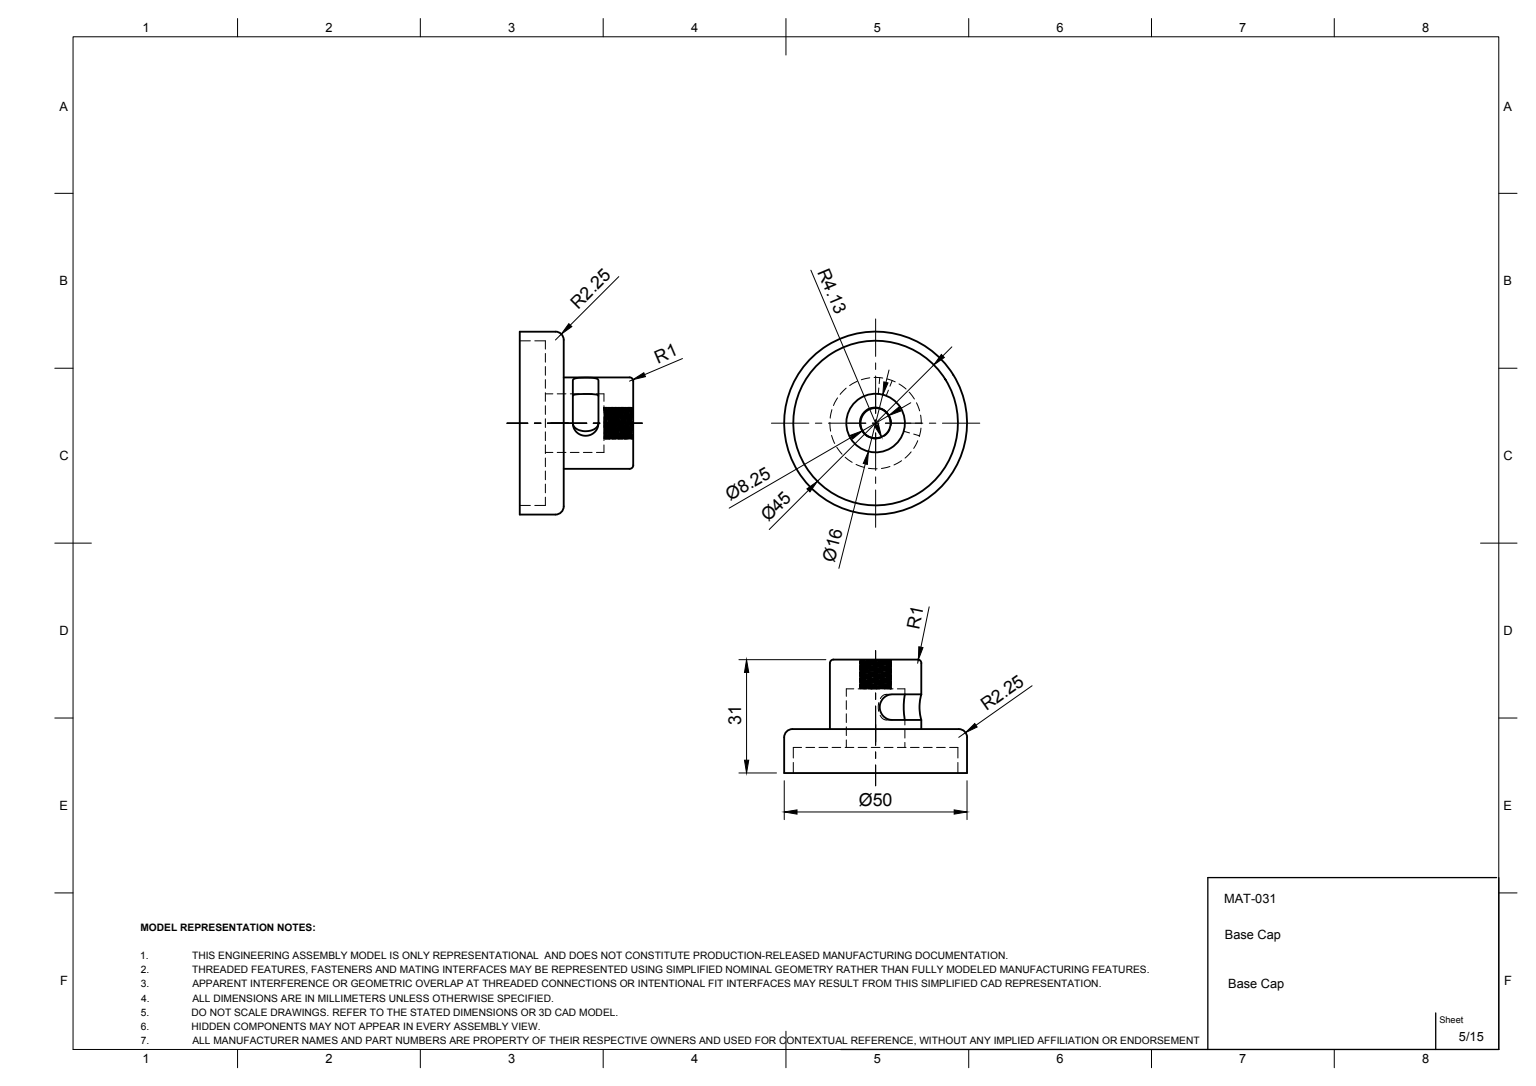
ISO-10303-21;
HEADER;
/* Generated by software containing ST-Developer
 * from STEP Tools, Inc. (www.steptools.com) 
 */

FILE_DESCRIPTION(
/* description */ ('STEP AP214'),
/* implementation_level */ '2;1');

FILE_NAME(
/* name */ 'Base Cap.step',
/* time_stamp */ '2026-11-14T06:58:01-08:00',
/* author */ (''),
/* organization */ (''),
/* preprocessor_version */ 'ST-DEVELOPER v20.2',
/* originating_system */ 'Autodesk Translation Framework v15.17.0.0',
/* authorisation */ '');

FILE_SCHEMA (('AUTOMOTIVE_DESIGN { 1 0 10303 214 3 1 1 }'));
ENDSEC;

DATA;
#10=MECHANICAL_DESIGN_GEOMETRIC_PRESENTATION_REPRESENTATION('',(#1148),#38635);
#124=(
BOUNDED_SURFACE()
B_SPLINE_SURFACE(1,2,((#28370,#28371,#28372,#28373,#28374,#28375,#28376,
#28377,#28378,#28379,#28380,#28381,#28382,#28383,#28384,#28385,#28386,#28387,
#28388,#28389,#28390,#28391,#28392,#28393,#28394,#28395,#28396,#28397,#28398,
#28399,#28400,#28401,#28402,#28403,#28404,#28405,#28406,#28407,#28408,#28409,
#28410,#28411,#28412,#28413,#28414,#28415,#28416,#28417,#28418,#28419,#28420,
#28421,#28422,#28423,#28424,#28425,#28426,#28427,#28428,#28429,#28430,#28431,
#28432,#28433,#28434,#28435,#28436,#28437,#28438,#28439,#28440,#28441,#28442,
#28443,#28444,#28445,#28446,#28447,#28448,#28449,#28450,#28451,#28452,#28453,
#28454,#28455,#28456,#28457,#28458,#28459,#28460,#28461,#28462,#28463,#28464,
#28465,#28466,#28467,#28468,#28469,#28470,#28471,#28472,#28473,#28474,#28475,
#28476,#28477,#28478,#28479,#28480,#28481,#28482,#28483,#28484,#28485,#28486,
#28487,#28488,#28489,#28490,#28491,#28492,#28493,#28494,#28495,#28496,#28497,
#28498,#28499,#28500,#28501,#28502,#28503,#28504,#28505,#28506,#28507,#28508,
#28509,#28510,#28511,#28512,#28513,#28514,#28515,#28516,#28517,#28518,#28519,
#28520,#28521,#28522,#28523,#28524,#28525,#28526,#28527,#28528,#28529,#28530,
#28531,#28532,#28533,#28534,#28535,#28536,#28537,#28538,#28539,#28540,#28541,
#28542,#28543,#28544,#28545,#28546,#28547,#28548,#28549,#28550,#28551,#28552,
#28553,#28554,#28555,#28556,#28557,#28558,#28559,#28560,#28561,#28562,#28563,
#28564,#28565,#28566,#28567,#28568,#28569,#28570,#28571,#28572,#28573,#28574,
#28575,#28576,#28577,#28578,#28579,#28580,#28581,#28582,#28583,#28584,#28585,
#28586,#28587,#28588,#28589,#28590,#28591,#28592,#28593,#28594,#28595,#28596,
#28597,#28598,#28599,#28600,#28601,#28602,#28603,#28604,#28605,#28606,#28607,
#28608,#28609,#28610,#28611,#28612,#28613,#28614,#28615,#28616,#28617,#28618,
#28619,#28620,#28621,#28622,#28623,#28624,#28625,#28626,#28627,#28628,#28629,
#28630,#28631,#28632,#28633,#28634,#28635,#28636,#28637,#28638,#28639,#28640,
#28641,#28642,#28643,#28644,#28645,#28646,#28647,#28648,#28649,#28650,#28651,
#28652,#28653,#28654,#28655,#28656,#28657,#28658,#28659,#28660,#28661,#28662,
#28663,#28664,#28665,#28666,#28667,#28668,#28669,#28670,#28671,#28672,#28673,
#28674,#28675,#28676,#28677,#28678,#28679,#28680,#28681,#28682,#28683,#28684,
#28685,#28686,#28687,#28688,#28689,#28690,#28691,#28692,#28693,#28694,#28695,
#28696,#28697,#28698,#28699,#28700,#28701,#28702,#28703,#28704,#28705,#28706,
#28707,#28708,#28709,#28710,#28711,#28712,#28713,#28714,#28715,#28716,#28717,
#28718,#28719,#28720,#28721,#28722,#28723,#28724,#28725,#28726,#28727,#28728,
#28729,#28730,#28731,#28732,#28733,#28734,#28735,#28736,#28737,#28738,#28739,
#28740,#28741,#28742,#28743,#28744,#28745,#28746,#28747,#28748),(#28749,
#28750,#28751,#28752,#28753,#28754,#28755,#28756,#28757,#28758,#28759,#28760,
#28761,#28762,#28763,#28764,#28765,#28766,#28767,#28768,#28769,#28770,#28771,
#28772,#28773,#28774,#28775,#28776,#28777,#28778,#28779,#28780,#28781,#28782,
#28783,#28784,#28785,#28786,#28787,#28788,#28789,#28790,#28791,#28792,#28793,
#28794,#28795,#28796,#28797,#28798,#28799,#28800,#28801,#28802,#28803,#28804,
#28805,#28806,#28807,#28808,#28809,#28810,#28811,#28812,#28813,#28814,#28815,
#28816,#28817,#28818,#28819,#28820,#28821,#28822,#28823,#28824,#28825,#28826,
#28827,#28828,#28829,#28830,#28831,#28832,#28833,#28834,#28835,#28836,#28837,
#28838,#28839,#28840,#28841,#28842,#28843,#28844,#28845,#28846,#28847,#28848,
#28849,#28850,#28851,#28852,#28853,#28854,#28855,#28856,#28857,#28858,#28859,
#28860,#28861,#28862,#28863,#28864,#28865,#28866,#28867,#28868,#28869,#28870,
#28871,#28872,#28873,#28874,#28875,#28876,#28877,#28878,#28879,#28880,#28881,
#28882,#28883,#28884,#28885,#28886,#28887,#28888,#28889,#28890,#28891,#28892,
#28893,#28894,#28895,#28896,#28897,#28898,#28899,#28900,#28901,#28902,#28903,
#28904,#28905,#28906,#28907,#28908,#28909,#28910,#28911,#28912,#28913,#28914,
#28915,#28916,#28917,#28918,#28919,#28920,#28921,#28922,#28923,#28924,#28925,
#28926,#28927,#28928,#28929,#28930,#28931,#28932,#28933,#28934,#28935,#28936,
#28937,#28938,#28939,#28940,#28941,#28942,#28943,#28944,#28945,#28946,#28947,
#28948,#28949,#28950,#28951,#28952,#28953,#28954,#28955,#28956,#28957,#28958,
#28959,#28960,#28961,#28962,#28963,#28964,#28965,#28966,#28967,#28968,#28969,
#28970,#28971,#28972,#28973,#28974,#28975,#28976,#28977,#28978,#28979,#28980,
#28981,#28982,#28983,#28984,#28985,#28986,#28987,#28988,#28989,#28990,#28991,
#28992,#28993,#28994,#28995,#28996,#28997,#28998,#28999,#29000,#29001,#29002,
#29003,#29004,#29005,#29006,#29007,#29008,#29009,#29010,#29011,#29012,#29013,
#29014,#29015,#29016,#29017,#29018,#29019,#29020,#29021,#29022,#29023,#29024,
#29025,#29026,#29027,#29028,#29029,#29030,#29031,#29032,#29033,#29034,#29035,
#29036,#29037,#29038,#29039,#29040,#29041,#29042,#29043,#29044,#29045,#29046,
#29047,#29048,#29049,#29050,#29051,#29052,#29053,#29054,#29055,#29056,#29057,
#29058,#29059,#29060,#29061,#29062,#29063,#29064,#29065,#29066,#29067,#29068,
#29069,#29070,#29071,#29072,#29073,#29074,#29075,#29076,#29077,#29078,#29079,
#29080,#29081,#29082,#29083,#29084,#29085,#29086,#29087,#29088,#29089,#29090,
#29091,#29092,#29093,#29094,#29095,#29096,#29097,#29098,#29099,#29100,#29101,
#29102,#29103,#29104,#29105,#29106,#29107,#29108,#29109,#29110,#29111,#29112,
#29113,#29114,#29115,#29116,#29117,#29118,#29119,#29120,#29121,#29122,#29123,
#29124,#29125,#29126,#29127)),.UNSPECIFIED.,.F.,.F.,.F.)
B_SPLINE_SURFACE_WITH_KNOTS((2,2),(3,2,2,2,2,2,2,2,2,2,2,2,2,2,2,2,2,2,
2,2,2,2,2,2,2,2,2,2,2,2,2,2,2,2,2,2,2,2,2,2,2,2,2,2,2,2,2,2,2,2,2,2,2,2,
2,2,2,2,2,2,2,2,2,2,2,2,2,2,2,2,2,2,2,2,2,2,2,2,2,2,2,2,2,2,2,2,2,2,2,2,
2,2,2,2,2,2,2,2,2,2,2,2,2,2,2,2,2,2,2,2,2,2,2,2,2,2,2,2,2,2,2,2,2,2,2,2,
2,2,2,2,2,2,2,2,2,2,2,2,2,2,2,2,2,2,2,2,2,2,2,2,2,2,2,2,2,2,2,2,2,2,2,2,
2,2,2,2,2,2,2,2,2,2,2,2,2,2,2,2,2,2,2,2,2,2,2,2,2,2,2,3),(0.,1.),(0.,0.00520833333333333,
0.0104166666666667,0.015625,0.0208333333333333,0.0260416666666667,0.03125,
0.0364583333333333,0.0416666666666667,0.046875,0.0520833333333333,0.0572916666666667,
0.0625,0.0677083333333333,0.0729166666666667,0.078125,0.0833333333333333,
0.0885416666666667,0.09375,0.0989583333333333,0.104166666666667,0.109375,
0.114583333333333,0.119791666666667,0.125,0.130208333333333,0.135416666666667,
0.140625,0.145833333333333,0.151041666666667,0.15625,0.161458333333333,
0.166666666666667,0.171875,0.177083333333333,0.182291666666667,0.1875,0.192708333333333,
0.197916666666667,0.203125,0.208333333333333,0.213541666666667,0.21875,
0.223958333333333,0.229166666666667,0.234375,0.239583333333333,0.244791666666667,
0.25,0.255208333333333,0.260416666666667,0.265625,0.270833333333333,0.276041666666667,
0.28125,0.286458333333333,0.291666666666667,0.296875,0.302083333333333,
0.307291666666667,0.3125,0.317708333333333,0.322916666666667,0.328125,0.333333333333333,
0.338541666666667,0.34375,0.348958333333333,0.354166666666667,0.359375,
0.364583333333333,0.369791666666667,0.375,0.380208333333333,0.385416666666667,
0.390625,0.395833333333333,0.401041666666667,0.40625,0.411458333333333,
0.416666666666667,0.421875,0.427083333333333,0.432291666666667,0.4375,0.442708333333333,
0.447916666666667,0.453125,0.458333333333333,0.463541666666667,0.46875,
0.473958333333333,0.479166666666667,0.484375,0.489583333333333,0.494791666666667,
0.5,0.505208333333333,0.510416666666667,0.515625,0.520833333333333,0.526041666666667,
0.53125,0.536458333333333,0.541666666666667,0.546875,0.552083333333333,
0.557291666666667,0.5625,0.567708333333333,0.572916666666667,0.578125,0.583333333333333,
0.588541666666667,0.59375,0.598958333333333,0.604166666666667,0.609375,
0.614583333333333,0.619791666666667,0.625,0.630208333333333,0.635416666666667,
0.640625,0.645833333333333,0.651041666666667,0.65625,0.661458333333333,
0.666666666666667,0.671875,0.677083333333333,0.682291666666667,0.6875,0.692708333333333,
0.697916666666667,0.703125,0.708333333333333,0.713541666666667,0.71875,
0.723958333333333,0.729166666666667,0.734375,0.739583333333333,0.744791666666667,
0.75,0.755208333333333,0.760416666666667,0.765625,0.770833333333333,0.776041666666667,
0.78125,0.786458333333333,0.791666666666667,0.796875,0.802083333333333,
0.807291666666667,0.8125,0.817708333333333,0.822916666666667,0.828125,0.833333333333333,
0.838541666666667,0.84375,0.848958333333333,0.854166666666667,0.859375,
0.864583333333333,0.869791666666667,0.875,0.880208333333333,0.885416666666667,
0.890625,0.895833333333333,0.901041666666667,0.90625,0.911458333333333,
0.916666666666667,0.921875,0.927083333333333,0.932291666666667,0.9375,0.942708333333333,
0.947916666666667,0.953125,0.958333333333333,0.963541666666667,0.96875,
0.973958333333333,0.979166666666667,0.984246579235552),.UNSPECIFIED.)
GEOMETRIC_REPRESENTATION_ITEM()
RATIONAL_B_SPLINE_SURFACE(((1.,0.866025403784439,1.,0.866025403784439,1.,
0.866025403784439,1.,0.866025403784439,1.,0.866025403784439,1.,0.866025403784439,
1.,0.866025403784439,1.,0.866025403784439,1.,0.866025403784439,1.,0.866025403784439,
1.,0.866025403784439,1.,0.866025403784439,1.,0.866025403784439,1.,0.866025403784439,
1.,0.866025403784439,1.,0.866025403784439,1.,0.866025403784439,1.,0.866025403784439,
1.,0.866025403784439,1.,0.866025403784439,1.,0.866025403784439,1.,0.866025403784439,
1.,0.866025403784439,1.,0.866025403784439,1.,0.866025403784439,1.,0.866025403784439,
1.,0.866025403784439,1.,0.866025403784439,1.,0.866025403784439,1.,0.866025403784439,
1.,0.866025403784439,1.,0.866025403784439,1.,0.866025403784439,1.,0.866025403784439,
1.,0.866025403784439,1.,0.866025403784439,1.,0.866025403784439,1.,0.866025403784439,
1.,0.866025403784439,1.,0.866025403784439,1.,0.866025403784439,1.,0.866025403784439,
1.,0.866025403784439,1.,0.866025403784439,1.,0.866025403784439,1.,0.866025403784439,
1.,0.866025403784439,1.,0.866025403784439,1.,0.866025403784439,1.,0.866025403784439,
1.,0.866025403784439,1.,0.866025403784439,1.,0.866025403784439,1.,0.866025403784439,
1.,0.866025403784439,1.,0.866025403784439,1.,0.866025403784439,1.,0.866025403784439,
1.,0.866025403784439,1.,0.866025403784439,1.,0.866025403784439,1.,0.866025403784439,
1.,0.866025403784439,1.,0.866025403784439,1.,0.866025403784439,1.,0.866025403784439,
1.,0.866025403784439,1.,0.866025403784439,1.,0.866025403784439,1.,0.866025403784439,
1.,0.866025403784439,1.,0.866025403784439,1.,0.866025403784439,1.,0.866025403784439,
1.,0.866025403784439,1.,0.866025403784439,1.,0.866025403784439,1.,0.866025403784439,
1.,0.866025403784439,1.,0.866025403784439,1.,0.866025403784439,1.,0.866025403784439,
1.,0.866025403784439,1.,0.866025403784439,1.,0.866025403784439,1.,0.866025403784439,
1.,0.866025403784439,1.,0.866025403784439,1.,0.866025403784439,1.,0.866025403784439,
1.,0.866025403784439,1.,0.866025403784439,1.,0.866025403784439,1.,0.866025403784439,
1.,0.866025403784439,1.,0.866025403784439,1.,0.866025403784439,1.,0.866025403784439,
1.,0.866025403784439,1.,0.866025403784439,1.,0.866025403784439,1.,0.866025403784439,
1.,0.866025403784439,1.,0.866025403784439,1.,0.866025403784439,1.,0.866025403784439,
1.,0.866025403784439,1.,0.866025403784439,1.,0.866025403784439,1.,0.866025403784439,
1.,0.866025403784439,1.,0.866025403784439,1.,0.866025403784439,1.,0.866025403784439,
1.,0.866025403784439,1.,0.866025403784439,1.,0.866025403784439,1.,0.866025403784439,
1.,0.866025403784439,1.,0.866025403784439,1.,0.866025403784439,1.,0.866025403784439,
1.,0.866025403784439,1.,0.866025403784439,1.,0.866025403784439,1.,0.866025403784439,
1.,0.866025403784439,1.,0.866025403784439,1.,0.866025403784439,1.,0.866025403784439,
1.,0.866025403784439,1.,0.866025403784439,1.,0.866025403784439,1.,0.866025403784439,
1.,0.866025403784439,1.,0.866025403784439,1.,0.866025403784439,1.,0.866025403784439,
1.,0.866025403784439,1.,0.866025403784439,1.,0.866025403784439,1.,0.866025403784439,
1.,0.866025403784439,1.,0.866025403784439,1.,0.866025403784439,1.,0.866025403784439,
1.,0.866025403784439,1.,0.866025403784439,1.,0.866025403784439,1.,0.866025403784439,
1.,0.866025403784439,1.,0.866025403784439,1.,0.866025403784439,1.,0.866025403784439,
1.,0.866025403784439,1.,0.866025403784439,1.,0.866025403784439,1.,0.866025403784439,
1.,0.866025403784439,1.,0.866025403784439,1.,0.866025403784439,1.,0.866025403784439,
1.,0.866025403784439,1.,0.866025403784439,1.,0.866025403784439,1.,0.866025403784439,
1.,0.866025403784439,1.,0.866025403784439,1.,0.866025403784439,1.,0.866025403784439,
1.,0.866025403784439,1.,0.866025403784439,1.,0.866025403784439,1.,0.866025403784439,
1.,0.866025403784439,1.,0.866025403784439,1.,0.866025403784439,1.,0.866025403784439,
1.,0.866025403784439,1.,0.866025403784439,1.,0.866025403784439,1.,0.866025403784439,
1.,0.866025403784439,1.,0.866025403784439,1.,0.866025403784439,1.,0.866025403784439,
1.,0.866025403784439,1.,0.866025403784439,1.,0.869328786836457,0.993556135519056),
(1.,0.866025403784439,1.,0.866025403784439,1.,0.866025403784439,1.,0.866025403784439,
1.,0.866025403784439,1.,0.866025403784439,1.,0.866025403784439,1.,0.866025403784439,
1.,0.866025403784439,1.,0.866025403784439,1.,0.866025403784439,1.,0.866025403784439,
1.,0.866025403784439,1.,0.866025403784439,1.,0.866025403784439,1.,0.866025403784439,
1.,0.866025403784439,1.,0.866025403784439,1.,0.866025403784439,1.,0.866025403784439,
1.,0.866025403784439,1.,0.866025403784439,1.,0.866025403784439,1.,0.866025403784439,
1.,0.866025403784439,1.,0.866025403784439,1.,0.866025403784439,1.,0.866025403784439,
1.,0.866025403784439,1.,0.866025403784439,1.,0.866025403784439,1.,0.866025403784439,
1.,0.866025403784439,1.,0.866025403784439,1.,0.866025403784439,1.,0.866025403784439,
1.,0.866025403784439,1.,0.866025403784439,1.,0.866025403784439,1.,0.866025403784439,
1.,0.866025403784439,1.,0.866025403784439,1.,0.866025403784439,1.,0.866025403784439,
1.,0.866025403784439,1.,0.866025403784439,1.,0.866025403784439,1.,0.866025403784439,
1.,0.866025403784439,1.,0.866025403784439,1.,0.866025403784439,1.,0.866025403784439,
1.,0.866025403784439,1.,0.866025403784439,1.,0.866025403784439,1.,0.866025403784439,
1.,0.866025403784439,1.,0.866025403784439,1.,0.866025403784439,1.,0.866025403784439,
1.,0.866025403784439,1.,0.866025403784439,1.,0.866025403784439,1.,0.866025403784439,
1.,0.866025403784439,1.,0.866025403784439,1.,0.866025403784439,1.,0.866025403784439,
1.,0.866025403784439,1.,0.866025403784439,1.,0.866025403784439,1.,0.866025403784439,
1.,0.866025403784439,1.,0.866025403784439,1.,0.866025403784439,1.,0.866025403784439,
1.,0.866025403784439,1.,0.866025403784439,1.,0.866025403784439,1.,0.866025403784439,
1.,0.866025403784439,1.,0.866025403784439,1.,0.866025403784439,1.,0.866025403784439,
1.,0.866025403784439,1.,0.866025403784439,1.,0.866025403784439,1.,0.866025403784439,
1.,0.866025403784439,1.,0.866025403784439,1.,0.866025403784439,1.,0.866025403784439,
1.,0.866025403784439,1.,0.866025403784439,1.,0.866025403784439,1.,0.866025403784439,
1.,0.866025403784439,1.,0.866025403784439,1.,0.866025403784439,1.,0.866025403784439,
1.,0.866025403784439,1.,0.866025403784439,1.,0.866025403784439,1.,0.866025403784439,
1.,0.866025403784439,1.,0.866025403784439,1.,0.866025403784439,1.,0.866025403784439,
1.,0.866025403784439,1.,0.866025403784439,1.,0.866025403784439,1.,0.866025403784439,
1.,0.866025403784439,1.,0.866025403784439,1.,0.866025403784439,1.,0.866025403784439,
1.,0.866025403784439,1.,0.866025403784439,1.,0.866025403784439,1.,0.866025403784439,
1.,0.866025403784439,1.,0.866025403784439,1.,0.866025403784439,1.,0.866025403784439,
1.,0.866025403784439,1.,0.866025403784439,1.,0.866025403784439,1.,0.866025403784439,
1.,0.866025403784439,1.,0.866025403784439,1.,0.866025403784439,1.,0.866025403784439,
1.,0.866025403784439,1.,0.866025403784439,1.,0.866025403784439,1.,0.866025403784439,
1.,0.866025403784439,1.,0.866025403784439,1.,0.866025403784439,1.,0.866025403784439,
1.,0.866025403784439,1.,0.866025403784439,1.,0.866025403784439,1.,0.866025403784439,
1.,0.866025403784439,1.,0.866025403784439,1.,0.866025403784439,1.,0.866025403784439,
1.,0.866025403784439,1.,0.866025403784439,1.,0.866025403784439,1.,0.866025403784439,
1.,0.866025403784439,1.,0.866025403784439,1.,0.866025403784439,1.,0.866025403784439,
1.,0.866025403784439,1.,0.866025403784439,1.,0.866025403784439,1.,0.866025403784439,
1.,0.866025403784439,1.,0.866025403784439,1.,0.866025403784439,1.,0.866025403784439,
1.,0.866025403784439,1.,0.866025403784439,1.,0.866025403784439,1.,0.866025403784439,
1.,0.866025403784439,1.,0.866025403784439,1.,0.866025403784439,1.,0.866025403784439,
1.,0.866025403784439,1.,0.866025403784439,1.,0.866025403784439,1.,0.866025403784439,
1.,0.866025403784439,1.,0.866025403784439,1.,0.866025403784439,1.,0.866025403784439,
1.,0.866025403784439,1.,0.866025403784439,1.,0.866025403784439,1.,0.866025403784439,
1.,0.866025403784439,1.,0.866025403784439,1.,0.866025403784439,1.,0.866025403784439,
1.,0.869328786836457,0.993556135519056)))
REPRESENTATION_ITEM('')
SURFACE()
);
#125=(
BOUNDED_SURFACE()
B_SPLINE_SURFACE(1,2,((#29128,#29129,#29130,#29131,#29132,#29133,#29134,
#29135,#29136,#29137,#29138,#29139,#29140,#29141,#29142,#29143,#29144,#29145,
#29146,#29147,#29148,#29149,#29150,#29151,#29152,#29153,#29154,#29155,#29156,
#29157,#29158,#29159,#29160,#29161,#29162,#29163,#29164,#29165,#29166,#29167,
#29168,#29169,#29170,#29171,#29172,#29173,#29174,#29175,#29176,#29177,#29178,
#29179,#29180,#29181,#29182,#29183,#29184,#29185,#29186,#29187,#29188,#29189,
#29190,#29191,#29192,#29193,#29194,#29195,#29196,#29197,#29198,#29199,#29200,
#29201,#29202,#29203,#29204,#29205,#29206,#29207,#29208,#29209,#29210,#29211,
#29212,#29213,#29214,#29215,#29216,#29217,#29218,#29219,#29220,#29221,#29222,
#29223,#29224,#29225,#29226,#29227,#29228,#29229,#29230,#29231,#29232,#29233,
#29234,#29235,#29236,#29237,#29238,#29239,#29240,#29241,#29242,#29243,#29244,
#29245,#29246,#29247,#29248,#29249,#29250,#29251,#29252,#29253,#29254,#29255,
#29256,#29257,#29258,#29259,#29260,#29261,#29262,#29263,#29264,#29265,#29266,
#29267,#29268,#29269,#29270,#29271,#29272,#29273,#29274,#29275,#29276,#29277,
#29278,#29279,#29280,#29281,#29282,#29283,#29284,#29285,#29286,#29287,#29288,
#29289,#29290,#29291,#29292,#29293,#29294,#29295,#29296,#29297,#29298,#29299,
#29300,#29301,#29302,#29303,#29304,#29305,#29306,#29307,#29308,#29309,#29310,
#29311,#29312,#29313,#29314,#29315,#29316,#29317,#29318,#29319,#29320,#29321,
#29322,#29323,#29324,#29325,#29326,#29327,#29328,#29329,#29330,#29331,#29332,
#29333,#29334,#29335,#29336,#29337,#29338,#29339,#29340,#29341,#29342,#29343,
#29344,#29345,#29346,#29347,#29348,#29349,#29350,#29351,#29352,#29353,#29354,
#29355,#29356,#29357,#29358,#29359,#29360,#29361,#29362,#29363,#29364,#29365,
#29366,#29367,#29368,#29369,#29370,#29371,#29372,#29373,#29374,#29375,#29376,
#29377,#29378,#29379,#29380,#29381,#29382,#29383,#29384,#29385,#29386,#29387,
#29388,#29389,#29390,#29391,#29392,#29393,#29394,#29395,#29396,#29397,#29398,
#29399,#29400,#29401,#29402,#29403,#29404,#29405,#29406,#29407,#29408,#29409,
#29410,#29411,#29412,#29413,#29414,#29415,#29416,#29417,#29418,#29419,#29420,
#29421,#29422,#29423,#29424,#29425,#29426,#29427,#29428,#29429,#29430,#29431,
#29432,#29433,#29434,#29435,#29436,#29437,#29438,#29439,#29440,#29441,#29442,
#29443,#29444,#29445,#29446,#29447,#29448,#29449,#29450,#29451,#29452,#29453,
#29454,#29455,#29456,#29457,#29458,#29459,#29460,#29461,#29462,#29463,#29464,
#29465,#29466,#29467,#29468,#29469,#29470,#29471,#29472,#29473,#29474,#29475,
#29476,#29477,#29478,#29479,#29480,#29481,#29482,#29483,#29484,#29485,#29486,
#29487,#29488,#29489,#29490,#29491,#29492,#29493,#29494,#29495,#29496,#29497,
#29498,#29499,#29500,#29501,#29502,#29503,#29504,#29505,#29506),(#29507,
#29508,#29509,#29510,#29511,#29512,#29513,#29514,#29515,#29516,#29517,#29518,
#29519,#29520,#29521,#29522,#29523,#29524,#29525,#29526,#29527,#29528,#29529,
#29530,#29531,#29532,#29533,#29534,#29535,#29536,#29537,#29538,#29539,#29540,
#29541,#29542,#29543,#29544,#29545,#29546,#29547,#29548,#29549,#29550,#29551,
#29552,#29553,#29554,#29555,#29556,#29557,#29558,#29559,#29560,#29561,#29562,
#29563,#29564,#29565,#29566,#29567,#29568,#29569,#29570,#29571,#29572,#29573,
#29574,#29575,#29576,#29577,#29578,#29579,#29580,#29581,#29582,#29583,#29584,
#29585,#29586,#29587,#29588,#29589,#29590,#29591,#29592,#29593,#29594,#29595,
#29596,#29597,#29598,#29599,#29600,#29601,#29602,#29603,#29604,#29605,#29606,
#29607,#29608,#29609,#29610,#29611,#29612,#29613,#29614,#29615,#29616,#29617,
#29618,#29619,#29620,#29621,#29622,#29623,#29624,#29625,#29626,#29627,#29628,
#29629,#29630,#29631,#29632,#29633,#29634,#29635,#29636,#29637,#29638,#29639,
#29640,#29641,#29642,#29643,#29644,#29645,#29646,#29647,#29648,#29649,#29650,
#29651,#29652,#29653,#29654,#29655,#29656,#29657,#29658,#29659,#29660,#29661,
#29662,#29663,#29664,#29665,#29666,#29667,#29668,#29669,#29670,#29671,#29672,
#29673,#29674,#29675,#29676,#29677,#29678,#29679,#29680,#29681,#29682,#29683,
#29684,#29685,#29686,#29687,#29688,#29689,#29690,#29691,#29692,#29693,#29694,
#29695,#29696,#29697,#29698,#29699,#29700,#29701,#29702,#29703,#29704,#29705,
#29706,#29707,#29708,#29709,#29710,#29711,#29712,#29713,#29714,#29715,#29716,
#29717,#29718,#29719,#29720,#29721,#29722,#29723,#29724,#29725,#29726,#29727,
#29728,#29729,#29730,#29731,#29732,#29733,#29734,#29735,#29736,#29737,#29738,
#29739,#29740,#29741,#29742,#29743,#29744,#29745,#29746,#29747,#29748,#29749,
#29750,#29751,#29752,#29753,#29754,#29755,#29756,#29757,#29758,#29759,#29760,
#29761,#29762,#29763,#29764,#29765,#29766,#29767,#29768,#29769,#29770,#29771,
#29772,#29773,#29774,#29775,#29776,#29777,#29778,#29779,#29780,#29781,#29782,
#29783,#29784,#29785,#29786,#29787,#29788,#29789,#29790,#29791,#29792,#29793,
#29794,#29795,#29796,#29797,#29798,#29799,#29800,#29801,#29802,#29803,#29804,
#29805,#29806,#29807,#29808,#29809,#29810,#29811,#29812,#29813,#29814,#29815,
#29816,#29817,#29818,#29819,#29820,#29821,#29822,#29823,#29824,#29825,#29826,
#29827,#29828,#29829,#29830,#29831,#29832,#29833,#29834,#29835,#29836,#29837,
#29838,#29839,#29840,#29841,#29842,#29843,#29844,#29845,#29846,#29847,#29848,
#29849,#29850,#29851,#29852,#29853,#29854,#29855,#29856,#29857,#29858,#29859,
#29860,#29861,#29862,#29863,#29864,#29865,#29866,#29867,#29868,#29869,#29870,
#29871,#29872,#29873,#29874,#29875,#29876,#29877,#29878,#29879,#29880,#29881,
#29882,#29883,#29884,#29885)),.UNSPECIFIED.,.F.,.F.,.F.)
B_SPLINE_SURFACE_WITH_KNOTS((2,2),(3,2,2,2,2,2,2,2,2,2,2,2,2,2,2,2,2,2,
2,2,2,2,2,2,2,2,2,2,2,2,2,2,2,2,2,2,2,2,2,2,2,2,2,2,2,2,2,2,2,2,2,2,2,2,
2,2,2,2,2,2,2,2,2,2,2,2,2,2,2,2,2,2,2,2,2,2,2,2,2,2,2,2,2,2,2,2,2,2,2,2,
2,2,2,2,2,2,2,2,2,2,2,2,2,2,2,2,2,2,2,2,2,2,2,2,2,2,2,2,2,2,2,2,2,2,2,2,
2,2,2,2,2,2,2,2,2,2,2,2,2,2,2,2,2,2,2,2,2,2,2,2,2,2,2,2,2,2,2,2,2,2,2,2,
2,2,2,2,2,2,2,2,2,2,2,2,2,2,2,2,2,2,2,2,2,2,2,2,2,2,2,3),(0.,1.),(0.,0.00520833333333333,
0.0104166666666667,0.015625,0.0208333333333333,0.0260416666666667,0.03125,
0.0364583333333333,0.0416666666666667,0.046875,0.0520833333333333,0.0572916666666667,
0.0625,0.0677083333333333,0.0729166666666667,0.078125,0.0833333333333333,
0.0885416666666667,0.09375,0.0989583333333333,0.104166666666667,0.109375,
0.114583333333333,0.119791666666667,0.125,0.130208333333333,0.135416666666667,
0.140625,0.145833333333333,0.151041666666667,0.15625,0.161458333333333,
0.166666666666667,0.171875,0.177083333333333,0.182291666666667,0.1875,0.192708333333333,
0.197916666666667,0.203125,0.208333333333333,0.213541666666667,0.21875,
0.223958333333333,0.229166666666667,0.234375,0.239583333333333,0.244791666666667,
0.25,0.255208333333333,0.260416666666667,0.265625,0.270833333333333,0.276041666666667,
0.28125,0.286458333333333,0.291666666666667,0.296875,0.302083333333333,
0.307291666666667,0.3125,0.317708333333333,0.322916666666667,0.328125,0.333333333333333,
0.338541666666667,0.34375,0.348958333333333,0.354166666666667,0.359375,
0.364583333333333,0.369791666666667,0.375,0.380208333333333,0.385416666666667,
0.390625,0.395833333333333,0.401041666666667,0.40625,0.411458333333333,
0.416666666666667,0.421875,0.427083333333333,0.432291666666667,0.4375,0.442708333333333,
0.447916666666667,0.453125,0.458333333333333,0.463541666666667,0.46875,
0.473958333333333,0.479166666666667,0.484375,0.489583333333333,0.494791666666667,
0.5,0.505208333333333,0.510416666666667,0.515625,0.520833333333333,0.526041666666667,
0.53125,0.536458333333333,0.541666666666667,0.546875,0.552083333333333,
0.557291666666667,0.5625,0.567708333333333,0.572916666666667,0.578125,0.583333333333333,
0.588541666666667,0.59375,0.598958333333333,0.604166666666667,0.609375,
0.614583333333333,0.619791666666667,0.625,0.630208333333333,0.635416666666667,
0.640625,0.645833333333333,0.651041666666667,0.65625,0.661458333333333,
0.666666666666667,0.671875,0.677083333333333,0.682291666666667,0.6875,0.692708333333333,
0.697916666666667,0.703125,0.708333333333333,0.713541666666667,0.71875,
0.723958333333333,0.729166666666667,0.734375,0.739583333333333,0.744791666666667,
0.75,0.755208333333333,0.760416666666667,0.765625,0.770833333333333,0.776041666666667,
0.78125,0.786458333333333,0.791666666666667,0.796875,0.802083333333333,
0.807291666666667,0.8125,0.817708333333333,0.822916666666667,0.828125,0.833333333333333,
0.838541666666667,0.84375,0.848958333333333,0.854166666666667,0.859375,
0.864583333333333,0.869791666666667,0.875,0.880208333333333,0.885416666666667,
0.890625,0.895833333333333,0.901041666666667,0.90625,0.911458333333333,
0.916666666666667,0.921875,0.927083333333333,0.932291666666667,0.9375,0.942708333333333,
0.947916666666667,0.953125,0.958333333333333,0.963541666666667,0.96875,
0.973958333333333,0.979166666666667,0.984246579355594),.UNSPECIFIED.)
GEOMETRIC_REPRESENTATION_ITEM()
RATIONAL_B_SPLINE_SURFACE(((1.,0.866025403784439,1.,0.866025403784439,1.,
0.866025403784439,1.,0.866025403784439,1.,0.866025403784439,1.,0.866025403784439,
1.,0.866025403784439,1.,0.866025403784439,1.,0.866025403784439,1.,0.866025403784439,
1.,0.866025403784439,1.,0.866025403784439,1.,0.866025403784439,1.,0.866025403784439,
1.,0.866025403784439,1.,0.866025403784439,1.,0.866025403784439,1.,0.866025403784439,
1.,0.866025403784439,1.,0.866025403784439,1.,0.866025403784439,1.,0.866025403784439,
1.,0.866025403784439,1.,0.866025403784439,1.,0.866025403784439,1.,0.866025403784439,
1.,0.866025403784439,1.,0.866025403784439,1.,0.866025403784439,1.,0.866025403784439,
1.,0.866025403784439,1.,0.866025403784439,1.,0.866025403784439,1.,0.866025403784439,
1.,0.866025403784439,1.,0.866025403784439,1.,0.866025403784439,1.,0.866025403784439,
1.,0.866025403784439,1.,0.866025403784439,1.,0.866025403784439,1.,0.866025403784439,
1.,0.866025403784439,1.,0.866025403784439,1.,0.866025403784439,1.,0.866025403784439,
1.,0.866025403784439,1.,0.866025403784439,1.,0.866025403784439,1.,0.866025403784439,
1.,0.866025403784439,1.,0.866025403784439,1.,0.866025403784439,1.,0.866025403784439,
1.,0.866025403784439,1.,0.866025403784439,1.,0.866025403784439,1.,0.866025403784439,
1.,0.866025403784439,1.,0.866025403784439,1.,0.866025403784439,1.,0.866025403784439,
1.,0.866025403784439,1.,0.866025403784439,1.,0.866025403784439,1.,0.866025403784439,
1.,0.866025403784439,1.,0.866025403784439,1.,0.866025403784439,1.,0.866025403784439,
1.,0.866025403784439,1.,0.866025403784439,1.,0.866025403784439,1.,0.866025403784439,
1.,0.866025403784439,1.,0.866025403784439,1.,0.866025403784439,1.,0.866025403784439,
1.,0.866025403784439,1.,0.866025403784439,1.,0.866025403784439,1.,0.866025403784439,
1.,0.866025403784439,1.,0.866025403784439,1.,0.866025403784439,1.,0.866025403784439,
1.,0.866025403784439,1.,0.866025403784439,1.,0.866025403784439,1.,0.866025403784439,
1.,0.866025403784439,1.,0.866025403784439,1.,0.866025403784439,1.,0.866025403784439,
1.,0.866025403784439,1.,0.866025403784439,1.,0.866025403784439,1.,0.866025403784439,
1.,0.866025403784439,1.,0.866025403784439,1.,0.866025403784439,1.,0.866025403784439,
1.,0.866025403784439,1.,0.866025403784439,1.,0.866025403784439,1.,0.866025403784439,
1.,0.866025403784439,1.,0.866025403784439,1.,0.866025403784439,1.,0.866025403784439,
1.,0.866025403784439,1.,0.866025403784439,1.,0.866025403784439,1.,0.866025403784439,
1.,0.866025403784439,1.,0.866025403784439,1.,0.866025403784439,1.,0.866025403784439,
1.,0.866025403784439,1.,0.866025403784439,1.,0.866025403784439,1.,0.866025403784439,
1.,0.866025403784439,1.,0.866025403784439,1.,0.866025403784439,1.,0.866025403784439,
1.,0.866025403784439,1.,0.866025403784439,1.,0.866025403784439,1.,0.866025403784439,
1.,0.866025403784439,1.,0.866025403784439,1.,0.866025403784439,1.,0.866025403784439,
1.,0.866025403784439,1.,0.866025403784439,1.,0.866025403784439,1.,0.866025403784439,
1.,0.866025403784439,1.,0.866025403784439,1.,0.866025403784439,1.,0.866025403784439,
1.,0.866025403784439,1.,0.866025403784439,1.,0.866025403784439,1.,0.866025403784439,
1.,0.866025403784439,1.,0.866025403784439,1.,0.866025403784439,1.,0.866025403784439,
1.,0.866025403784439,1.,0.866025403784439,1.,0.866025403784439,1.,0.866025403784439,
1.,0.866025403784439,1.,0.866025403784439,1.,0.866025403784439,1.,0.866025403784439,
1.,0.866025403784439,1.,0.866025403784439,1.,0.866025403784439,1.,0.866025403784439,
1.,0.866025403784439,1.,0.866025403784439,1.,0.866025403784439,1.,0.866025403784439,
1.,0.866025403784439,1.,0.866025403784439,1.,0.866025403784439,1.,0.866025403784439,
1.,0.866025403784439,1.,0.866025403784439,1.,0.866025403784439,1.,0.866025403784439,
1.,0.866025403784439,1.,0.866025403784439,1.,0.866025403784439,1.,0.866025403784439,
1.,0.866025403784439,1.,0.866025403784439,1.,0.866025403784439,1.,0.866025403784439,
1.,0.866025403784439,1.,0.866025403784439,1.,0.866025403784439,1.,0.866025403784439,
1.,0.866025403784439,1.,0.866025403784439,1.,0.869328783748594,0.993556141390235),
(1.,0.866025403784439,1.,0.866025403784439,1.,0.866025403784439,1.,0.866025403784439,
1.,0.866025403784439,1.,0.866025403784439,1.,0.866025403784439,1.,0.866025403784439,
1.,0.866025403784439,1.,0.866025403784439,1.,0.866025403784439,1.,0.866025403784439,
1.,0.866025403784439,1.,0.866025403784439,1.,0.866025403784439,1.,0.866025403784439,
1.,0.866025403784439,1.,0.866025403784439,1.,0.866025403784439,1.,0.866025403784439,
1.,0.866025403784439,1.,0.866025403784439,1.,0.866025403784439,1.,0.866025403784439,
1.,0.866025403784439,1.,0.866025403784439,1.,0.866025403784439,1.,0.866025403784439,
1.,0.866025403784439,1.,0.866025403784439,1.,0.866025403784439,1.,0.866025403784439,
1.,0.866025403784439,1.,0.866025403784439,1.,0.866025403784439,1.,0.866025403784439,
1.,0.866025403784439,1.,0.866025403784439,1.,0.866025403784439,1.,0.866025403784439,
1.,0.866025403784439,1.,0.866025403784439,1.,0.866025403784439,1.,0.866025403784439,
1.,0.866025403784439,1.,0.866025403784439,1.,0.866025403784439,1.,0.866025403784439,
1.,0.866025403784439,1.,0.866025403784439,1.,0.866025403784439,1.,0.866025403784439,
1.,0.866025403784439,1.,0.866025403784439,1.,0.866025403784439,1.,0.866025403784439,
1.,0.866025403784439,1.,0.866025403784439,1.,0.866025403784439,1.,0.866025403784439,
1.,0.866025403784439,1.,0.866025403784439,1.,0.866025403784439,1.,0.866025403784439,
1.,0.866025403784439,1.,0.866025403784439,1.,0.866025403784439,1.,0.866025403784439,
1.,0.866025403784439,1.,0.866025403784439,1.,0.866025403784439,1.,0.866025403784439,
1.,0.866025403784439,1.,0.866025403784439,1.,0.866025403784439,1.,0.866025403784439,
1.,0.866025403784439,1.,0.866025403784439,1.,0.866025403784439,1.,0.866025403784439,
1.,0.866025403784439,1.,0.866025403784439,1.,0.866025403784439,1.,0.866025403784439,
1.,0.866025403784439,1.,0.866025403784439,1.,0.866025403784439,1.,0.866025403784439,
1.,0.866025403784439,1.,0.866025403784439,1.,0.866025403784439,1.,0.866025403784439,
1.,0.866025403784439,1.,0.866025403784439,1.,0.866025403784439,1.,0.866025403784439,
1.,0.866025403784439,1.,0.866025403784439,1.,0.866025403784439,1.,0.866025403784439,
1.,0.866025403784439,1.,0.866025403784439,1.,0.866025403784439,1.,0.866025403784439,
1.,0.866025403784439,1.,0.866025403784439,1.,0.866025403784439,1.,0.866025403784439,
1.,0.866025403784439,1.,0.866025403784439,1.,0.866025403784439,1.,0.866025403784439,
1.,0.866025403784439,1.,0.866025403784439,1.,0.866025403784439,1.,0.866025403784439,
1.,0.866025403784439,1.,0.866025403784439,1.,0.866025403784439,1.,0.866025403784439,
1.,0.866025403784439,1.,0.866025403784439,1.,0.866025403784439,1.,0.866025403784439,
1.,0.866025403784439,1.,0.866025403784439,1.,0.866025403784439,1.,0.866025403784439,
1.,0.866025403784439,1.,0.866025403784439,1.,0.866025403784439,1.,0.866025403784439,
1.,0.866025403784439,1.,0.866025403784439,1.,0.866025403784439,1.,0.866025403784439,
1.,0.866025403784439,1.,0.866025403784439,1.,0.866025403784439,1.,0.866025403784439,
1.,0.866025403784439,1.,0.866025403784439,1.,0.866025403784439,1.,0.866025403784439,
1.,0.866025403784439,1.,0.866025403784439,1.,0.866025403784439,1.,0.866025403784439,
1.,0.866025403784439,1.,0.866025403784439,1.,0.866025403784439,1.,0.866025403784439,
1.,0.866025403784439,1.,0.866025403784439,1.,0.866025403784439,1.,0.866025403784439,
1.,0.866025403784439,1.,0.866025403784439,1.,0.866025403784439,1.,0.866025403784439,
1.,0.866025403784439,1.,0.866025403784439,1.,0.866025403784439,1.,0.866025403784439,
1.,0.866025403784439,1.,0.866025403784439,1.,0.866025403784439,1.,0.866025403784439,
1.,0.866025403784439,1.,0.866025403784439,1.,0.866025403784439,1.,0.866025403784439,
1.,0.866025403784439,1.,0.866025403784439,1.,0.866025403784439,1.,0.866025403784439,
1.,0.866025403784439,1.,0.866025403784439,1.,0.866025403784439,1.,0.866025403784439,
1.,0.866025403784439,1.,0.866025403784439,1.,0.866025403784439,1.,0.866025403784439,
1.,0.866025403784439,1.,0.866025403784439,1.,0.866025403784439,1.,0.866025403784439,
1.,0.869328783748594,0.993556141390235)))
REPRESENTATION_ITEM('')
SURFACE()
);
#138=B_SPLINE_SURFACE_WITH_KNOTS('',1,3,((#28118,#28119,#28120,#28121,#28122,
#28123,#28124,#28125,#28126,#28127,#28128,#28129,#28130,#28131,#28132,#28133,
#28134,#28135,#28136,#28137,#28138,#28139,#28140,#28141,#28142,#28143,#28144,
#28145,#28146,#28147,#28148,#28149,#28150,#28151,#28152,#28153,#28154,#28155,
#28156,#28157,#28158,#28159,#28160,#28161,#28162,#28163,#28164,#28165,#28166,
#28167,#28168,#28169,#28170,#28171),(#28172,#28173,#28174,#28175,#28176,
#28177,#28178,#28179,#28180,#28181,#28182,#28183,#28184,#28185,#28186,#28187,
#28188,#28189,#28190,#28191,#28192,#28193,#28194,#28195,#28196,#28197,#28198,
#28199,#28200,#28201,#28202,#28203,#28204,#28205,#28206,#28207,#28208,#28209,
#28210,#28211,#28212,#28213,#28214,#28215,#28216,#28217,#28218,#28219,#28220,
#28221,#28222,#28223,#28224,#28225)),.UNSPECIFIED.,.F.,.F.,.F.,(2,2),(4,
2,2,2,2,2,2,2,2,2,2,2,2,2,2,2,2,2,2,2,2,2,2,2,2,2,4),(-0.00171316499800555,
1.),(-0.00171316499800555,0.015625,0.0234375,0.02734375,0.03125,0.046875,
0.0546875,0.0625,0.09375,0.125,0.1875,0.25,0.5,0.625,0.75,0.8125,0.84375,
0.875,0.90625,0.921875,0.9296875,0.9375,0.953125,0.9609375,0.96484375,0.96875,
1.00171316499801),.UNSPECIFIED.);
#139=B_SPLINE_SURFACE_WITH_KNOTS('',1,3,((#28230,#28231,#28232,#28233,#28234,
#28235,#28236,#28237,#28238,#28239,#28240,#28241,#28242,#28243,#28244,#28245,
#28246,#28247,#28248,#28249,#28250,#28251,#28252,#28253,#28254,#28255,#28256,
#28257,#28258,#28259,#28260,#28261,#28262,#28263,#28264,#28265,#28266,#28267,
#28268,#28269,#28270,#28271,#28272,#28273,#28274,#28275,#28276,#28277,#28278,
#28279,#28280,#28281,#28282,#28283),(#28284,#28285,#28286,#28287,#28288,
#28289,#28290,#28291,#28292,#28293,#28294,#28295,#28296,#28297,#28298,#28299,
#28300,#28301,#28302,#28303,#28304,#28305,#28306,#28307,#28308,#28309,#28310,
#28311,#28312,#28313,#28314,#28315,#28316,#28317,#28318,#28319,#28320,#28321,
#28322,#28323,#28324,#28325,#28326,#28327,#28328,#28329,#28330,#28331,#28332,
#28333,#28334,#28335,#28336,#28337)),.UNSPECIFIED.,.F.,.F.,.F.,(2,2),(4,
2,2,2,2,2,2,2,2,2,2,2,2,2,2,2,2,2,2,2,2,2,2,2,2,2,4),(-0.0017131650178696,
1.),(-0.00171316501786942,0.015625,0.0234375,0.02734375,0.03125,0.046875,
0.0546875,0.0625,0.09375,0.125,0.1875,0.25,0.5,0.625,0.75,0.8125,0.84375,
0.875,0.90625,0.921875,0.9296875,0.9375,0.953125,0.9609375,0.96484375,0.96875,
1.00171316501787),.UNSPECIFIED.);
#140=TOROIDAL_SURFACE('',#17973,11.5,1.00000000000001);
#141=TOROIDAL_SURFACE('',#17983,22.75,2.25);
#186=(
BOUNDED_CURVE()
B_SPLINE_CURVE(2,(#24977,#24978,#24979,#24980,#24981,#24982,#24983),
 .UNSPECIFIED.,.F.,.F.)
B_SPLINE_CURVE_WITH_KNOTS((3,2,2,3),(0.,0.00520833333333333,0.0104166666666667,
0.015625),.UNSPECIFIED.)
CURVE()
GEOMETRIC_REPRESENTATION_ITEM()
RATIONAL_B_SPLINE_CURVE((1.,0.866025403784439,1.,0.866025403784439,1.,0.866025403784439,
1.))
REPRESENTATION_ITEM('')
);
#187=(
BOUNDED_CURVE()
B_SPLINE_CURVE(2,(#24986,#24987,#24988,#24989,#24990,#24991,#24992),
 .UNSPECIFIED.,.F.,.F.)
B_SPLINE_CURVE_WITH_KNOTS((3,2,2,3),(0.,0.00520833333333333,0.0104166666666667,
0.015625),.UNSPECIFIED.)
CURVE()
GEOMETRIC_REPRESENTATION_ITEM()
RATIONAL_B_SPLINE_CURVE((1.,0.866025403784439,1.,0.866025403784439,1.,0.866025403784439,
1.))
REPRESENTATION_ITEM('')
);
#188=(
BOUNDED_CURVE()
B_SPLINE_CURVE(2,(#24997,#24998,#24999,#25000,#25001,#25002,#25003,#25004,
#25005,#25006,#25007,#25008,#25009),.UNSPECIFIED.,.F.,.F.)
B_SPLINE_CURVE_WITH_KNOTS((3,2,2,2,2,2,3),(0.015625,0.0208333333333333,
0.0260416666666667,0.03125,0.0364583333333333,0.0416666666666667,0.046875),
 .UNSPECIFIED.)
CURVE()
GEOMETRIC_REPRESENTATION_ITEM()
RATIONAL_B_SPLINE_CURVE((1.,0.866025403784439,1.,0.866025403784439,1.,0.866025403784439,
1.,0.866025403784439,1.,0.866025403784439,1.,0.866025403784439,1.))
REPRESENTATION_ITEM('')
);
#189=(
BOUNDED_CURVE()
B_SPLINE_CURVE(2,(#25010,#25011,#25012,#25013,#25014,#25015,#25016,#25017,
#25018,#25019,#25020,#25021,#25022),.UNSPECIFIED.,.F.,.F.)
B_SPLINE_CURVE_WITH_KNOTS((3,2,2,2,2,2,3),(0.015625,0.0208333333333333,
0.0260416666666667,0.03125,0.0364583333333333,0.0416666666666667,0.046875),
 .UNSPECIFIED.)
CURVE()
GEOMETRIC_REPRESENTATION_ITEM()
RATIONAL_B_SPLINE_CURVE((1.,0.866025403784439,1.,0.866025403784439,1.,0.866025403784439,
1.,0.866025403784439,1.,0.866025403784439,1.,0.866025403784439,1.))
REPRESENTATION_ITEM('')
);
#190=(
BOUNDED_CURVE()
B_SPLINE_CURVE(2,(#25027,#25028,#25029,#25030,#25031,#25032,#25033,#25034,
#25035,#25036,#25037,#25038,#25039),.UNSPECIFIED.,.F.,.F.)
B_SPLINE_CURVE_WITH_KNOTS((3,2,2,2,2,2,3),(0.046875,0.0520833333333333,
0.0572916666666667,0.0625,0.0677083333333333,0.0729166666666667,0.078125),
 .UNSPECIFIED.)
CURVE()
GEOMETRIC_REPRESENTATION_ITEM()
RATIONAL_B_SPLINE_CURVE((1.,0.866025403784439,1.,0.866025403784439,1.,0.866025403784439,
1.,0.866025403784439,1.,0.866025403784439,1.,0.866025403784439,1.))
REPRESENTATION_ITEM('')
);
#191=(
BOUNDED_CURVE()
B_SPLINE_CURVE(2,(#25040,#25041,#25042,#25043,#25044,#25045,#25046,#25047,
#25048,#25049,#25050,#25051,#25052),.UNSPECIFIED.,.F.,.F.)
B_SPLINE_CURVE_WITH_KNOTS((3,2,2,2,2,2,3),(0.046875,0.0520833333333333,
0.0572916666666667,0.0625,0.0677083333333333,0.0729166666666667,0.078125),
 .UNSPECIFIED.)
CURVE()
GEOMETRIC_REPRESENTATION_ITEM()
RATIONAL_B_SPLINE_CURVE((1.,0.866025403784439,1.,0.866025403784439,1.,0.866025403784439,
1.,0.866025403784439,1.,0.866025403784439,1.,0.866025403784439,1.))
REPRESENTATION_ITEM('')
);
#192=(
BOUNDED_CURVE()
B_SPLINE_CURVE(2,(#25057,#25058,#25059,#25060,#25061,#25062,#25063,#25064,
#25065,#25066,#25067,#25068,#25069),.UNSPECIFIED.,.F.,.F.)
B_SPLINE_CURVE_WITH_KNOTS((3,2,2,2,2,2,3),(0.078125,0.0833333333333333,
0.0885416666666667,0.09375,0.0989583333333333,0.104166666666667,0.109375),
 .UNSPECIFIED.)
CURVE()
GEOMETRIC_REPRESENTATION_ITEM()
RATIONAL_B_SPLINE_CURVE((1.,0.866025403784439,1.,0.866025403784439,1.,0.866025403784439,
1.,0.866025403784439,1.,0.866025403784439,1.,0.866025403784439,1.))
REPRESENTATION_ITEM('')
);
#193=(
BOUNDED_CURVE()
B_SPLINE_CURVE(2,(#25070,#25071,#25072,#25073,#25074,#25075,#25076,#25077,
#25078,#25079,#25080,#25081,#25082),.UNSPECIFIED.,.F.,.F.)
B_SPLINE_CURVE_WITH_KNOTS((3,2,2,2,2,2,3),(0.078125,0.0833333333333333,
0.0885416666666667,0.09375,0.0989583333333333,0.104166666666667,0.109375),
 .UNSPECIFIED.)
CURVE()
GEOMETRIC_REPRESENTATION_ITEM()
RATIONAL_B_SPLINE_CURVE((1.,0.866025403784439,1.,0.866025403784439,1.,0.866025403784439,
1.,0.866025403784439,1.,0.866025403784439,1.,0.866025403784439,1.))
REPRESENTATION_ITEM('')
);
#194=(
BOUNDED_CURVE()
B_SPLINE_CURVE(2,(#25087,#25088,#25089,#25090,#25091,#25092,#25093,#25094,
#25095,#25096,#25097,#25098,#25099),.UNSPECIFIED.,.F.,.F.)
B_SPLINE_CURVE_WITH_KNOTS((3,2,2,2,2,2,3),(0.109375,0.114583333333333,0.119791666666667,
0.125,0.130208333333333,0.135416666666667,0.140625),.UNSPECIFIED.)
CURVE()
GEOMETRIC_REPRESENTATION_ITEM()
RATIONAL_B_SPLINE_CURVE((1.,0.866025403784439,1.,0.866025403784439,1.,0.866025403784439,
1.,0.866025403784439,1.,0.866025403784439,1.,0.866025403784439,1.))
REPRESENTATION_ITEM('')
);
#195=(
BOUNDED_CURVE()
B_SPLINE_CURVE(2,(#25100,#25101,#25102,#25103,#25104,#25105,#25106,#25107,
#25108,#25109,#25110,#25111,#25112),.UNSPECIFIED.,.F.,.F.)
B_SPLINE_CURVE_WITH_KNOTS((3,2,2,2,2,2,3),(0.109375,0.114583333333333,0.119791666666667,
0.125,0.130208333333333,0.135416666666667,0.140625),.UNSPECIFIED.)
CURVE()
GEOMETRIC_REPRESENTATION_ITEM()
RATIONAL_B_SPLINE_CURVE((1.,0.866025403784439,1.,0.866025403784439,1.,0.866025403784439,
1.,0.866025403784439,1.,0.866025403784439,1.,0.866025403784439,1.))
REPRESENTATION_ITEM('')
);
#196=(
BOUNDED_CURVE()
B_SPLINE_CURVE(2,(#25117,#25118,#25119,#25120,#25121,#25122,#25123,#25124,
#25125,#25126,#25127,#25128,#25129),.UNSPECIFIED.,.F.,.F.)
B_SPLINE_CURVE_WITH_KNOTS((3,2,2,2,2,2,3),(0.140625,0.145833333333333,0.151041666666667,
0.15625,0.161458333333333,0.166666666666667,0.171875),.UNSPECIFIED.)
CURVE()
GEOMETRIC_REPRESENTATION_ITEM()
RATIONAL_B_SPLINE_CURVE((1.,0.866025403784439,1.,0.866025403784439,1.,0.866025403784439,
1.,0.866025403784439,1.,0.866025403784439,1.,0.866025403784439,1.))
REPRESENTATION_ITEM('')
);
#197=(
BOUNDED_CURVE()
B_SPLINE_CURVE(2,(#25130,#25131,#25132,#25133,#25134,#25135,#25136,#25137,
#25138,#25139,#25140,#25141,#25142),.UNSPECIFIED.,.F.,.F.)
B_SPLINE_CURVE_WITH_KNOTS((3,2,2,2,2,2,3),(0.140625,0.145833333333333,0.151041666666667,
0.15625,0.161458333333333,0.166666666666667,0.171875),.UNSPECIFIED.)
CURVE()
GEOMETRIC_REPRESENTATION_ITEM()
RATIONAL_B_SPLINE_CURVE((1.,0.866025403784439,1.,0.866025403784439,1.,0.866025403784439,
1.,0.866025403784439,1.,0.866025403784439,1.,0.866025403784439,1.))
REPRESENTATION_ITEM('')
);
#198=(
BOUNDED_CURVE()
B_SPLINE_CURVE(2,(#25147,#25148,#25149,#25150,#25151,#25152,#25153,#25154,
#25155,#25156,#25157,#25158,#25159),.UNSPECIFIED.,.F.,.F.)
B_SPLINE_CURVE_WITH_KNOTS((3,2,2,2,2,2,3),(0.171875,0.177083333333333,0.182291666666667,
0.1875,0.192708333333333,0.197916666666667,0.203125),.UNSPECIFIED.)
CURVE()
GEOMETRIC_REPRESENTATION_ITEM()
RATIONAL_B_SPLINE_CURVE((1.,0.866025403784439,1.,0.866025403784439,1.,0.866025403784439,
1.,0.866025403784439,1.,0.866025403784439,1.,0.866025403784439,1.))
REPRESENTATION_ITEM('')
);
#199=(
BOUNDED_CURVE()
B_SPLINE_CURVE(2,(#25160,#25161,#25162,#25163,#25164,#25165,#25166,#25167,
#25168,#25169,#25170,#25171,#25172),.UNSPECIFIED.,.F.,.F.)
B_SPLINE_CURVE_WITH_KNOTS((3,2,2,2,2,2,3),(0.171875,0.177083333333333,0.182291666666667,
0.1875,0.192708333333333,0.197916666666667,0.203125),.UNSPECIFIED.)
CURVE()
GEOMETRIC_REPRESENTATION_ITEM()
RATIONAL_B_SPLINE_CURVE((1.,0.866025403784439,1.,0.866025403784439,1.,0.866025403784439,
1.,0.866025403784439,1.,0.866025403784439,1.,0.866025403784439,1.))
REPRESENTATION_ITEM('')
);
#200=(
BOUNDED_CURVE()
B_SPLINE_CURVE(2,(#25177,#25178,#25179,#25180,#25181,#25182,#25183,#25184,
#25185,#25186,#25187,#25188,#25189),.UNSPECIFIED.,.F.,.F.)
B_SPLINE_CURVE_WITH_KNOTS((3,2,2,2,2,2,3),(0.203125,0.208333333333333,0.213541666666667,
0.21875,0.223958333333333,0.229166666666667,0.234375),.UNSPECIFIED.)
CURVE()
GEOMETRIC_REPRESENTATION_ITEM()
RATIONAL_B_SPLINE_CURVE((1.,0.866025403784439,1.,0.866025403784439,1.,0.866025403784439,
1.,0.866025403784439,1.,0.866025403784439,1.,0.866025403784439,1.))
REPRESENTATION_ITEM('')
);
#201=(
BOUNDED_CURVE()
B_SPLINE_CURVE(2,(#25190,#25191,#25192,#25193,#25194,#25195,#25196,#25197,
#25198,#25199,#25200,#25201,#25202),.UNSPECIFIED.,.F.,.F.)
B_SPLINE_CURVE_WITH_KNOTS((3,2,2,2,2,2,3),(0.203125,0.208333333333333,0.213541666666667,
0.21875,0.223958333333333,0.229166666666667,0.234375),.UNSPECIFIED.)
CURVE()
GEOMETRIC_REPRESENTATION_ITEM()
RATIONAL_B_SPLINE_CURVE((1.,0.866025403784439,1.,0.866025403784439,1.,0.866025403784439,
1.,0.866025403784439,1.,0.866025403784439,1.,0.866025403784439,1.))
REPRESENTATION_ITEM('')
);
#202=(
BOUNDED_CURVE()
B_SPLINE_CURVE(2,(#25207,#25208,#25209,#25210,#25211,#25212,#25213,#25214,
#25215,#25216,#25217,#25218,#25219),.UNSPECIFIED.,.F.,.F.)
B_SPLINE_CURVE_WITH_KNOTS((3,2,2,2,2,2,3),(0.234375,0.239583333333333,0.244791666666667,
0.25,0.255208333333333,0.260416666666667,0.265625),.UNSPECIFIED.)
CURVE()
GEOMETRIC_REPRESENTATION_ITEM()
RATIONAL_B_SPLINE_CURVE((1.,0.866025403784439,1.,0.866025403784439,1.,0.866025403784439,
1.,0.866025403784439,1.,0.866025403784439,1.,0.866025403784439,1.))
REPRESENTATION_ITEM('')
);
#203=(
BOUNDED_CURVE()
B_SPLINE_CURVE(2,(#25220,#25221,#25222,#25223,#25224,#25225,#25226,#25227,
#25228,#25229,#25230,#25231,#25232),.UNSPECIFIED.,.F.,.F.)
B_SPLINE_CURVE_WITH_KNOTS((3,2,2,2,2,2,3),(0.234375,0.239583333333333,0.244791666666667,
0.25,0.255208333333333,0.260416666666667,0.265625),.UNSPECIFIED.)
CURVE()
GEOMETRIC_REPRESENTATION_ITEM()
RATIONAL_B_SPLINE_CURVE((1.,0.866025403784439,1.,0.866025403784439,1.,0.866025403784439,
1.,0.866025403784439,1.,0.866025403784439,1.,0.866025403784439,1.))
REPRESENTATION_ITEM('')
);
#204=(
BOUNDED_CURVE()
B_SPLINE_CURVE(2,(#25237,#25238,#25239,#25240,#25241,#25242,#25243,#25244,
#25245,#25246,#25247,#25248,#25249),.UNSPECIFIED.,.F.,.F.)
B_SPLINE_CURVE_WITH_KNOTS((3,2,2,2,2,2,3),(0.265625,0.270833333333333,0.276041666666667,
0.28125,0.286458333333333,0.291666666666667,0.296875),.UNSPECIFIED.)
CURVE()
GEOMETRIC_REPRESENTATION_ITEM()
RATIONAL_B_SPLINE_CURVE((1.,0.866025403784439,1.,0.866025403784439,1.,0.866025403784439,
1.,0.866025403784439,1.,0.866025403784439,1.,0.866025403784439,1.))
REPRESENTATION_ITEM('')
);
#205=(
BOUNDED_CURVE()
B_SPLINE_CURVE(2,(#25250,#25251,#25252,#25253,#25254,#25255,#25256,#25257,
#25258,#25259,#25260,#25261,#25262),.UNSPECIFIED.,.F.,.F.)
B_SPLINE_CURVE_WITH_KNOTS((3,2,2,2,2,2,3),(0.265625,0.270833333333333,0.276041666666667,
0.28125,0.286458333333333,0.291666666666667,0.296875),.UNSPECIFIED.)
CURVE()
GEOMETRIC_REPRESENTATION_ITEM()
RATIONAL_B_SPLINE_CURVE((1.,0.866025403784439,1.,0.866025403784439,1.,0.866025403784439,
1.,0.866025403784439,1.,0.866025403784439,1.,0.866025403784439,1.))
REPRESENTATION_ITEM('')
);
#206=(
BOUNDED_CURVE()
B_SPLINE_CURVE(2,(#25267,#25268,#25269,#25270,#25271,#25272,#25273,#25274,
#25275,#25276,#25277,#25278,#25279),.UNSPECIFIED.,.F.,.F.)
B_SPLINE_CURVE_WITH_KNOTS((3,2,2,2,2,2,3),(0.296875,0.302083333333333,0.307291666666667,
0.3125,0.317708333333333,0.322916666666667,0.328125),.UNSPECIFIED.)
CURVE()
GEOMETRIC_REPRESENTATION_ITEM()
RATIONAL_B_SPLINE_CURVE((1.,0.866025403784439,1.,0.866025403784439,1.,0.866025403784439,
1.,0.866025403784439,1.,0.866025403784439,1.,0.866025403784439,1.))
REPRESENTATION_ITEM('')
);
#207=(
BOUNDED_CURVE()
B_SPLINE_CURVE(2,(#25280,#25281,#25282,#25283,#25284,#25285,#25286,#25287,
#25288,#25289,#25290,#25291,#25292),.UNSPECIFIED.,.F.,.F.)
B_SPLINE_CURVE_WITH_KNOTS((3,2,2,2,2,2,3),(0.296875,0.302083333333333,0.307291666666667,
0.3125,0.317708333333333,0.322916666666667,0.328125),.UNSPECIFIED.)
CURVE()
GEOMETRIC_REPRESENTATION_ITEM()
RATIONAL_B_SPLINE_CURVE((1.,0.866025403784439,1.,0.866025403784439,1.,0.866025403784439,
1.,0.866025403784439,1.,0.866025403784439,1.,0.866025403784439,1.))
REPRESENTATION_ITEM('')
);
#208=(
BOUNDED_CURVE()
B_SPLINE_CURVE(2,(#25297,#25298,#25299,#25300,#25301,#25302,#25303,#25304,
#25305,#25306,#25307,#25308,#25309),.UNSPECIFIED.,.F.,.F.)
B_SPLINE_CURVE_WITH_KNOTS((3,2,2,2,2,2,3),(0.328125,0.333333333333333,0.338541666666667,
0.34375,0.348958333333333,0.354166666666667,0.359375),.UNSPECIFIED.)
CURVE()
GEOMETRIC_REPRESENTATION_ITEM()
RATIONAL_B_SPLINE_CURVE((1.,0.866025403784439,1.,0.866025403784439,1.,0.866025403784439,
1.,0.866025403784439,1.,0.866025403784439,1.,0.866025403784439,1.))
REPRESENTATION_ITEM('')
);
#209=(
BOUNDED_CURVE()
B_SPLINE_CURVE(2,(#25310,#25311,#25312,#25313,#25314,#25315,#25316,#25317,
#25318,#25319,#25320,#25321,#25322),.UNSPECIFIED.,.F.,.F.)
B_SPLINE_CURVE_WITH_KNOTS((3,2,2,2,2,2,3),(0.328125,0.333333333333333,0.338541666666667,
0.34375,0.348958333333333,0.354166666666667,0.359375),.UNSPECIFIED.)
CURVE()
GEOMETRIC_REPRESENTATION_ITEM()
RATIONAL_B_SPLINE_CURVE((1.,0.866025403784439,1.,0.866025403784439,1.,0.866025403784439,
1.,0.866025403784439,1.,0.866025403784439,1.,0.866025403784439,1.))
REPRESENTATION_ITEM('')
);
#210=(
BOUNDED_CURVE()
B_SPLINE_CURVE(2,(#25327,#25328,#25329,#25330,#25331,#25332,#25333,#25334,
#25335,#25336,#25337,#25338,#25339),.UNSPECIFIED.,.F.,.F.)
B_SPLINE_CURVE_WITH_KNOTS((3,2,2,2,2,2,3),(0.359375,0.364583333333333,0.369791666666667,
0.375,0.380208333333333,0.385416666666667,0.390625),.UNSPECIFIED.)
CURVE()
GEOMETRIC_REPRESENTATION_ITEM()
RATIONAL_B_SPLINE_CURVE((1.,0.866025403784439,1.,0.866025403784439,1.,0.866025403784439,
1.,0.866025403784439,1.,0.866025403784439,1.,0.866025403784439,1.))
REPRESENTATION_ITEM('')
);
#211=(
BOUNDED_CURVE()
B_SPLINE_CURVE(2,(#25340,#25341,#25342,#25343,#25344,#25345,#25346,#25347,
#25348,#25349,#25350,#25351,#25352),.UNSPECIFIED.,.F.,.F.)
B_SPLINE_CURVE_WITH_KNOTS((3,2,2,2,2,2,3),(0.359375,0.364583333333333,0.369791666666667,
0.375,0.380208333333333,0.385416666666667,0.390625),.UNSPECIFIED.)
CURVE()
GEOMETRIC_REPRESENTATION_ITEM()
RATIONAL_B_SPLINE_CURVE((1.,0.866025403784439,1.,0.866025403784439,1.,0.866025403784439,
1.,0.866025403784439,1.,0.866025403784439,1.,0.866025403784439,1.))
REPRESENTATION_ITEM('')
);
#212=(
BOUNDED_CURVE()
B_SPLINE_CURVE(2,(#25357,#25358,#25359,#25360,#25361,#25362,#25363,#25364,
#25365,#25366,#25367,#25368,#25369),.UNSPECIFIED.,.F.,.F.)
B_SPLINE_CURVE_WITH_KNOTS((3,2,2,2,2,2,3),(0.390625,0.395833333333333,0.401041666666667,
0.40625,0.411458333333333,0.416666666666667,0.421875),.UNSPECIFIED.)
CURVE()
GEOMETRIC_REPRESENTATION_ITEM()
RATIONAL_B_SPLINE_CURVE((1.,0.866025403784439,1.,0.866025403784439,1.,0.866025403784439,
1.,0.866025403784439,1.,0.866025403784439,1.,0.866025403784439,1.))
REPRESENTATION_ITEM('')
);
#213=(
BOUNDED_CURVE()
B_SPLINE_CURVE(2,(#25370,#25371,#25372,#25373,#25374,#25375,#25376,#25377,
#25378,#25379,#25380,#25381,#25382),.UNSPECIFIED.,.F.,.F.)
B_SPLINE_CURVE_WITH_KNOTS((3,2,2,2,2,2,3),(0.390625,0.395833333333333,0.401041666666667,
0.40625,0.411458333333333,0.416666666666667,0.421875),.UNSPECIFIED.)
CURVE()
GEOMETRIC_REPRESENTATION_ITEM()
RATIONAL_B_SPLINE_CURVE((1.,0.866025403784439,1.,0.866025403784439,1.,0.866025403784439,
1.,0.866025403784439,1.,0.866025403784439,1.,0.866025403784439,1.))
REPRESENTATION_ITEM('')
);
#214=(
BOUNDED_CURVE()
B_SPLINE_CURVE(2,(#25387,#25388,#25389,#25390,#25391,#25392,#25393,#25394,
#25395,#25396,#25397,#25398,#25399),.UNSPECIFIED.,.F.,.F.)
B_SPLINE_CURVE_WITH_KNOTS((3,2,2,2,2,2,3),(0.421875,0.427083333333333,0.432291666666667,
0.4375,0.442708333333333,0.447916666666667,0.453125),.UNSPECIFIED.)
CURVE()
GEOMETRIC_REPRESENTATION_ITEM()
RATIONAL_B_SPLINE_CURVE((1.,0.866025403784439,1.,0.866025403784439,1.,0.866025403784439,
1.,0.866025403784439,1.,0.866025403784439,1.,0.866025403784439,1.))
REPRESENTATION_ITEM('')
);
#215=(
BOUNDED_CURVE()
B_SPLINE_CURVE(2,(#25400,#25401,#25402,#25403,#25404,#25405,#25406,#25407,
#25408,#25409,#25410,#25411,#25412),.UNSPECIFIED.,.F.,.F.)
B_SPLINE_CURVE_WITH_KNOTS((3,2,2,2,2,2,3),(0.421875,0.427083333333333,0.432291666666667,
0.4375,0.442708333333333,0.447916666666667,0.453125),.UNSPECIFIED.)
CURVE()
GEOMETRIC_REPRESENTATION_ITEM()
RATIONAL_B_SPLINE_CURVE((1.,0.866025403784439,1.,0.866025403784439,1.,0.866025403784439,
1.,0.866025403784439,1.,0.866025403784439,1.,0.866025403784439,1.))
REPRESENTATION_ITEM('')
);
#216=(
BOUNDED_CURVE()
B_SPLINE_CURVE(2,(#25417,#25418,#25419,#25420,#25421,#25422,#25423,#25424,
#25425,#25426,#25427,#25428,#25429),.UNSPECIFIED.,.F.,.F.)
B_SPLINE_CURVE_WITH_KNOTS((3,2,2,2,2,2,3),(0.453125,0.458333333333333,0.463541666666667,
0.46875,0.473958333333333,0.479166666666667,0.484375),.UNSPECIFIED.)
CURVE()
GEOMETRIC_REPRESENTATION_ITEM()
RATIONAL_B_SPLINE_CURVE((1.,0.866025403784439,1.,0.866025403784439,1.,0.866025403784439,
1.,0.866025403784439,1.,0.866025403784439,1.,0.866025403784439,1.))
REPRESENTATION_ITEM('')
);
#217=(
BOUNDED_CURVE()
B_SPLINE_CURVE(2,(#25430,#25431,#25432,#25433,#25434,#25435,#25436,#25437,
#25438,#25439,#25440,#25441,#25442),.UNSPECIFIED.,.F.,.F.)
B_SPLINE_CURVE_WITH_KNOTS((3,2,2,2,2,2,3),(0.453125,0.458333333333333,0.463541666666667,
0.46875,0.473958333333333,0.479166666666667,0.484375),.UNSPECIFIED.)
CURVE()
GEOMETRIC_REPRESENTATION_ITEM()
RATIONAL_B_SPLINE_CURVE((1.,0.866025403784439,1.,0.866025403784439,1.,0.866025403784439,
1.,0.866025403784439,1.,0.866025403784439,1.,0.866025403784439,1.))
REPRESENTATION_ITEM('')
);
#218=(
BOUNDED_CURVE()
B_SPLINE_CURVE(2,(#25447,#25448,#25449,#25450,#25451,#25452,#25453,#25454,
#25455,#25456,#25457,#25458,#25459),.UNSPECIFIED.,.F.,.F.)
B_SPLINE_CURVE_WITH_KNOTS((3,2,2,2,2,2,3),(0.484375,0.489583333333333,0.494791666666667,
0.5,0.505208333333333,0.510416666666667,0.515625),.UNSPECIFIED.)
CURVE()
GEOMETRIC_REPRESENTATION_ITEM()
RATIONAL_B_SPLINE_CURVE((1.,0.866025403784439,1.,0.866025403784439,1.,0.866025403784439,
1.,0.866025403784439,1.,0.866025403784439,1.,0.866025403784439,1.))
REPRESENTATION_ITEM('')
);
#219=(
BOUNDED_CURVE()
B_SPLINE_CURVE(2,(#25460,#25461,#25462,#25463,#25464,#25465,#25466,#25467,
#25468,#25469,#25470,#25471,#25472),.UNSPECIFIED.,.F.,.F.)
B_SPLINE_CURVE_WITH_KNOTS((3,2,2,2,2,2,3),(0.484375,0.489583333333333,0.494791666666667,
0.5,0.505208333333333,0.510416666666667,0.515625),.UNSPECIFIED.)
CURVE()
GEOMETRIC_REPRESENTATION_ITEM()
RATIONAL_B_SPLINE_CURVE((1.,0.866025403784439,1.,0.866025403784439,1.,0.866025403784439,
1.,0.866025403784439,1.,0.866025403784439,1.,0.866025403784439,1.))
REPRESENTATION_ITEM('')
);
#220=(
BOUNDED_CURVE()
B_SPLINE_CURVE(2,(#25477,#25478,#25479,#25480,#25481,#25482,#25483,#25484,
#25485,#25486,#25487,#25488,#25489),.UNSPECIFIED.,.F.,.F.)
B_SPLINE_CURVE_WITH_KNOTS((3,2,2,2,2,2,3),(0.515625,0.520833333333333,0.526041666666667,
0.53125,0.536458333333333,0.541666666666667,0.546875),.UNSPECIFIED.)
CURVE()
GEOMETRIC_REPRESENTATION_ITEM()
RATIONAL_B_SPLINE_CURVE((1.,0.866025403784439,1.,0.866025403784439,1.,0.866025403784439,
1.,0.866025403784439,1.,0.866025403784439,1.,0.866025403784439,1.))
REPRESENTATION_ITEM('')
);
#221=(
BOUNDED_CURVE()
B_SPLINE_CURVE(2,(#25490,#25491,#25492,#25493,#25494,#25495,#25496,#25497,
#25498,#25499,#25500,#25501,#25502),.UNSPECIFIED.,.F.,.F.)
B_SPLINE_CURVE_WITH_KNOTS((3,2,2,2,2,2,3),(0.515625,0.520833333333333,0.526041666666667,
0.53125,0.536458333333333,0.541666666666667,0.546875),.UNSPECIFIED.)
CURVE()
GEOMETRIC_REPRESENTATION_ITEM()
RATIONAL_B_SPLINE_CURVE((1.,0.866025403784439,1.,0.866025403784439,1.,0.866025403784439,
1.,0.866025403784439,1.,0.866025403784439,1.,0.866025403784439,1.))
REPRESENTATION_ITEM('')
);
#222=(
BOUNDED_CURVE()
B_SPLINE_CURVE(2,(#25507,#25508,#25509,#25510,#25511,#25512,#25513,#25514,
#25515,#25516,#25517,#25518,#25519),.UNSPECIFIED.,.F.,.F.)
B_SPLINE_CURVE_WITH_KNOTS((3,2,2,2,2,2,3),(0.546875,0.552083333333333,0.557291666666667,
0.5625,0.567708333333333,0.572916666666667,0.578125),.UNSPECIFIED.)
CURVE()
GEOMETRIC_REPRESENTATION_ITEM()
RATIONAL_B_SPLINE_CURVE((1.,0.866025403784439,1.,0.866025403784439,1.,0.866025403784439,
1.,0.866025403784439,1.,0.866025403784439,1.,0.866025403784439,1.))
REPRESENTATION_ITEM('')
);
#223=(
BOUNDED_CURVE()
B_SPLINE_CURVE(2,(#25520,#25521,#25522,#25523,#25524,#25525,#25526,#25527,
#25528,#25529,#25530,#25531,#25532),.UNSPECIFIED.,.F.,.F.)
B_SPLINE_CURVE_WITH_KNOTS((3,2,2,2,2,2,3),(0.546875,0.552083333333333,0.557291666666667,
0.5625,0.567708333333333,0.572916666666667,0.578125),.UNSPECIFIED.)
CURVE()
GEOMETRIC_REPRESENTATION_ITEM()
RATIONAL_B_SPLINE_CURVE((1.,0.866025403784439,1.,0.866025403784439,1.,0.866025403784439,
1.,0.866025403784439,1.,0.866025403784439,1.,0.866025403784439,1.))
REPRESENTATION_ITEM('')
);
#224=(
BOUNDED_CURVE()
B_SPLINE_CURVE(2,(#25537,#25538,#25539,#25540,#25541,#25542,#25543,#25544,
#25545,#25546,#25547,#25548,#25549),.UNSPECIFIED.,.F.,.F.)
B_SPLINE_CURVE_WITH_KNOTS((3,2,2,2,2,2,3),(0.578125,0.583333333333333,0.588541666666667,
0.59375,0.598958333333333,0.604166666666667,0.609375),.UNSPECIFIED.)
CURVE()
GEOMETRIC_REPRESENTATION_ITEM()
RATIONAL_B_SPLINE_CURVE((1.,0.866025403784439,1.,0.866025403784439,1.,0.866025403784439,
1.,0.866025403784439,1.,0.866025403784439,1.,0.866025403784439,1.))
REPRESENTATION_ITEM('')
);
#225=(
BOUNDED_CURVE()
B_SPLINE_CURVE(2,(#25550,#25551,#25552,#25553,#25554,#25555,#25556,#25557,
#25558,#25559,#25560,#25561,#25562),.UNSPECIFIED.,.F.,.F.)
B_SPLINE_CURVE_WITH_KNOTS((3,2,2,2,2,2,3),(0.578125,0.583333333333333,0.588541666666667,
0.59375,0.598958333333333,0.604166666666667,0.609375),.UNSPECIFIED.)
CURVE()
GEOMETRIC_REPRESENTATION_ITEM()
RATIONAL_B_SPLINE_CURVE((1.,0.866025403784439,1.,0.866025403784439,1.,0.866025403784439,
1.,0.866025403784439,1.,0.866025403784439,1.,0.866025403784439,1.))
REPRESENTATION_ITEM('')
);
#226=(
BOUNDED_CURVE()
B_SPLINE_CURVE(2,(#25567,#25568,#25569,#25570,#25571,#25572,#25573,#25574,
#25575,#25576,#25577,#25578,#25579),.UNSPECIFIED.,.F.,.F.)
B_SPLINE_CURVE_WITH_KNOTS((3,2,2,2,2,2,3),(0.609375,0.614583333333333,0.619791666666667,
0.625,0.630208333333333,0.635416666666667,0.640625),.UNSPECIFIED.)
CURVE()
GEOMETRIC_REPRESENTATION_ITEM()
RATIONAL_B_SPLINE_CURVE((1.,0.866025403784439,1.,0.866025403784439,1.,0.866025403784439,
1.,0.866025403784439,1.,0.866025403784439,1.,0.866025403784439,1.))
REPRESENTATION_ITEM('')
);
#227=(
BOUNDED_CURVE()
B_SPLINE_CURVE(2,(#25580,#25581,#25582,#25583,#25584,#25585,#25586,#25587,
#25588,#25589,#25590,#25591,#25592),.UNSPECIFIED.,.F.,.F.)
B_SPLINE_CURVE_WITH_KNOTS((3,2,2,2,2,2,3),(0.609375,0.614583333333333,0.619791666666667,
0.625,0.630208333333333,0.635416666666667,0.640625),.UNSPECIFIED.)
CURVE()
GEOMETRIC_REPRESENTATION_ITEM()
RATIONAL_B_SPLINE_CURVE((1.,0.866025403784439,1.,0.866025403784439,1.,0.866025403784439,
1.,0.866025403784439,1.,0.866025403784439,1.,0.866025403784439,1.))
REPRESENTATION_ITEM('')
);
#228=(
BOUNDED_CURVE()
B_SPLINE_CURVE(2,(#25597,#25598,#25599,#25600,#25601,#25602,#25603,#25604,
#25605,#25606,#25607,#25608,#25609),.UNSPECIFIED.,.F.,.F.)
B_SPLINE_CURVE_WITH_KNOTS((3,2,2,2,2,2,3),(0.640625,0.645833333333333,0.651041666666667,
0.65625,0.661458333333333,0.666666666666667,0.671875),.UNSPECIFIED.)
CURVE()
GEOMETRIC_REPRESENTATION_ITEM()
RATIONAL_B_SPLINE_CURVE((1.,0.866025403784439,1.,0.866025403784439,1.,0.866025403784439,
1.,0.866025403784439,1.,0.866025403784439,1.,0.866025403784439,1.))
REPRESENTATION_ITEM('')
);
#229=(
BOUNDED_CURVE()
B_SPLINE_CURVE(2,(#25610,#25611,#25612,#25613,#25614,#25615,#25616,#25617,
#25618,#25619,#25620,#25621,#25622),.UNSPECIFIED.,.F.,.F.)
B_SPLINE_CURVE_WITH_KNOTS((3,2,2,2,2,2,3),(0.640625,0.645833333333333,0.651041666666667,
0.65625,0.661458333333333,0.666666666666667,0.671875),.UNSPECIFIED.)
CURVE()
GEOMETRIC_REPRESENTATION_ITEM()
RATIONAL_B_SPLINE_CURVE((1.,0.866025403784439,1.,0.866025403784439,1.,0.866025403784439,
1.,0.866025403784439,1.,0.866025403784439,1.,0.866025403784439,1.))
REPRESENTATION_ITEM('')
);
#230=(
BOUNDED_CURVE()
B_SPLINE_CURVE(2,(#25627,#25628,#25629,#25630,#25631,#25632,#25633,#25634,
#25635,#25636,#25637,#25638,#25639),.UNSPECIFIED.,.F.,.F.)
B_SPLINE_CURVE_WITH_KNOTS((3,2,2,2,2,2,3),(0.671875,0.677083333333333,0.682291666666667,
0.6875,0.692708333333333,0.697916666666667,0.703125),.UNSPECIFIED.)
CURVE()
GEOMETRIC_REPRESENTATION_ITEM()
RATIONAL_B_SPLINE_CURVE((1.,0.866025403784439,1.,0.866025403784439,1.,0.866025403784439,
1.,0.866025403784439,1.,0.866025403784439,1.,0.866025403784439,1.))
REPRESENTATION_ITEM('')
);
#231=(
BOUNDED_CURVE()
B_SPLINE_CURVE(2,(#25640,#25641,#25642,#25643,#25644,#25645,#25646,#25647,
#25648,#25649,#25650,#25651,#25652),.UNSPECIFIED.,.F.,.F.)
B_SPLINE_CURVE_WITH_KNOTS((3,2,2,2,2,2,3),(0.671875,0.677083333333333,0.682291666666667,
0.6875,0.692708333333333,0.697916666666667,0.703125),.UNSPECIFIED.)
CURVE()
GEOMETRIC_REPRESENTATION_ITEM()
RATIONAL_B_SPLINE_CURVE((1.,0.866025403784439,1.,0.866025403784439,1.,0.866025403784439,
1.,0.866025403784439,1.,0.866025403784439,1.,0.866025403784439,1.))
REPRESENTATION_ITEM('')
);
#232=(
BOUNDED_CURVE()
B_SPLINE_CURVE(2,(#25657,#25658,#25659,#25660,#25661,#25662,#25663,#25664,
#25665,#25666,#25667,#25668,#25669),.UNSPECIFIED.,.F.,.F.)
B_SPLINE_CURVE_WITH_KNOTS((3,2,2,2,2,2,3),(0.703125,0.708333333333333,0.713541666666667,
0.71875,0.723958333333333,0.729166666666667,0.734375),.UNSPECIFIED.)
CURVE()
GEOMETRIC_REPRESENTATION_ITEM()
RATIONAL_B_SPLINE_CURVE((1.,0.866025403784439,1.,0.866025403784439,1.,0.866025403784439,
1.,0.866025403784439,1.,0.866025403784439,1.,0.866025403784439,1.))
REPRESENTATION_ITEM('')
);
#233=(
BOUNDED_CURVE()
B_SPLINE_CURVE(2,(#25670,#25671,#25672,#25673,#25674,#25675,#25676,#25677,
#25678,#25679,#25680,#25681,#25682),.UNSPECIFIED.,.F.,.F.)
B_SPLINE_CURVE_WITH_KNOTS((3,2,2,2,2,2,3),(0.703125,0.708333333333333,0.713541666666667,
0.71875,0.723958333333333,0.729166666666667,0.734375),.UNSPECIFIED.)
CURVE()
GEOMETRIC_REPRESENTATION_ITEM()
RATIONAL_B_SPLINE_CURVE((1.,0.866025403784439,1.,0.866025403784439,1.,0.866025403784439,
1.,0.866025403784439,1.,0.866025403784439,1.,0.866025403784439,1.))
REPRESENTATION_ITEM('')
);
#234=(
BOUNDED_CURVE()
B_SPLINE_CURVE(2,(#25688,#25689,#25690,#25691,#25692),.UNSPECIFIED.,.F.,
 .F.)
B_SPLINE_CURVE_WITH_KNOTS((3,2,3),(0.765625,0.770833333333333,0.771318117457215),
 .UNSPECIFIED.)
CURVE()
GEOMETRIC_REPRESENTATION_ITEM()
RATIONAL_B_SPLINE_CURVE((1.,0.866025403784439,1.,0.987529838608244,0.977381086342234))
REPRESENTATION_ITEM('')
);
#235=(
BOUNDED_CURVE()
B_SPLINE_CURVE(2,(#25695,#25696,#25697,#25698,#25699),.UNSPECIFIED.,.F.,
 .F.)
B_SPLINE_CURVE_WITH_KNOTS((3,2,3),(0.765625,0.770833333333333,0.775106737579528),
 .UNSPECIFIED.)
CURVE()
GEOMETRIC_REPRESENTATION_ITEM()
RATIONAL_B_SPLINE_CURVE((1.,0.866025403784439,1.,0.890074699196848,0.960535413324785))
REPRESENTATION_ITEM('')
);
#236=(
BOUNDED_CURVE()
B_SPLINE_CURVE(2,(#28344,#28345,#28346,#28347,#28348,#28349,#28350,#28351,
#28352,#28353,#28354,#28355,#28356),.UNSPECIFIED.,.F.,.F.)
B_SPLINE_CURVE_WITH_KNOTS((3,2,2,2,2,2,3),(0.734375,0.739583333333333,0.744791666666667,
0.75,0.755208333333333,0.760416666666667,0.765625),.UNSPECIFIED.)
CURVE()
GEOMETRIC_REPRESENTATION_ITEM()
RATIONAL_B_SPLINE_CURVE((1.,0.866025403784439,1.,0.866025403784439,1.,0.866025403784439,
1.,0.866025403784439,1.,0.866025403784439,1.,0.866025403784439,1.))
REPRESENTATION_ITEM('')
);
#237=(
BOUNDED_CURVE()
B_SPLINE_CURVE(2,(#28357,#28358,#28359,#28360,#28361,#28362,#28363,#28364,
#28365,#28366,#28367,#28368,#28369),.UNSPECIFIED.,.F.,.F.)
B_SPLINE_CURVE_WITH_KNOTS((3,2,2,2,2,2,3),(0.734375,0.739583333333333,0.744791666666667,
0.75,0.755208333333333,0.760416666666667,0.765625),.UNSPECIFIED.)
CURVE()
GEOMETRIC_REPRESENTATION_ITEM()
RATIONAL_B_SPLINE_CURVE((1.,0.866025403784439,1.,0.866025403784439,1.,0.866025403784439,
1.,0.866025403784439,1.,0.866025403784439,1.,0.866025403784439,1.))
REPRESENTATION_ITEM('')
);
#864=FACE_BOUND('',#2779,.T.);
#865=FACE_BOUND('',#2781,.T.);
#866=FACE_BOUND('',#2783,.T.);
#867=FACE_BOUND('',#2785,.T.);
#868=FACE_BOUND('',#2787,.T.);
#908=B_SPLINE_CURVE_WITH_KNOTS('',3,(#25706,#25707,#25708,#25709,#25710,
#25711,#25712,#25713,#25714,#25715,#25716,#25717,#25718,#25719,#25720,#25721,
#25722,#25723,#25724,#25725,#25726,#25727,#25728,#25729,#25730,#25731,#25732,
#25733,#25734,#25735,#25736,#25737,#25738,#25739,#25740,#25741),
 .UNSPECIFIED.,.F.,.F.,(4,2,2,2,2,2,2,2,2,2,2,2,2,2,2,2,2,4),(0.,0.0855939099291143,
0.17410949539989,0.337900796524859,0.497108066486332,0.656524415442333,
0.820403798482143,0.977076652433585,1.1382988894702,1.30211536903791,1.45920718825481,
1.6223913309354,1.78298213056648,1.94186476292235,2.10710718046966,2.26419884117872,
2.42492153336099,2.58541477279612),.UNSPECIFIED.);
#909=B_SPLINE_CURVE_WITH_KNOTS('',3,(#25747,#25748,#25749,#25750,#25751,
#25752,#25753,#25754,#25755,#25756,#25757,#25758,#25759,#25760,#25761,#25762,
#25763,#25764,#25765,#25766,#25767,#25768,#25769,#25770,#25771,#25772,#25773,
#25774,#25775,#25776,#25777,#25778,#25779,#25780,#25781,#25782),
 .UNSPECIFIED.,.F.,.F.,(4,2,2,2,2,2,2,2,2,2,2,2,2,2,2,2,2,4),(60.7773622036861,
60.7984307512578,60.9623015973858,61.1221066343054,61.2805211858834,61.444748688821,
61.6027543469895,61.7661864642053,61.9283577950001,62.0848598014743,62.2487106901294,
62.4090254078727,62.5666049251944,62.7313988978381,62.889895395675,63.0516314776395,
63.2095616444729,63.3630379643741),.UNSPECIFIED.);
#910=B_SPLINE_CURVE_WITH_KNOTS('',3,(#25785,#25786,#25787,#25788,#25789,
#25790,#25791,#25792,#25793,#25794,#25795,#25796,#25797,#25798,#25799,#25800,
#25801,#25802,#25803,#25804,#25805,#25806,#25807,#25808,#25809,#25810,#25811,
#25812,#25813,#25814,#25815,#25816,#25817,#25818,#25819,#25820,#25821,#25822),
 .UNSPECIFIED.,.F.,.F.,(4,2,2,2,2,2,2,2,2,2,2,2,2,2,2,2,2,2,4),(2.58541477279612,
2.58875674058881,2.74542529180111,2.90803801163507,3.07013217269297,3.22851746172615,
3.39318279931958,3.55092904348818,3.71112742512023,3.87498226727406,4.0314645454848,
4.19351122166086,4.35734638384252,4.51524546689183,4.67935054595871,4.83797716078043,
4.99767285707326,5.1615476489584,5.1855645153609),.UNSPECIFIED.);
#911=B_SPLINE_CURVE_WITH_KNOTS('',3,(#25827,#25828,#25829,#25830,#25831,
#25832,#25833,#25834,#25835,#25836,#25837,#25838,#25839,#25840,#25841,#25842,
#25843,#25844,#25845,#25846,#25847,#25848,#25849,#25850,#25851,#25852,#25853,
#25854,#25855,#25856,#25857,#25858,#25859,#25860,#25861,#25862),
 .UNSPECIFIED.,.F.,.F.,(4,2,2,2,2,2,2,2,2,2,2,2,2,2,2,2,2,4),(58.1771396961264,
58.224613592811,58.3897391041826,58.5485203454945,58.7093619904073,58.8724312620513,
59.0294255289243,59.1932370819247,59.3543749967249,59.5111139777451,59.6750046303897,
59.8343399231803,59.9937618262344,60.1574607072996,60.315005213044,60.4802904170643,
60.6419193578722,60.7773622036861),.UNSPECIFIED.);
#912=B_SPLINE_CURVE_WITH_KNOTS('',3,(#25863,#25864,#25865,#25866,#25867,
#25868,#25869,#25870,#25871,#25872,#25873,#25874,#25875,#25876,#25877,#25878,
#25879,#25880,#25881,#25882,#25883,#25884,#25885,#25886,#25887,#25888,#25889,
#25890,#25891,#25892,#25893,#25894,#25895,#25896,#25897,#25898),
 .UNSPECIFIED.,.F.,.F.,(4,2,2,2,2,2,2,2,2,2,2,2,2,2,2,2,2,4),(5.1855645153609,
5.31809241175765,5.47960631614643,5.64345734077483,5.80083607956624,5.96434590256516,
6.12417910937735,6.28334770275447,6.44892428370015,6.60574353245866,6.76677257273097,
6.93059221744087,7.08748561288601,7.25043434000472,7.41159722098884,7.57027369545872,
7.73527696164013,7.78581990814952),.UNSPECIFIED.);
#913=B_SPLINE_CURVE_WITH_KNOTS('',3,(#25903,#25904,#25905,#25906,#25907,
#25908,#25909,#25910,#25911,#25912,#25913,#25914,#25915,#25916,#25917,#25918,
#25919,#25920,#25921,#25922,#25923,#25924,#25925,#25926,#25927,#25928,#25929,
#25930,#25931,#25932,#25933,#25934,#25935,#25936,#25937,#25938),
 .UNSPECIFIED.,.F.,.F.,(4,2,2,2,2,2,2,2,2,2,2,2,2,2,2,2,2,4),(55.5770402575689,
55.6524503192492,55.8164457466301,55.974248469311,56.1384186057709,56.3003534752986,
56.4568207460609,56.620670390864,56.7807635929306,56.9386504233684,57.1031998344716,
57.2614839345338,57.4238795946348,57.5863762730804,57.7429819545077,57.9068118223431,
58.0674272232114,58.1771396961264),.UNSPECIFIED.);
#914=B_SPLINE_CURVE_WITH_KNOTS('',3,(#25939,#25940,#25941,#25942,#25943,
#25944,#25945,#25946,#25947,#25948,#25949,#25950,#25951,#25952,#25953,#25954,
#25955,#25956,#25957,#25958,#25959,#25960,#25961,#25962,#25963,#25964,#25965,
#25966,#25967,#25968,#25969,#25970,#25971,#25972,#25973,#25974),
 .UNSPECIFIED.,.F.,.F.,(4,2,2,2,2,2,2,2,2,2,2,2,2,2,2,2,2,4),(7.78581990814952,
7.89259977417174,8.05310409347892,8.21694253542575,8.37350006053866,8.53587605970679,
8.6986491541994,8.85682980243783,9.0212593655275,9.17933464700114,9.33932036571389,
9.50317869408483,9.65965348486788,9.82147380855276,9.98605555221982,10.1437614501634,
10.307645465901,10.3859883446169),.UNSPECIFIED.);
#915=B_SPLINE_CURVE_WITH_KNOTS('',3,(#25979,#25980,#25981,#25982,#25983,
#25984,#25985,#25986,#25987,#25988,#25989,#25990,#25991,#25992,#25993,#25994,
#25995,#25996,#25997,#25998,#25999,#26000,#26001,#26002,#26003,#26004,#26005,
#26006,#26007,#26008,#26009,#26010,#26011,#26012,#26013,#26014),
 .UNSPECIFIED.,.F.,.F.,(4,2,2,2,2,2,2,2,2,2,2,2,2,2,2,2,2,4),(52.9768680989303,
53.081832297763,53.2446622895934,53.4014648709036,53.5652829780878,53.726203631189,
53.8830974752061,54.0485565057052,54.2076239213249,54.3676916335495,54.5310872191559,
54.6883648994079,54.8521973651977,55.0136084384584,55.1701810570016,55.3340506253698,
55.4936479339503,55.5770402575689),.UNSPECIFIED.);
#916=B_SPLINE_CURVE_WITH_KNOTS('',3,(#26015,#26016,#26017,#26018,#26019,
#26020,#26021,#26022,#26023,#26024,#26025,#26026,#26027,#26028,#26029,#26030,
#26031,#26032,#26033,#26034,#26035,#26036,#26037,#26038,#26039,#26040,#26041,
#26042,#26043,#26044,#26045,#26046,#26047,#26048,#26049,#26050),
 .UNSPECIFIED.,.F.,.F.,(4,2,2,2,2,2,2,2,2,2,2,2,2,2,2,2,2,4),(10.3859883446169,
10.4666739699023,10.6261726770555,10.790050887668,10.946678863482,11.1079867851551,
11.2718131320933,11.4289892727587,11.5922689727822,11.7526295968928,11.9115959323349,
12.0769359936918,12.2339397311091,12.3947517233337,12.5585825995751,12.7153077276059,
12.8780179916939,12.9862583448684),.UNSPECIFIED.);
#917=B_SPLINE_CURVE_WITH_KNOTS('',3,(#26055,#26056,#26057,#26058,#26059,
#26060,#26061,#26062,#26063,#26064,#26065,#26066,#26067,#26068,#26069,#26070,
#26071,#26072,#26073,#26074,#26075,#26076,#26077,#26078,#26079,#26080,#26081,
#26082,#26083,#26084,#26085,#26086,#26087,#26088,#26089,#26090),
 .UNSPECIFIED.,.F.,.F.,(4,2,2,2,2,2,2,2,2,2,2,2,2,2,2,2,2,4),(50.3767904783692,
50.5107812061852,50.6724906071711,50.828973545376,50.9928307396947,51.1527115480716,
51.3109574918724,51.4752705457191,51.6333495951751,51.7964642972003,51.9587226784194,
52.115238606926,52.2790758624476,52.4394709077892,52.5969192615452,52.7618026110902,
52.9203752231922,52.9768680989303),.UNSPECIFIED.);
#918=B_SPLINE_CURVE_WITH_KNOTS('',3,(#26091,#26092,#26093,#26094,#26095,
#26096,#26097,#26098,#26099,#26100,#26101,#26102,#26103,#26104,#26105,#26106,
#26107,#26108,#26109,#26110,#26111,#26112,#26113,#26114,#26115,#26116,#26117,
#26118,#26119,#26120,#26121,#26122,#26123,#26124,#26125,#26126),
 .UNSPECIFIED.,.F.,.F.,(4,2,2,2,2,2,2,2,2,2,2,2,2,2,2,2,2,4),(12.9862583448684,
13.0398334471711,13.198303057029,13.3630660757444,13.5206812995336,13.680967893734,
13.8448182265697,14.0013132076352,14.1634544438297,14.3269766650684,14.4849563935275,
14.6491542481686,14.8076151751952,14.9673935886308,15.1312638796505,15.287780569243,
15.4493815170271,15.5864597642529),.UNSPECIFIED.);
#919=B_SPLINE_CURVE_WITH_KNOTS('',3,(#26131,#26132,#26133,#26134,#26135,
#26136,#26137,#26138,#26139,#26140,#26141,#26142,#26143,#26144,#26145,#26146,
#26147,#26148,#26149,#26150,#26151,#26152,#26153,#26154,#26155,#26156,#26157,
#26158,#26159,#26160,#26161,#26162,#26163,#26164,#26165,#26166),
 .UNSPECIFIED.,.F.,.F.,(4,2,2,2,2,2,2,2,2,2,2,2,2,2,2,2,2,4),(47.7766546378743,
47.9374651673666,48.0981733406384,48.2552750339325,48.4205017209669,48.5793705970124,
48.7399906609457,48.9031593617984,49.060237346639,49.2240500153142,49.3852581718922,
49.5419351947185,49.7058122286832,49.865214957112,50.0244445853918,50.1882207786755,
50.3458320184278,50.3767904783692),.UNSPECIFIED.);
#920=B_SPLINE_CURVE_WITH_KNOTS('',3,(#26167,#26168,#26169,#26170,#26171,
#26172,#26173,#26174,#26175,#26176,#26177,#26178,#26179,#26180,#26181,#26182,
#26183,#26184,#26185,#26186,#26187,#26188,#26189,#26190,#26191,#26192,#26193,
#26194,#26195,#26196,#26197,#26198,#26199,#26200,#26201,#26202,#26203,#26204),
 .UNSPECIFIED.,.F.,.F.,(4,2,2,2,2,2,2,2,2,2,2,2,2,2,2,2,2,2,4),(15.5864597642529,
15.6132408118112,15.7707051340016,15.9343126587632,16.0939249158545,16.2531794243581,
16.4170714994651,16.5738675985109,16.7349219742824,16.8987375458885,17.0556532440191,
17.2186301669557,17.3797093851925,17.5384101242186,17.7034419351815,17.8607275155819,
18.0212576121742,18.1850918696393,18.1866042820843),.UNSPECIFIED.);
#921=B_SPLINE_CURVE_WITH_KNOTS('',3,(#26209,#26210,#26211,#26212,#26213,
#26214,#26215,#26216,#26217,#26218,#26219,#26220,#26221,#26222,#26223,#26224,
#26225,#26226,#26227,#26228,#26229,#26230,#26231,#26232,#26233,#26234,#26235,
#26236,#26237,#26238,#26239,#26240,#26241,#26242,#26243,#26244,#26245,#26246),
 .UNSPECIFIED.,.F.,.F.,(4,2,2,2,2,2,2,2,2,2,2,2,2,2,2,2,2,2,4),(45.1765418699449,
45.2008622875136,45.3647351735005,45.524417367748,45.6830642524393,45.8471544022965,
46.0050402672,46.1689154269324,46.3309469416839,46.4874256817532,46.6512786206368,
46.8114626984097,46.9692247153789,47.1338743924919,47.2922459061876,47.4543757188514,
47.6169728017918,47.7736318836056,47.7766546378743),.UNSPECIFIED.);
#922=B_SPLINE_CURVE_WITH_KNOTS('',3,(#26247,#26248,#26249,#26250,#26251,
#26252,#26253,#26254,#26255,#26256,#26257,#26258,#26259,#26260,#26261,#26262,
#26263,#26264,#26265,#26266,#26267,#26268,#26269,#26270,#26271,#26272,#26273,
#26274,#26275,#26276,#26277,#26278,#26279,#26280,#26281,#26282),
 .UNSPECIFIED.,.F.,.F.,(4,2,2,2,2,2,2,2,2,2,2,2,2,2,2,2,2,4),(18.1866042820843,
18.3416583432495,18.5040624481538,18.6667381565374,18.8249426329171,18.9894000170298,
19.1474252494328,19.3074357342038,19.4712898558371,19.6277597294378,19.7896065096557,
19.9540828346108,20.1118108083518,20.2757204293955,20.4346898301103,20.5942109922705,
20.7580850070076,20.7866467102843),.UNSPECIFIED.);
#923=B_SPLINE_CURVE_WITH_KNOTS('',3,(#26287,#26288,#26289,#26290,#26291,
#26292,#26293,#26294,#26295,#26296,#26297,#26298,#26299,#26300,#26301,#26302,
#26303,#26304,#26305,#26306,#26307,#26308,#26309,#26310,#26311,#26312,#26313,
#26314,#26315,#26316,#26317,#26318,#26319,#26320,#26321,#26322),
 .UNSPECIFIED.,.F.,.F.,(4,2,2,2,2,2,2,2,2,2,2,2,2,2,2,2,2,4),(42.5763202365159,
42.6272137044713,42.7922006287403,42.9508628372109,43.1120609046234,43.2749934789742,
43.4318737653827,43.5956919693039,43.7567061916774,43.9135330874799,44.0790936811999,
44.2382483942517,44.3981092173091,44.5616035062386,44.7189684127531,44.8828158463609,
45.0443156631371,45.1765418699449),.UNSPECIFIED.);
#924=B_SPLINE_CURVE_WITH_KNOTS('',3,(#26323,#26324,#26325,#26326,#26327,
#26328,#26329,#26330,#26331,#26332,#26333,#26334,#26335,#26336,#26337,#26338,
#26339,#26340,#26341,#26342,#26343,#26344,#26345,#26346,#26347,#26348,#26349,
#26350,#26351,#26352,#26353,#26354,#26355,#26356,#26357,#26358),
 .UNSPECIFIED.,.F.,.F.,(4,2,2,2,2,2,2,2,2,2,2,2,2,2,2,2,2,4),(20.7866467102843,
20.9146963524292,21.0760277965509,21.2398535490734,21.3970528690657,21.5603592074625,
21.7206442282256,21.879633563418,22.0450009494638,22.2019744509748,22.3628112483055,
22.5266369147414,22.6833780419026,22.8461157700061,23.0078396944665,23.1663326694566,
23.3311232209272,23.3868406765007),.UNSPECIFIED.);
#925=B_SPLINE_CURVE_WITH_KNOTS('',3,(#26363,#26364,#26365,#26366,#26367,
#26368,#26369,#26370,#26371,#26372,#26373,#26374,#26375,#26376,#26377,#26378,
#26379,#26380,#26381,#26382,#26383,#26384,#26385,#26386,#26387,#26388,#26389,
#26390,#26391,#26392,#26393,#26394,#26395,#26396,#26397,#26398),
 .UNSPECIFIED.,.F.,.F.,(4,2,2,2,2,2,2,2,2,2,2,2,2,2,2,2,2,4),(39.976181354914,
40.0548545094264,40.2187235993922,40.3764162958879,40.5410428736157,40.7028479160014,
40.8593220347091,41.0231789792917,41.183150212704,41.3412453402344,41.5056589319328,
41.6638255482828,41.8266399717696,41.9889998998425,42.1455504461389,42.3093874956531,
42.469876832279,42.5763202365159),.UNSPECIFIED.);
#926=B_SPLINE_CURVE_WITH_KNOTS('',3,(#26399,#26400,#26401,#26402,#26403,
#26404,#26405,#26406,#26407,#26408,#26409,#26410,#26411,#26412,#26413,#26414,
#26415,#26416,#26417,#26418,#26419,#26420,#26421,#26422,#26423,#26424,#26425,
#26426,#26427,#26428,#26429,#26430,#26431,#26432,#26433,#26434),
 .UNSPECIFIED.,.F.,.F.,(4,2,2,2,2,2,2,2,2,2,2,2,2,2,2,2,2,4),(23.3868406765007,
23.4886942399868,23.6490054702219,23.8128505253174,23.9693475111746,24.131515447711,
24.294934472013,24.4529365506312,24.6171605508436,24.7755657085432,24.9353671583331,
25.0992321700508,25.2557375472926,25.4173629469987,25.5826345980646,25.7401753747385,
25.9038705675823,25.9870085755541),.UNSPECIFIED.);
#927=B_SPLINE_CURVE_WITH_KNOTS('',3,(#26439,#26440,#26441,#26442,#26443,
#26444,#26445,#26446,#26447,#26448,#26449,#26450,#26451,#26452,#26453,#26454,
#26455,#26456,#26457,#26458,#26459,#26460,#26461,#26462,#26463,#26464,#26465,
#26466,#26467,#26468,#26469,#26470,#26471,#26472,#26473,#26474),
 .UNSPECIFIED.,.F.,.F.,(4,2,2,2,2,2,2,2,2,2,2,2,2,2,2,2,2,4),(37.3759376529246,
37.4845427362404,37.6472373015768,37.8039522835337,37.9677822299911,38.1285797555106,
38.2855942839381,38.4509186393567,38.6098713537324,38.7702632861893,38.9335276219079,
39.0906900865903,39.2545134241937,39.4158074320668,39.572440014719,39.7363168360909,
39.8958021421056,39.976181354914),.UNSPECIFIED.);
#928=B_SPLINE_CURVE_WITH_KNOTS('',3,(#26475,#26476,#26477,#26478,#26479,
#26480,#26481,#26482,#26483,#26484,#26485,#26486,#26487,#26488,#26489,#26490,
#26491,#26492,#26493,#26494,#26495,#26496,#26497,#26498,#26499,#26500,#26501,
#26502,#26503,#26504,#26505,#26506,#26507,#26508,#26509,#26510),
 .UNSPECIFIED.,.F.,.F.,(4,2,2,2,2,2,2,2,2,2,2,2,2,2,2,2,2,4),(25.9870085755541,
26.0632825128444,26.2226140300249,26.3864988483248,26.5432310331721,26.7043651749984,
26.8681708361658,27.0251614375154,27.1882270747621,27.3490576030318,27.5078350894429,
27.6729569285989,27.8301355116954,27.9907472073234,28.1545711733677,28.311172302475,
28.4736653813112,28.5871150949191),.UNSPECIFIED.);
#929=B_SPLINE_CURVE_WITH_KNOTS('',3,(#26515,#26516,#26517,#26518,#26519,
#26520,#26521,#26522,#26523,#26524,#26525,#26526,#26527,#26528,#26529,#26530,
#26531,#26532,#26533,#26534,#26535,#26536,#26537,#26538,#26539,#26540,#26541,
#26542,#26543,#26544,#26545,#26546,#26547,#26548,#26549,#26550),
 .UNSPECIFIED.,.F.,.F.,(4,2,2,2,2,2,2,2,2,2,2,2,2,2,2,2,2,4),(34.7757588841055,
34.9131766642864,35.0747633517156,35.2312822366005,35.3951516261494,35.5549164450714,
35.7133996037316,35.8775823658074,36.0355488361476,36.1991146383398,36.3612405616305,
36.5177317480541,36.68158117977,36.8418534210273,36.9994857262212,37.1642329854863,
37.3226888436329,37.3759376529246),.UNSPECIFIED.);
#930=B_SPLINE_CURVE_WITH_KNOTS('',3,(#26551,#26552,#26553,#26554,#26555,
#26556,#26557,#26558,#26559,#26560,#26561,#26562,#26563,#26564,#26565,#26566,
#26567,#26568,#26569,#26570,#26571,#26572,#26573,#26574,#26575,#26576,#26577,
#26578,#26579,#26580,#26581,#26582,#26583,#26584,#26585,#26586),
 .UNSPECIFIED.,.F.,.F.,(4,2,2,2,2,2,2,2,2,2,2,2,2,2,2,2,2,4),(28.5871150949191,
28.6360488595124,28.7943292099721,28.9588749397764,29.1167530356116,29.2768424992895,
29.4406862391693,29.5971479886017,29.7590791830785,29.9232364301957,30.0810353144069,
30.2450269438081,30.4038198713806,30.5634133135096,30.7272769768795,30.883843214224,
31.0452504411699,31.1870971694932),.UNSPECIFIED.);
#931=B_SPLINE_CURVE_WITH_KNOTS('',3,(#26591,#26592,#26593,#26594,#26595,
#26596,#26597,#26598,#26599,#26600,#26601,#26602,#26603,#26604,#26605,#26606,
#26607,#26608,#26609,#26610,#26611,#26612,#26613,#26614,#26615,#26616,#26617,
#26618,#26619,#26620,#26621,#26622,#26623,#26624,#26625,#26626,#26627,#26628),
 .UNSPECIFIED.,.F.,.F.,(4,2,2,2,2,2,2,2,2,2,2,2,2,2,2,2,2,2,4),(32.175633435784,
32.1775107813409,32.3413446580404,32.501860016056,32.6591611046315,32.8241767832933,
32.9828635414385,33.1439805221191,33.3069415147973,33.4638441163799,33.6276592531707,
33.7886991048983,33.9455039498272,34.1093951733975,34.2686355916604,34.4282781528139,
34.5918698348922,34.7493201518321,34.7757588841055),.UNSPECIFIED.);
#932=B_SPLINE_CURVE_WITH_KNOTS('',3,(#26629,#26630,#26631,#26632,#26633,
#26634,#26635,#26636,#26637,#26638,#26639,#26640,#26641,#26642,#26643,#26644,
#26645,#26646,#26647,#26648,#26649,#26650,#26651,#26652,#26653,#26654,#26655,
#26656,#26657,#26658,#26659,#26660,#26661,#26662,#26663,#26664,#26665,#26666),
 .UNSPECIFIED.,.F.,.F.,(4,2,2,2,2,2,2,2,2,2,2,2,2,2,2,2,2,2,4),(31.1870971694932,
31.2090772686752,31.3663512188482,31.5297431143764,31.6898001409927,31.8488637597776,
32.0143190871344,32.1712055862005,32.3321225158812,32.4959346463123,32.6527332075193,
32.814331120641,32.970833571967,33.1346911409304,33.294466191355,33.4528984815721,
33.6170936754505,33.7750699448881,33.787031069066),.UNSPECIFIED.);
#933=B_SPLINE_CURVE_WITH_KNOTS('',3,(#26671,#26672,#26673,#26674,#26675,
#26676,#26677,#26678,#26679,#26680,#26681,#26682,#26683,#26684,#26685,#26686,
#26687,#26688,#26689,#26690,#26691,#26692,#26693,#26694,#26695,#26696,#26697,
#26698,#26699,#26700,#26701,#26702,#26703,#26704,#26705,#26706),
 .UNSPECIFIED.,.F.,.F.,(4,2,2,2,2,2,2,2,2,2,2,2,2,2,2,2,2,4),(29.5756035802014,
29.6045003448811,29.7683739842147,29.9278820022522,30.0868774516155,30.2507723498575,
30.4084873914971,30.5730119648943,30.7348436465841,30.8913135094951,31.0551672611946,
31.2151634914049,31.3732104004737,31.537651997735,31.6958427008405,31.8585627767629,
32.0209509921586,32.175633435784),.UNSPECIFIED.);
#934=B_SPLINE_CURVE_WITH_KNOTS('',3,(#26707,#26708,#26709,#26710,#26711,
#26712,#26713,#26714,#26715,#26716,#26717,#26718,#26719,#26720,#26721,#26722,
#26723,#26724,#26725,#26726,#26727,#26728,#26729,#26730,#26731,#26732,#26733,
#26734,#26735,#26736,#26737,#26738,#26739,#26740,#26741,#26742),
 .UNSPECIFIED.,.F.,.F.,(4,2,2,2,2,2,2,2,2,2,2,2,2,2,2,2,2,4),(33.787031069066,
33.9385479563215,34.1006868518737,34.2571718625092,34.42100947491,34.5812931938916,
34.7388835311519,34.9036443059465,35.0621107580024,35.2238858328536,35.3865939729145,
35.5433136155739,35.7071317939495,35.8679409387723,36.0249243123382,36.1902620337357,
36.3492250687649,36.3870506062284),.UNSPECIFIED.);
#935=B_SPLINE_CURVE_WITH_KNOTS('',3,(#26747,#26748,#26749,#26750,#26751,
#26752,#26753,#26754,#26755,#26756,#26757,#26758,#26759,#26760,#26761,#26762,
#26763,#26764,#26765,#26766,#26767,#26768,#26769,#26770,#26771,#26772,#26773,
#26774,#26775,#26776,#26777,#26778,#26779,#26780,#26781,#26782),
 .UNSPECIFIED.,.F.,.F.,(4,2,2,2,2,2,2,2,2,2,2,2,2,2,2,2,2,4),(26.9754188903882,
27.0315113171753,27.1962861825211,27.3547655743049,27.5165311558328,27.6792532653912,
27.8359842958766,27.9998100765242,28.1606325684036,28.3176182504787,28.4829700532874,
28.6419459835266,28.8022649856762,28.9655561057364,29.1227419640259,29.2865656025431,
29.4478833589509,29.5756035802014),.UNSPECIFIED.);
#936=B_SPLINE_CURVE_WITH_KNOTS('',3,(#26783,#26784,#26785,#26786,#26787,
#26788,#26789,#26790,#26791,#26792,#26793,#26794,#26795,#26796,#26797,#26798,
#26799,#26800,#26801,#26802,#26803,#26804,#26805,#26806,#26807,#26808,#26809,
#26810,#26811,#26812,#26813,#26814,#26815,#26816,#26817,#26818),
 .UNSPECIFIED.,.F.,.F.,(4,2,2,2,2,2,2,2,2,2,2,2,2,2,2,2,2,4),(36.3870506062284,
36.5095505106562,36.6728277922848,36.8300008138566,36.9938159430349,37.1551205776933,
37.3117325973914,37.4755984325684,37.6350936337405,37.7940923476327,37.957973577995,
38.1156759713782,38.2802126316001,38.4420305861104,38.5984931880261,38.7623391387606,
38.9223220705895,38.9870541035935),.UNSPECIFIED.);
#937=B_SPLINE_CURVE_WITH_KNOTS('',3,(#26823,#26824,#26825,#26826,#26827,
#26828,#26829,#26830,#26831,#26832,#26833,#26834,#26835,#26836,#26837,#26838,
#26839,#26840,#26841,#26842,#26843,#26844,#26845,#26846,#26847,#26848,#26849,
#26850,#26851,#26852,#26853,#26854,#26855,#26856,#26857,#26858),
 .UNSPECIFIED.,.F.,.F.,(4,2,2,2,2,2,2,2,2,2,2,2,2,2,2,2,2,4),(24.3752567166036,
24.4565959364233,24.6172359201442,24.781068110726,24.9376878811401,25.1002110361017,
25.2625412882476,25.4208485741219,25.5854244165739,25.743280986078,25.9033982265957,
26.0672501674617,26.2237210788033,26.3856814121459,26.5497791793857,26.7136243818014,
26.8739213856385,26.9754188903882),.UNSPECIFIED.);
#938=B_SPLINE_CURVE_WITH_KNOTS('',3,(#26859,#26860,#26861,#26862,#26863,
#26864,#26865,#26866,#26867,#26868,#26869,#26870,#26871,#26872,#26873,#26874,
#26875,#26876,#26877,#26878,#26879,#26880,#26881,#26882,#26883,#26884,#26885,
#26886,#26887,#26888,#26889,#26890,#26891,#26892,#26893,#26894),
 .UNSPECIFIED.,.F.,.F.,(4,2,2,2,2,2,2,2,2,2,2,2,2,2,2,2,2,4),(38.9870541035935,
39.0803705159472,39.2447979793195,39.4029756632131,39.5657063457729,39.7280804788507,
39.8846302741835,40.0484563466386,40.2089581787015,40.3662583228638,40.5312596936028,
40.6899333193432,40.8510582940319,41.014005155137,41.1708951149417,41.3347024266529,
41.495728810533,41.5870777147423),.UNSPECIFIED.);
#939=B_SPLINE_CURVE_WITH_KNOTS('',3,(#26899,#26900,#26901,#26902,#26903,
#26904,#26905,#26906,#26907,#26908,#26909,#26910,#26911,#26912,#26913,#26914,
#26915,#26916,#26917,#26918,#26919,#26920,#26921,#26922,#26923,#26924,#26925,
#26926,#26927,#26928,#26929,#26930,#26931,#26932,#26933,#26934),
 .UNSPECIFIED.,.F.,.F.,(4,2,2,2,2,2,2,2,2,2,2,2,2,2,2,2,2,4),(21.7751553262989,
21.8822756137629,22.0439113791663,22.2090980146475,22.3666462235154,22.5303509413377,
22.6897109077896,22.8490499085509,23.012923595653,23.1696335579083,23.3307757123397,
23.4945773891925,23.6515904448586,23.8146860274203,23.9754731163525,24.1342776665709,
24.2994299151046,24.3752567166036),.UNSPECIFIED.);
#940=B_SPLINE_CURVE_WITH_KNOTS('',3,(#26935,#26936,#26937,#26938,#26939,
#26940,#26941,#26942,#26943,#26944,#26945,#26946,#26947,#26948,#26949,#26950,
#26951,#26952,#26953,#26954,#26955,#26956,#26957,#26958,#26959,#26960,#26961,
#26962,#26963,#26964,#26965,#26966,#26967,#26968,#26969,#26970),
 .UNSPECIFIED.,.F.,.F.,(4,2,2,2,2,2,2,2,2,2,2,2,2,2,2,2,2,4),(41.5870777147423,
41.6525299655238,41.8164131898957,41.9756404002719,42.1352879802968,42.298865531762,
42.4563027572898,42.6201504819589,42.7817237805508,42.9382363008472,43.1020976718053,
43.2618494583129,43.4203343808643,43.5845032887473,43.7424569469071,43.9060330407087,
44.0681451134247,44.1871553710452),.UNSPECIFIED.);
#941=B_SPLINE_CURVE_WITH_KNOTS('',3,(#26975,#26976,#26977,#26978,#26979,
#26980,#26981,#26982,#26983,#26984,#26985,#26986,#26987,#26988,#26989,#26990,
#26991,#26992,#26993,#26994,#26995,#26996,#26997,#26998,#26999,#27000,#27001,
#27002,#27003,#27004,#27005,#27006,#27007,#27008,#27009,#27010),
 .UNSPECIFIED.,.F.,.F.,(4,2,2,2,2,2,2,2,2,2,2,2,2,2,2,2,2,4),(19.1751960155601,
19.3101100041855,19.4728601071602,19.6345116693977,19.7930142851345,19.957817190375,
20.1153499099463,20.2756716296436,20.4395055506287,20.595997428871,20.7581772725523,
20.9215153105913,21.0795263704231,21.2437618078274,21.4021202185422,21.5619310799127,
21.725784954197,21.7751553262989),.UNSPECIFIED.);
#942=B_SPLINE_CURVE_WITH_KNOTS('',3,(#27011,#27012,#27013,#27014,#27015,
#27016,#27017,#27018,#27019,#27020,#27021,#27022,#27023,#27024,#27025,#27026,
#27027,#27028,#27029,#27030,#27031,#27032,#27033,#27034,#27035,#27036,#27037,
#27038,#27039,#27040,#27041,#27042,#27043,#27044,#27045,#27046),
 .UNSPECIFIED.,.F.,.F.,(4,2,2,2,2,2,2,2,2,2,2,2,2,2,2,2,2,4),(44.1871553710452,
44.2246274834992,44.3884688978133,44.5487277671559,44.7063597731386,44.8710928730091,
45.0295356890391,45.1913978592965,45.3540783838714,45.5107819285521,45.6746038470453,
45.835387924594,45.9923996031062,46.1577097889147,46.3166494871573,46.4770468473187,
46.6402972479939,46.7872229415117),.UNSPECIFIED.);
#943=B_SPLINE_CURVE_WITH_KNOTS('',3,(#27051,#27052,#27053,#27054,#27055,
#27056,#27057,#27058,#27059,#27060,#27061,#27062,#27063,#27064,#27065,#27066,
#27067,#27068,#27069,#27070,#27071,#27072,#27073,#27074,#27075,#27076,#27077,
#27078,#27079,#27080,#27081,#27082,#27083,#27084,#27085,#27086,#27087,#27088),
 .UNSPECIFIED.,.F.,.F.,(4,2,2,2,2,2,2,2,2,2,2,2,2,2,2,2,2,2,4),(16.5752364738999,
16.5809043992186,16.738641033749,16.9025615621065,17.0614820445148,17.2210120734106,
17.384875732046,17.5414685495772,17.7028095566869,17.8666275515996,18.0238363732713,
18.1871544175959,18.3473786463044,18.5063772919755,18.6717568025283,18.8287020750767,
18.989549409536,19.1533639946529,19.1751960155601),.UNSPECIFIED.);
#944=B_SPLINE_CURVE_WITH_KNOTS('',3,(#27089,#27090,#27091,#27092,#27093,
#27094,#27095,#27096,#27097,#27098,#27099,#27100,#27101,#27102,#27103,#27104,
#27105,#27106,#27107,#27108,#27109,#27110,#27111,#27112,#27113,#27114,#27115,
#27116,#27117,#27118,#27119,#27120,#27121,#27122,#27123,#27124,#27125,#27126),
 .UNSPECIFIED.,.F.,.F.,(4,2,2,2,2,2,2,2,2,2,2,2,2,2,2,2,2,2,4),(46.7872229415117,
46.7974467558072,46.9612612134908,47.1225419740756,47.279169178961,47.4430377815618,
47.6025101340063,47.7615649335297,47.9254202372429,48.083100144397,48.2477375280673,
48.4095287324009,48.5659953165688,48.7298440455678,48.8898018523219,49.0478978172873,
49.2122971621086,49.370450620887,49.3871486091453),.UNSPECIFIED.);
#945=B_SPLINE_CURVE_WITH_KNOTS('',3,(#27131,#27132,#27133,#27134,#27135,
#27136,#27137,#27138,#27139,#27140,#27141,#27142,#27143,#27144,#27145,#27146,
#27147,#27148,#27149,#27150,#27151,#27152,#27153,#27154,#27155,#27156,#27157,
#27158,#27159,#27160,#27161,#27162,#27163,#27164,#27165,#27166),
 .UNSPECIFIED.,.F.,.F.,(4,2,2,2,2,2,2,2,2,2,2,2,2,2,2,2,2,4),(13.9753192948077,
14.0067045743461,14.1654153988763,14.3304600567658,14.4877125732657,14.6482537657069,
14.8120776792938,14.9686439321478,15.1310607227353,15.2936603060804,15.4518746263024,
15.6163444221346,15.7743273673789,15.9343483004934,16.098192059448,16.2546518382711,
16.4165102067085,16.5752364738999),.UNSPECIFIED.);
#946=B_SPLINE_CURVE_WITH_KNOTS('',3,(#27167,#27168,#27169,#27170,#27171,
#27172,#27173,#27174,#27175,#27176,#27177,#27178,#27179,#27180,#27181,#27182,
#27183,#27184,#27185,#27186,#27187,#27188,#27189,#27190,#27191,#27192,#27193,
#27194,#27195,#27196,#27197,#27198,#27199,#27200,#27201,#27202),
 .UNSPECIFIED.,.F.,.F.,(4,2,2,2,2,2,2,2,2,2,2,2,2,2,2,2,2,4),(49.3871486091453,
49.5332745128823,49.6956202467741,49.8521606598271,50.0159894913195,50.1764651674857,
50.3338005374518,50.4987730301628,50.6574219569031,50.8186270526262,50.9815453671276,
51.138412973096,51.3022229403195,51.4632235408708,51.6200463160427,51.7855925924826,
51.9447341554513,51.9871887418935),.UNSPECIFIED.);
#947=B_SPLINE_CURVE_WITH_KNOTS('',3,(#27207,#27208,#27209,#27210,#27211,
#27212,#27213,#27214,#27215,#27216,#27217,#27218,#27219,#27220,#27221,#27222,
#27223,#27224,#27225,#27226,#27227,#27228,#27229,#27230,#27231,#27232,#27233,
#27234,#27235,#27236,#27237,#27238,#27239,#27240,#27241,#27242),
 .UNSPECIFIED.,.F.,.F.,(4,2,2,2,2,2,2,2,2,2,2,2,2,2,2,2,2,4),(11.3752281506608,
11.4331440082726,11.5928714158197,11.7567340594759,11.9132545003004,12.074802135132,
12.2403347218686,12.3978092052149,12.561429194959,12.7209864699398,12.8802511578905,
13.0441335836658,13.2009066387116,13.3619717253299,13.525777036828,13.6827019191146,
13.8456915128137,13.9753192948077),.UNSPECIFIED.);
#948=B_SPLINE_CURVE_WITH_KNOTS('',3,(#27243,#27244,#27245,#27246,#27247,
#27248,#27249,#27250,#27251,#27252,#27253,#27254,#27255,#27256,#27257,#27258,
#27259,#27260,#27261,#27262,#27263,#27264,#27265,#27266,#27267,#27268,#27269,
#27270,#27271,#27272,#27273,#27274,#27275,#27276,#27277,#27278),
 .UNSPECIFIED.,.F.,.F.,(4,2,2,2,2,2,2,2,2,2,2,2,2,2,2,2,2,4),(51.9871887418935,
52.1045989553424,52.2680792084208,52.4254310665492,52.5892693766665,52.7507558469993,
52.9072959719357,53.0711604271069,53.2308295999598,53.3894774879068,53.5535538206852,
53.7114268637422,53.8753109335028,54.037328629624,54.193798648683,54.3576431588387,
54.5178138567586,54.5872639586609),.UNSPECIFIED.);
#949=B_SPLINE_CURVE_WITH_KNOTS('',3,(#27283,#27284,#27285,#27286,#27287,
#27288,#27289,#27290,#27291,#27292,#27293,#27294,#27295,#27296,#27297,#27298,
#27299,#27300,#27301,#27302,#27303,#27304,#27305,#27306,#27307,#27308,#27309,
#27310,#27311,#27312,#27313,#27314,#27315,#27316,#27317,#27318),
 .UNSPECIFIED.,.F.,.F.,(4,2,2,2,2,2,2,2,2,2,2,2,2,2,2,2,2,4),(8.77513878253031,
8.85957795966849,9.02033579080828,9.1841589294471,9.34084550443931,9.50349734972825,
9.66544094625724,9.82385895709363,9.98856332188794,10.1462334324883,10.3064663402911,
10.4703090291096,10.626787297808,10.7888715304564,10.9525392357421,11.1104691365834,
11.2746107142529,11.3752281506608),.UNSPECIFIED.);
#950=B_SPLINE_CURVE_WITH_KNOTS('',3,(#27319,#27320,#27321,#27322,#27323,
#27324,#27325,#27326,#27327,#27328,#27329,#27330,#27331,#27332,#27333,#27334,
#27335,#27336,#27337,#27338,#27339,#27340,#27341,#27342,#27343,#27344,#27345,
#27346,#27347,#27348,#27349,#27350,#27351,#27352,#27353,#27354),
 .UNSPECIFIED.,.F.,.F.,(4,2,2,2,2,2,2,2,2,2,2,2,2,2,2,2,2,4),(54.5872639586609,
54.6755750711845,54.8402105986611,54.9985690338287,55.1607060588628,55.3232890958237,
55.4799369962627,55.6437618441001,55.8044565200012,55.9615550736393,56.1267675505751,
56.285623328814,56.4462480452348,56.6094027495969,56.7664676863386,56.9302711419498,
57.0914659561543,57.1873615863288),.UNSPECIFIED.);
#951=B_SPLINE_CURVE_WITH_KNOTS('',3,(#27359,#27360,#27361,#27362,#27363,
#27364,#27365,#27366,#27367,#27368,#27369,#27370,#27371,#27372,#27373,#27374,
#27375,#27376,#27377,#27378,#27379,#27380,#27381,#27382,#27383,#27384,#27385,
#27386,#27387,#27388,#27389,#27390,#27391,#27392,#27393,#27394),
 .UNSPECIFIED.,.F.,.F.,(4,2,2,2,2,2,2,2,2,2,2,2,2,2,2,2,2,4),(6.17506899243254,
6.28542206375772,6.44718527831052,6.61191749423575,6.76957357592004,6.93340167664995,
7.09250849583087,7.25195667231655,7.41582556755354,7.57246560060843,7.7337211992204,
7.897532695118,8.05465744283474,8.21787978367144,8.37834425273139,8.537259359205,
8.70254085846295,8.77513878253031),.UNSPECIFIED.);
#952=B_SPLINE_CURVE_WITH_KNOTS('',3,(#27395,#27396,#27397,#27398,#27399,
#27400,#27401,#27402,#27403,#27404,#27405,#27406,#27407,#27408,#27409,#27410,
#27411,#27412,#27413,#27414,#27415,#27416,#27417,#27418,#27419,#27420,#27421,
#27422,#27423,#27424,#27425,#27426,#27427,#27428,#27429,#27430),
 .UNSPECIFIED.,.F.,.F.,(4,2,2,2,2,2,2,2,2,2,2,2,2,2,2,2,2,4),(57.1873615863288,
57.2481374311781,57.412005851322,57.5713955105336,57.7306270023818,57.8943893060583,
58.051987626823,58.2169466622617,58.3786421174995,58.5351175364027,58.6989661200439,
58.8588333669063,59.0170797936999,59.1813784709152,59.3394442077022,59.50256768913,
59.6648117339904,59.7873029751542),.UNSPECIFIED.);
#953=B_SPLINE_CURVE_WITH_KNOTS('',3,(#27435,#27436,#27437,#27438,#27439,
#27440,#27441,#27442,#27443,#27444,#27445,#27446,#27447,#27448,#27449,#27450,
#27451,#27452,#27453,#27454,#27455,#27456,#27457,#27458,#27459,#27460,#27461,
#27462,#27463,#27464,#27465,#27466,#27467,#27468,#27469,#27470),
 .UNSPECIFIED.,.F.,.F.,(4,2,2,2,2,2,2,2,2,2,2,2,2,2,2,2,2,4),(3.57510705038708,
3.71339809964079,3.87628653037861,4.03756721491112,4.19619004676284,4.36113233712773,
4.5185000268825,4.67894820506975,4.84277732466363,4.99930711704217,5.16162319475703,
5.32453503301027,5.48266292720209,5.64703288620151,5.8051728690298,5.9651042464861,
6.1289532790101,6.17506899243254),.UNSPECIFIED.);
#954=B_SPLINE_CURVE_WITH_KNOTS('',3,(#27471,#27472,#27473,#27474,#27475,
#27476,#27477,#27478,#27479,#27480,#27481,#27482,#27483,#27484,#27485,#27486,
#27487,#27488,#27489,#27490,#27491,#27492,#27493,#27494,#27495,#27496,#27497,
#27498,#27499,#27500,#27501,#27502,#27503,#27504,#27505,#27506),
 .UNSPECIFIED.,.F.,.F.,(4,2,2,2,2,2,2,2,2,2,2,2,2,2,2,2,2,4),(59.7873029751542,
59.8213176769373,59.9851463211867,60.1455275333865,60.3029742107817,60.4678429536221,
60.6264020880418,60.7878657484224,60.9506812879062,61.107471377028,61.2712808583781,
61.4321876678488,61.5890773203166,61.7545218029967,61.913575824595,62.0736472442929,
62.2370285455998,62.3872680920556),.UNSPECIFIED.);
#955=B_SPLINE_CURVE_WITH_KNOTS('',3,(#27512,#27513,#27514,#27515,#27516,
#27517,#27518,#27519),.UNSPECIFIED.,.F.,.F.,(4,2,2,4),(64.9871389669336,
65.1296711980224,65.2172690762215,65.3048855506376),.UNSPECIFIED.);
#956=B_SPLINE_CURVE_WITH_KNOTS('',3,(#27522,#27523,#27524,#27525,#27526,
#27527,#27528,#27529,#27530,#27531,#27532,#27533,#27534,#27535,#27536,#27537),
 .UNSPECIFIED.,.F.,.F.,(4,2,2,2,2,2,2,4),(0.,0.0888555353420051,0.177236701399272,
0.337381099353558,0.501224862287476,0.657691166279862,0.819680858070591,
0.975100065405521),.UNSPECIFIED.);
#957=B_SPLINE_CURVE_WITH_KNOTS('',3,(#27550,#27551,#27552,#27553,#27554,
#27555,#27556,#27557,#27558,#27559,#27560,#27561,#27562,#27563,#27564,#27565,
#27566,#27567,#27568,#27569,#27570,#27571,#27572,#27573,#27574,#27575,#27576,
#27577,#27578,#27579,#27580,#27581,#27582,#27583),.UNSPECIFIED.,.F.,.F.,
(4,2,2,2,2,2,2,2,2,2,2,2,2,2,2,2,4),(0.,0.0200190791396383,0.0342447058880318,
0.0622704019494858,0.138479246631928,0.207804595812129,0.31343546609501,
0.445646771066455,0.604311883207654,0.806831895759981,1.16880638589577,
1.2714352086145,1.35107618267665,1.37963884460666,1.40478661373671,1.44768560678447,
1.58331119056091),.UNSPECIFIED.);
#958=B_SPLINE_CURVE_WITH_KNOTS('',3,(#27592,#27593,#27594,#27595,#27596,
#27597,#27598,#27599,#27600,#27601,#27602,#27603,#27604,#27605,#27606,#27607,
#27608,#27609,#27610,#27611,#27612,#27613,#27614,#27615,#27616,#27617,#27618,
#27619,#27620,#27621,#27622,#27623,#27624,#27625),.UNSPECIFIED.,.F.,.F.,
(4,2,2,2,2,2,2,2,2,2,2,2,2,2,2,2,4),(0.,0.0200190791268279,0.0342447058137099,
0.062270401610795,0.138479245078895,0.207804592960761,0.313435460954431,
0.445646763082409,0.604311871816074,0.806831880422644,1.168806362678,1.27143518292978,
1.35107615505061,1.37963881630498,1.40478658485205,1.44768557691437,1.58331115935392),
 .UNSPECIFIED.);
#959=B_SPLINE_CURVE_WITH_KNOTS('',3,(#27641,#27642,#27643,#27644,#27645,
#27646,#27647,#27648,#27649,#27650,#27651,#27652,#27653,#27654,#27655,#27656,
#27657,#27658,#27659,#27660,#27661,#27662,#27663,#27664,#27665,#27666,#27667,
#27668,#27669,#27670,#27671,#27672,#27673,#27674,#27675,#27676,#27677,#27678,
#27679,#27680,#27681,#27682,#27683,#27684,#27685,#27686,#27687,#27688,#27689,
#27690,#27691,#27692,#27693,#27694,#27695,#27696,#27697,#27698,#27699,#27700,
#27701,#27702,#27703,#27704,#27705,#27706,#27707,#27708,#27709,#27710,#27711,
#27712,#27713,#27714,#27715,#27716,#27717,#27718,#27719,#27720,#27721,#27722,
#27723,#27724,#27725,#27726,#27727,#27728,#27729,#27730,#27731,#27732,#27733,
#27734,#27735,#27736,#27737,#27738,#27739,#27740,#27741,#27742,#27743,#27744,
#27745,#27746,#27747,#27748,#27749,#27750,#27751,#27752,#27753,#27754,#27755,
#27756,#27757,#27758,#27759,#27760,#27761,#27762,#27763,#27764,#27765,#27766,
#27767,#27768,#27769,#27770,#27771,#27772,#27773,#27774,#27775,#27776,#27777,
#27778,#27779,#27780,#27781,#27782,#27783,#27784,#27785,#27786,#27787,#27788,
#27789,#27790,#27791,#27792,#27793,#27794,#27795,#27796,#27797,#27798,#27799,
#27800,#27801,#27802,#27803,#27804,#27805,#27806,#27807,#27808,#27809,#27810,
#27811,#27812),.UNSPECIFIED.,.F.,.F.,(4,3,3,3,3,3,3,3,3,3,3,3,3,3,3,3,3,
3,3,3,3,3,3,3,3,3,3,3,3,3,3,3,3,3,3,3,3,3,3,3,3,3,3,3,3,3,3,3,3,3,3,3,3,
3,3,3,3,4),(0.,0.0123304528366813,0.015625,0.0234375,0.02734375,0.0301056900711975,
0.03125,0.046875,0.0546875,0.0594470156310227,0.0625,0.075247186070732,
0.088385422654067,0.09375,0.107364232132532,0.121140761267218,0.125,0.147800625991517,
0.171014013031671,0.1875,0.21875,0.25,0.291221604078999,0.330354604152427,
0.367655777317147,0.402706302973929,0.436731165753159,0.469340412865769,
0.5,0.532623098826544,0.565615945128827,0.599234685440434,0.625,0.66623935755091,
0.713840887684498,0.75,0.7738913879151,0.796705025179732,0.8125,0.84375,
0.857899936485349,0.871788138789888,0.875,0.888569347832588,0.902293044929379,
0.90625,0.921875,0.9296875,0.934420440289022,0.9375,0.953125,0.9609375,
0.96484375,0.967460263406796,0.96875,0.981091439099429,0.993421435631299,
1.),.UNSPECIFIED.);
#960=B_SPLINE_CURVE_WITH_KNOTS('',3,(#27819,#27820,#27821,#27822,#27823,
#27824,#27825,#27826,#27827,#27828,#27829,#27830,#27831,#27832,#27833,#27834,
#27835,#27836,#27837,#27838,#27839,#27840,#27841,#27842,#27843,#27844,#27845,
#27846,#27847,#27848,#27849,#27850,#27851,#27852,#27853,#27854,#27855,#27856,
#27857,#27858,#27859,#27860,#27861,#27862,#27863,#27864,#27865,#27866,#27867,
#27868,#27869,#27870,#27871,#27872,#27873,#27874,#27875,#27876,#27877,#27878,
#27879,#27880,#27881,#27882,#27883,#27884,#27885,#27886,#27887,#27888,#27889,
#27890,#27891,#27892,#27893,#27894,#27895,#27896,#27897,#27898,#27899,#27900,
#27901,#27902,#27903,#27904,#27905,#27906,#27907,#27908,#27909,#27910,#27911,
#27912,#27913,#27914,#27915,#27916,#27917,#27918,#27919,#27920,#27921,#27922,
#27923,#27924,#27925,#27926,#27927,#27928,#27929,#27930,#27931,#27932,#27933,
#27934,#27935,#27936,#27937,#27938,#27939,#27940,#27941,#27942,#27943,#27944,
#27945,#27946,#27947,#27948,#27949,#27950,#27951,#27952,#27953,#27954,#27955,
#27956,#27957,#27958,#27959,#27960,#27961,#27962,#27963,#27964,#27965,#27966,
#27967,#27968,#27969,#27970,#27971,#27972,#27973,#27974,#27975,#27976,#27977,
#27978,#27979,#27980,#27981,#27982,#27983,#27984,#27985,#27986,#27987,#27988,
#27989,#27990),.UNSPECIFIED.,.F.,.F.,(4,3,3,3,3,3,3,3,3,3,3,3,3,3,3,3,3,
3,3,3,3,3,3,3,3,3,3,3,3,3,3,3,3,3,3,3,3,3,3,3,3,3,3,3,3,3,3,3,3,3,3,3,3,
3,3,3,3,4),(0.,0.0123304529175167,0.015625,0.0234375,0.02734375,0.0301056900816795,
0.03125,0.0520631268126456,0.0546875,0.0594470156580883,0.0625,0.0752471860780028,
0.0883854226637524,0.09375,0.107364232235248,0.121140761476458,0.125,0.147800626053147,
0.171014013162799,0.1875,0.21875,0.25,0.291221604248134,0.33035460442656,
0.367655777650242,0.402706303325056,0.436731166106891,0.469340413207235,
0.5,0.532623098825363,0.565615945123432,0.599234685425392,0.625,0.666239357866276,
0.713840888882716,0.75,0.773891388313745,0.796705025965584,0.8125,0.84375,
0.857899936516628,0.871788138848581,0.875,0.888569347967903,0.902293045202129,
0.90625,0.921875,0.9296875,0.934420440304062,0.9375,0.953125,0.9609375,
0.96484375,0.967460263411401,0.96875,0.981091439135241,0.993421435702746,
1.),.UNSPECIFIED.);
#961=B_SPLINE_CURVE_WITH_KNOTS('',3,(#28009,#28010,#28011,#28012,#28013,
#28014,#28015,#28016,#28017,#28018,#28019,#28020,#28021,#28022,#28023,#28024,
#28025,#28026,#28027,#28028,#28029,#28030,#28031,#28032,#28033,#28034,#28035,
#28036,#28037,#28038,#28039,#28040,#28041,#28042,#28043,#28044,#28045,#28046),
 .UNSPECIFIED.,.F.,.F.,(4,2,2,2,2,2,2,2,2,2,2,2,2,2,2,2,2,2,4),(0.975100065405521,
0.983650720032818,1.14149968175405,1.30554854967722,1.4642415654359,1.6238861288094,
1.78774983079492,1.944297258767,2.10575797334962,2.26959209753089,2.42691864100778,
2.59037021955754,2.75029520673997,2.90941141310176,3.0749281527528,3.23177015259627,
3.39274353675959,3.5565536980093,3.57510705038708),.UNSPECIFIED.);
#962=B_SPLINE_CURVE_WITH_KNOTS('',3,(#28047,#28048,#28049,#28050,#28051,
#28052,#28053,#28054,#28055,#28056,#28057,#28058,#28059,#28060,#28061,#28062,
#28063,#28064,#28065,#28066,#28067,#28068,#28069,#28070,#28071,#28072,#28073,
#28074,#28075,#28076,#28077,#28078,#28079,#28080,#28081,#28082,#28083,#28084),
 .UNSPECIFIED.,.F.,.F.,(4,2,2,2,2,2,2,2,2,2,2,2,2,2,2,2,2,2,4),(62.3872680920556,
62.3942929217837,62.5581159138936,62.7195133790498,62.8760794400901,63.0399401958598,
63.1995242071887,63.3583274114545,63.5223087369075,63.6800983500538,63.8442771207718,
64.0061978767224,64.1626564560649,64.3264972909694,64.4865768024129,64.6444627786545,
64.8089977143487,64.9672684116498,64.9871389669336),.UNSPECIFIED.);
#963=B_SPLINE_CURVE_WITH_KNOTS('',3,(#28086,#28087,#28088,#28089,#28090,
#28091,#28092,#28093,#28094,#28095,#28096,#28097,#28098,#28099),
 .UNSPECIFIED.,.F.,.F.,(4,2,2,2,2,2,4),(-0.787689357170944,-0.679879919295326,
-0.568513455580561,-0.412331745472765,-0.251692020866062,-0.13048064500736,
0.),.UNSPECIFIED.);
#964=B_SPLINE_CURVE_WITH_KNOTS('',3,(#28100,#28101,#28102,#28103,#28104,
#28105,#28106,#28107,#28108,#28109,#28110,#28111,#28112,#28113),
 .UNSPECIFIED.,.F.,.F.,(4,2,2,2,2,2,4),(-0.921983674052104,-0.763174312937053,
-0.618141011889387,-0.428360064692964,-0.24740957459713,-0.123269265571007,
0.),.UNSPECIFIED.);
#1022=CONICAL_SURFACE('',#17964,4.15,0.785398163397535);
#1114=SHAPE_REPRESENTATION_RELATIONSHIP('SRR','None',#38687,#1128);
#1128=ADVANCED_BREP_SHAPE_REPRESENTATION('',(#1174),#38623);
#1148=STYLED_ITEM('',(#38766),#1174);
#1174=MANIFOLD_SOLID_BREP('Body1',#17614);
#1237=PLANE('',#17993);
#1238=PLANE('',#17994);
#1239=PLANE('',#17995);
#1240=PLANE('',#17996);
#1241=PLANE('',#17997);
#1242=PLANE('',#17998);
#1243=PLANE('',#17999);
#1244=PLANE('',#18000);
#1712=FACE_OUTER_BOUND('',#2720,.T.);
#1713=FACE_OUTER_BOUND('',#2721,.T.);
#1714=FACE_OUTER_BOUND('',#2722,.T.);
#1715=FACE_OUTER_BOUND('',#2723,.T.);
#1716=FACE_OUTER_BOUND('',#2724,.T.);
#1717=FACE_OUTER_BOUND('',#2725,.T.);
#1718=FACE_OUTER_BOUND('',#2726,.T.);
#1719=FACE_OUTER_BOUND('',#2727,.T.);
#1720=FACE_OUTER_BOUND('',#2728,.T.);
#1721=FACE_OUTER_BOUND('',#2729,.T.);
#1722=FACE_OUTER_BOUND('',#2730,.T.);
#1723=FACE_OUTER_BOUND('',#2731,.T.);
#1724=FACE_OUTER_BOUND('',#2732,.T.);
#1725=FACE_OUTER_BOUND('',#2733,.T.);
#1726=FACE_OUTER_BOUND('',#2734,.T.);
#1727=FACE_OUTER_BOUND('',#2735,.T.);
#1728=FACE_OUTER_BOUND('',#2736,.T.);
#1729=FACE_OUTER_BOUND('',#2737,.T.);
#1730=FACE_OUTER_BOUND('',#2738,.T.);
#1731=FACE_OUTER_BOUND('',#2739,.T.);
#1732=FACE_OUTER_BOUND('',#2740,.T.);
#1733=FACE_OUTER_BOUND('',#2741,.T.);
#1734=FACE_OUTER_BOUND('',#2742,.T.);
#1735=FACE_OUTER_BOUND('',#2743,.T.);
#1736=FACE_OUTER_BOUND('',#2744,.T.);
#1737=FACE_OUTER_BOUND('',#2745,.T.);
#1738=FACE_OUTER_BOUND('',#2746,.T.);
#1739=FACE_OUTER_BOUND('',#2747,.T.);
#1740=FACE_OUTER_BOUND('',#2748,.T.);
#1741=FACE_OUTER_BOUND('',#2749,.T.);
#1742=FACE_OUTER_BOUND('',#2750,.T.);
#1743=FACE_OUTER_BOUND('',#2751,.T.);
#1744=FACE_OUTER_BOUND('',#2752,.T.);
#1745=FACE_OUTER_BOUND('',#2753,.T.);
#1746=FACE_OUTER_BOUND('',#2754,.T.);
#1747=FACE_OUTER_BOUND('',#2755,.T.);
#1748=FACE_OUTER_BOUND('',#2756,.T.);
#1749=FACE_OUTER_BOUND('',#2757,.T.);
#1750=FACE_OUTER_BOUND('',#2758,.T.);
#1751=FACE_OUTER_BOUND('',#2759,.T.);
#1752=FACE_OUTER_BOUND('',#2760,.T.);
#1753=FACE_OUTER_BOUND('',#2761,.T.);
#1754=FACE_OUTER_BOUND('',#2762,.T.);
#1755=FACE_OUTER_BOUND('',#2763,.T.);
#1756=FACE_OUTER_BOUND('',#2764,.T.);
#1757=FACE_OUTER_BOUND('',#2765,.T.);
#1758=FACE_OUTER_BOUND('',#2766,.T.);
#1759=FACE_OUTER_BOUND('',#2767,.T.);
#1760=FACE_OUTER_BOUND('',#2768,.T.);
#1761=FACE_OUTER_BOUND('',#2769,.T.);
#1762=FACE_OUTER_BOUND('',#2770,.T.);
#1763=FACE_OUTER_BOUND('',#2771,.T.);
#1764=FACE_OUTER_BOUND('',#2772,.T.);
#1765=FACE_OUTER_BOUND('',#2773,.T.);
#1766=FACE_OUTER_BOUND('',#2774,.T.);
#1767=FACE_OUTER_BOUND('',#2775,.T.);
#1768=FACE_OUTER_BOUND('',#2776,.T.);
#1769=FACE_OUTER_BOUND('',#2777,.T.);
#1770=FACE_OUTER_BOUND('',#2778,.T.);
#1771=FACE_OUTER_BOUND('',#2780,.T.);
#1772=FACE_OUTER_BOUND('',#2782,.T.);
#1773=FACE_OUTER_BOUND('',#2784,.T.);
#1774=FACE_OUTER_BOUND('',#2786,.T.);
#1775=FACE_OUTER_BOUND('',#2788,.T.);
#1776=FACE_OUTER_BOUND('',#2789,.T.);
#1777=FACE_OUTER_BOUND('',#2790,.T.);
#1778=FACE_OUTER_BOUND('',#2791,.T.);
#1779=FACE_OUTER_BOUND('',#2792,.T.);
#1780=FACE_OUTER_BOUND('',#2793,.T.);
#1781=FACE_OUTER_BOUND('',#2794,.T.);
#1782=FACE_OUTER_BOUND('',#2795,.T.);
#2720=EDGE_LOOP('',(#11227,#11228,#11229,#11230));
#2721=EDGE_LOOP('',(#11231,#11232,#11233,#11234));
#2722=EDGE_LOOP('',(#11235,#11236,#11237,#11238));
#2723=EDGE_LOOP('',(#11239,#11240,#11241,#11242));
#2724=EDGE_LOOP('',(#11243,#11244,#11245,#11246));
#2725=EDGE_LOOP('',(#11247,#11248,#11249,#11250));
#2726=EDGE_LOOP('',(#11251,#11252,#11253,#11254));
#2727=EDGE_LOOP('',(#11255,#11256,#11257,#11258));
#2728=EDGE_LOOP('',(#11259,#11260,#11261,#11262));
#2729=EDGE_LOOP('',(#11263,#11264,#11265,#11266));
#2730=EDGE_LOOP('',(#11267,#11268,#11269,#11270));
#2731=EDGE_LOOP('',(#11271,#11272,#11273,#11274));
#2732=EDGE_LOOP('',(#11275,#11276,#11277,#11278));
#2733=EDGE_LOOP('',(#11279,#11280,#11281,#11282));
#2734=EDGE_LOOP('',(#11283,#11284,#11285,#11286));
#2735=EDGE_LOOP('',(#11287,#11288,#11289,#11290));
#2736=EDGE_LOOP('',(#11291,#11292,#11293,#11294));
#2737=EDGE_LOOP('',(#11295,#11296,#11297,#11298));
#2738=EDGE_LOOP('',(#11299,#11300,#11301,#11302));
#2739=EDGE_LOOP('',(#11303,#11304,#11305,#11306));
#2740=EDGE_LOOP('',(#11307,#11308,#11309,#11310));
#2741=EDGE_LOOP('',(#11311,#11312,#11313,#11314));
#2742=EDGE_LOOP('',(#11315,#11316,#11317,#11318));
#2743=EDGE_LOOP('',(#11319,#11320,#11321,#11322));
#2744=EDGE_LOOP('',(#11323,#11324,#11325,#11326));
#2745=EDGE_LOOP('',(#11327,#11328,#11329));
#2746=EDGE_LOOP('',(#11330,#11331,#11332,#11333,#11334,#11335));
#2747=EDGE_LOOP('',(#11336,#11337,#11338,#11339));
#2748=EDGE_LOOP('',(#11340,#11341,#11342,#11343));
#2749=EDGE_LOOP('',(#11344,#11345,#11346,#11347));
#2750=EDGE_LOOP('',(#11348,#11349,#11350,#11351));
#2751=EDGE_LOOP('',(#11352,#11353,#11354,#11355));
#2752=EDGE_LOOP('',(#11356,#11357,#11358,#11359));
#2753=EDGE_LOOP('',(#11360,#11361,#11362,#11363));
#2754=EDGE_LOOP('',(#11364,#11365,#11366,#11367));
#2755=EDGE_LOOP('',(#11368,#11369,#11370,#11371));
#2756=EDGE_LOOP('',(#11372,#11373,#11374,#11375));
#2757=EDGE_LOOP('',(#11376,#11377,#11378,#11379));
#2758=EDGE_LOOP('',(#11380,#11381,#11382,#11383));
#2759=EDGE_LOOP('',(#11384,#11385,#11386,#11387));
#2760=EDGE_LOOP('',(#11388,#11389,#11390,#11391));
#2761=EDGE_LOOP('',(#11392,#11393,#11394,#11395));
#2762=EDGE_LOOP('',(#11396,#11397,#11398,#11399));
#2763=EDGE_LOOP('',(#11400,#11401,#11402,#11403));
#2764=EDGE_LOOP('',(#11404,#11405,#11406,#11407));
#2765=EDGE_LOOP('',(#11408,#11409,#11410,#11411));
#2766=EDGE_LOOP('',(#11412,#11413,#11414,#11415));
#2767=EDGE_LOOP('',(#11416,#11417,#11418,#11419));
#2768=EDGE_LOOP('',(#11420,#11421,#11422,#11423));
#2769=EDGE_LOOP('',(#11424,#11425,#11426,#11427));
#2770=EDGE_LOOP('',(#11428,#11429,#11430,#11431,#11432));
#2771=EDGE_LOOP('',(#11433,#11434,#11435,#11436,#11437,#11438,#11439,#11440,
#11441,#11442,#11443,#11444));
#2772=EDGE_LOOP('',(#11445,#11446,#11447,#11448));
#2773=EDGE_LOOP('',(#11449,#11450,#11451,#11452,#11453,#11454,#11455,#11456,
#11457,#11458,#11459,#11460));
#2774=EDGE_LOOP('',(#11461,#11462,#11463,#11464));
#2775=EDGE_LOOP('',(#11465,#11466,#11467,#11468));
#2776=EDGE_LOOP('',(#11469,#11470,#11471,#11472));
#2777=EDGE_LOOP('',(#11473,#11474,#11475,#11476));
#2778=EDGE_LOOP('',(#11477));
#2779=EDGE_LOOP('',(#11478,#11479,#11480,#11481));
#2780=EDGE_LOOP('',(#11482));
#2781=EDGE_LOOP('',(#11483));
#2782=EDGE_LOOP('',(#11484));
#2783=EDGE_LOOP('',(#11485));
#2784=EDGE_LOOP('',(#11486));
#2785=EDGE_LOOP('',(#11487));
#2786=EDGE_LOOP('',(#11488));
#2787=EDGE_LOOP('',(#11489));
#2788=EDGE_LOOP('',(#11490,#11491,#11492,#11493));
#2789=EDGE_LOOP('',(#11494,#11495,#11496,#11497,#11498,#11499));
#2790=EDGE_LOOP('',(#11500,#11501,#11502,#11503));
#2791=EDGE_LOOP('',(#11504,#11505,#11506,#11507,#11508,#11509));
#2792=EDGE_LOOP('',(#11510,#11511,#11512,#11513));
#2793=EDGE_LOOP('',(#11514,#11515,#11516,#11517));
#2794=EDGE_LOOP('',(#11518,#11519,#11520,#11521,#11522,#11523,#11524,#11525,
#11526,#11527,#11528,#11529,#11530,#11531,#11532,#11533,#11534,#11535,#11536,
#11537,#11538,#11539,#11540,#11541,#11542,#11543,#11544,#11545,#11546,#11547,
#11548,#11549,#11550,#11551,#11552,#11553,#11554,#11555,#11556,#11557,#11558,
#11559,#11560,#11561,#11562,#11563,#11564,#11565,#11566,#11567,#11568,#11569,
#11570,#11571));
#2795=EDGE_LOOP('',(#11572,#11573,#11574,#11575,#11576,#11577,#11578,#11579,
#11580,#11581,#11582,#11583,#11584,#11585,#11586,#11587,#11588,#11589,#11590,
#11591,#11592,#11593,#11594,#11595,#11596,#11597,#11598,#11599,#11600,#11601,
#11602,#11603,#11604,#11605,#11606,#11607,#11608,#11609,#11610,#11611,#11612,
#11613,#11614,#11615,#11616,#11617,#11618,#11619,#11620,#11621,#11622,#11623,
#11624));
#3808=LINE('',#24975,#4752);
#3809=LINE('',#24985,#4753);
#3810=LINE('',#24996,#4754);
#3811=LINE('',#25026,#4755);
#3812=LINE('',#25056,#4756);
#3813=LINE('',#25086,#4757);
#3814=LINE('',#25116,#4758);
#3815=LINE('',#25146,#4759);
#3816=LINE('',#25176,#4760);
#3817=LINE('',#25206,#4761);
#3818=LINE('',#25236,#4762);
#3819=LINE('',#25266,#4763);
#3820=LINE('',#25296,#4764);
#3821=LINE('',#25326,#4765);
#3822=LINE('',#25356,#4766);
#3823=LINE('',#25386,#4767);
#3824=LINE('',#25416,#4768);
#3825=LINE('',#25446,#4769);
#3826=LINE('',#25476,#4770);
#3827=LINE('',#25506,#4771);
#3828=LINE('',#25536,#4772);
#3829=LINE('',#25566,#4773);
#3830=LINE('',#25596,#4774);
#3831=LINE('',#25626,#4775);
#3832=LINE('',#25656,#4776);
#3833=LINE('',#25686,#4777);
#3834=LINE('',#25703,#4778);
#3835=LINE('',#25745,#4779);
#3836=LINE('',#25783,#4780);
#3837=LINE('',#25826,#4781);
#3838=LINE('',#25902,#4782);
#3839=LINE('',#25978,#4783);
#3840=LINE('',#26054,#4784);
#3841=LINE('',#26130,#4785);
#3842=LINE('',#26208,#4786);
#3843=LINE('',#26286,#4787);
#3844=LINE('',#26362,#4788);
#3845=LINE('',#26438,#4789);
#3846=LINE('',#26514,#4790);
#3847=LINE('',#26590,#4791);
#3848=LINE('',#26670,#4792);
#3849=LINE('',#26746,#4793);
#3850=LINE('',#26822,#4794);
#3851=LINE('',#26898,#4795);
#3852=LINE('',#26974,#4796);
#3853=LINE('',#27050,#4797);
#3854=LINE('',#27130,#4798);
#3855=LINE('',#27206,#4799);
#3856=LINE('',#27282,#4800);
#3857=LINE('',#27358,#4801);
#3858=LINE('',#27434,#4802);
#3859=LINE('',#27510,#4803);
#3860=LINE('',#27540,#4804);
#3861=LINE('',#27546,#4805);
#3862=LINE('',#27587,#4806);
#3863=LINE('',#27637,#4807);
#3864=LINE('',#27815,#4808);
#3865=LINE('',#28001,#4809);
#3866=LINE('',#28006,#4810);
#3867=LINE('',#28226,#4811);
#3868=LINE('',#28227,#4812);
#3869=LINE('',#28229,#4813);
#3870=LINE('',#28338,#4814);
#3871=LINE('',#28341,#4815);
#3872=LINE('',#28342,#4816);
#4752=VECTOR('',#20101,4.29685191531258);
#4753=VECTOR('',#20102,1000.);
#4754=VECTOR('',#20105,4.29685191531258);
#4755=VECTOR('',#20108,4.29685191531258);
#4756=VECTOR('',#20111,4.29685191531258);
#4757=VECTOR('',#20114,4.29685191531258);
#4758=VECTOR('',#20117,4.29685191531258);
#4759=VECTOR('',#20120,4.29685191531258);
#4760=VECTOR('',#20123,4.29685191531258);
#4761=VECTOR('',#20126,4.29685191531258);
#4762=VECTOR('',#20129,4.29685191531258);
#4763=VECTOR('',#20132,4.29685191531258);
#4764=VECTOR('',#20135,4.29685191531258);
#4765=VECTOR('',#20138,4.29685191531258);
#4766=VECTOR('',#20141,4.29685191531258);
#4767=VECTOR('',#20144,4.29685191531258);
#4768=VECTOR('',#20147,4.29685191531258);
#4769=VECTOR('',#20150,4.29685191531258);
#4770=VECTOR('',#20153,4.29685191531258);
#4771=VECTOR('',#20156,4.29685191531258);
#4772=VECTOR('',#20159,4.29685191531258);
#4773=VECTOR('',#20162,4.29685191531258);
#4774=VECTOR('',#20165,4.29685191531258);
#4775=VECTOR('',#20168,4.29685191531258);
#4776=VECTOR('',#20171,4.29685191531258);
#4777=VECTOR('',#20174,4.29685191531258);
#4778=VECTOR('',#20179,4.12499999999999);
#4779=VECTOR('',#20184,4.12499999999999);
#4780=VECTOR('',#20185,1000.);
#4781=VECTOR('',#20190,4.12499999999999);
#4782=VECTOR('',#20193,4.12499999999999);
#4783=VECTOR('',#20196,4.12499999999999);
#4784=VECTOR('',#20199,4.12499999999999);
#4785=VECTOR('',#20202,4.12499999999999);
#4786=VECTOR('',#20205,4.12499999999999);
#4787=VECTOR('',#20208,4.12499999999999);
#4788=VECTOR('',#20211,4.12499999999999);
#4789=VECTOR('',#20214,4.12499999999999);
#4790=VECTOR('',#20217,4.12499999999999);
#4791=VECTOR('',#20220,4.12499999999999);
#4792=VECTOR('',#20223,4.12499999999999);
#4793=VECTOR('',#20226,4.12499999999999);
#4794=VECTOR('',#20229,4.12499999999999);
#4795=VECTOR('',#20232,4.12499999999999);
#4796=VECTOR('',#20235,4.12499999999999);
#4797=VECTOR('',#20238,4.12499999999999);
#4798=VECTOR('',#20241,4.12499999999999);
#4799=VECTOR('',#20244,4.12499999999999);
#4800=VECTOR('',#20247,4.12499999999999);
#4801=VECTOR('',#20250,4.12499999999999);
#4802=VECTOR('',#20253,4.12499999999999);
#4803=VECTOR('',#20256,4.12499999999999);
#4804=VECTOR('',#20261,4.15);
#4805=VECTOR('',#20268,8.);
#4806=VECTOR('',#20273,8.);
#4807=VECTOR('',#20292,12.5);
#4808=VECTOR('',#20297,12.5);
#4809=VECTOR('',#20314,25.);
#4810=VECTOR('',#20319,22.5);
#4811=VECTOR('',#20334,10.);
#4812=VECTOR('',#20335,10.);
#4813=VECTOR('',#20338,10.);
#4814=VECTOR('',#20339,10.);
#4815=VECTOR('',#20344,1000.);
#4816=VECTOR('',#20345,1000.);
#5634=CIRCLE('',#17935,4.29685191531251);
#5635=CIRCLE('',#17937,4.125);
#5636=CIRCLE('',#17939,4.125);
#5637=CIRCLE('',#17963,4.12499999999999);
#5638=CIRCLE('',#17965,4.15);
#5639=CIRCLE('',#17967,8.);
#5640=CIRCLE('',#17968,8.);
#5641=CIRCLE('',#17969,8.);
#5642=CIRCLE('',#17970,8.);
#5643=CIRCLE('',#17971,8.);
#5644=CIRCLE('',#17972,8.);
#5645=CIRCLE('',#17974,12.5);
#5646=CIRCLE('',#17975,1.00000000000001);
#5647=CIRCLE('',#17976,11.5);
#5648=CIRCLE('',#17978,12.5);
#5649=CIRCLE('',#17979,12.5);
#5650=CIRCLE('',#17980,12.5);
#5651=CIRCLE('',#17981,12.5);
#5652=CIRCLE('',#17982,12.5);
#5653=CIRCLE('',#17984,25.);
#5654=CIRCLE('',#17985,2.25);
#5655=CIRCLE('',#17986,22.75);
#5656=CIRCLE('',#17988,25.);
#5657=CIRCLE('',#17990,22.5);
#5658=CIRCLE('',#17991,22.5);
#6618=VERTEX_POINT('',#24973);
#6619=VERTEX_POINT('',#24974);
#6620=VERTEX_POINT('',#24976);
#6621=VERTEX_POINT('',#24984);
#6622=VERTEX_POINT('',#24994);
#6623=VERTEX_POINT('',#24995);
#6624=VERTEX_POINT('',#25024);
#6625=VERTEX_POINT('',#25025);
#6626=VERTEX_POINT('',#25054);
#6627=VERTEX_POINT('',#25055);
#6628=VERTEX_POINT('',#25084);
#6629=VERTEX_POINT('',#25085);
#6630=VERTEX_POINT('',#25114);
#6631=VERTEX_POINT('',#25115);
#6632=VERTEX_POINT('',#25144);
#6633=VERTEX_POINT('',#25145);
#6634=VERTEX_POINT('',#25174);
#6635=VERTEX_POINT('',#25175);
#6636=VERTEX_POINT('',#25204);
#6637=VERTEX_POINT('',#25205);
#6638=VERTEX_POINT('',#25234);
#6639=VERTEX_POINT('',#25235);
#6640=VERTEX_POINT('',#25264);
#6641=VERTEX_POINT('',#25265);
#6642=VERTEX_POINT('',#25294);
#6643=VERTEX_POINT('',#25295);
#6644=VERTEX_POINT('',#25324);
#6645=VERTEX_POINT('',#25325);
#6646=VERTEX_POINT('',#25354);
#6647=VERTEX_POINT('',#25355);
#6648=VERTEX_POINT('',#25384);
#6649=VERTEX_POINT('',#25385);
#6650=VERTEX_POINT('',#25414);
#6651=VERTEX_POINT('',#25415);
#6652=VERTEX_POINT('',#25444);
#6653=VERTEX_POINT('',#25445);
#6654=VERTEX_POINT('',#25474);
#6655=VERTEX_POINT('',#25475);
#6656=VERTEX_POINT('',#25504);
#6657=VERTEX_POINT('',#25505);
#6658=VERTEX_POINT('',#25534);
#6659=VERTEX_POINT('',#25535);
#6660=VERTEX_POINT('',#25564);
#6661=VERTEX_POINT('',#25565);
#6662=VERTEX_POINT('',#25594);
#6663=VERTEX_POINT('',#25595);
#6664=VERTEX_POINT('',#25624);
#6665=VERTEX_POINT('',#25625);
#6666=VERTEX_POINT('',#25654);
#6667=VERTEX_POINT('',#25655);
#6668=VERTEX_POINT('',#25684);
#6669=VERTEX_POINT('',#25685);
#6670=VERTEX_POINT('',#25687);
#6671=VERTEX_POINT('',#25693);
#6672=VERTEX_POINT('',#25701);
#6673=VERTEX_POINT('',#25702);
#6674=VERTEX_POINT('',#25704);
#6675=VERTEX_POINT('',#25743);
#6676=VERTEX_POINT('',#25744);
#6677=VERTEX_POINT('',#25746);
#6678=VERTEX_POINT('',#25824);
#6679=VERTEX_POINT('',#25825);
#6680=VERTEX_POINT('',#25900);
#6681=VERTEX_POINT('',#25901);
#6682=VERTEX_POINT('',#25976);
#6683=VERTEX_POINT('',#25977);
#6684=VERTEX_POINT('',#26052);
#6685=VERTEX_POINT('',#26053);
#6686=VERTEX_POINT('',#26128);
#6687=VERTEX_POINT('',#26129);
#6688=VERTEX_POINT('',#26206);
#6689=VERTEX_POINT('',#26207);
#6690=VERTEX_POINT('',#26284);
#6691=VERTEX_POINT('',#26285);
#6692=VERTEX_POINT('',#26360);
#6693=VERTEX_POINT('',#26361);
#6694=VERTEX_POINT('',#26436);
#6695=VERTEX_POINT('',#26437);
#6696=VERTEX_POINT('',#26512);
#6697=VERTEX_POINT('',#26513);
#6698=VERTEX_POINT('',#26588);
#6699=VERTEX_POINT('',#26589);
#6700=VERTEX_POINT('',#26668);
#6701=VERTEX_POINT('',#26669);
#6702=VERTEX_POINT('',#26744);
#6703=VERTEX_POINT('',#26745);
#6704=VERTEX_POINT('',#26820);
#6705=VERTEX_POINT('',#26821);
#6706=VERTEX_POINT('',#26896);
#6707=VERTEX_POINT('',#26897);
#6708=VERTEX_POINT('',#26972);
#6709=VERTEX_POINT('',#26973);
#6710=VERTEX_POINT('',#27048);
#6711=VERTEX_POINT('',#27049);
#6712=VERTEX_POINT('',#27128);
#6713=VERTEX_POINT('',#27129);
#6714=VERTEX_POINT('',#27204);
#6715=VERTEX_POINT('',#27205);
#6716=VERTEX_POINT('',#27280);
#6717=VERTEX_POINT('',#27281);
#6718=VERTEX_POINT('',#27356);
#6719=VERTEX_POINT('',#27357);
#6720=VERTEX_POINT('',#27432);
#6721=VERTEX_POINT('',#27433);
#6722=VERTEX_POINT('',#27508);
#6723=VERTEX_POINT('',#27509);
#6724=VERTEX_POINT('',#27511);
#6725=VERTEX_POINT('',#27520);
#6726=VERTEX_POINT('',#27539);
#6727=VERTEX_POINT('',#27543);
#6728=VERTEX_POINT('',#27545);
#6729=VERTEX_POINT('',#27547);
#6730=VERTEX_POINT('',#27549);
#6731=VERTEX_POINT('',#27584);
#6732=VERTEX_POINT('',#27586);
#6733=VERTEX_POINT('',#27589);
#6734=VERTEX_POINT('',#27591);
#6735=VERTEX_POINT('',#27628);
#6736=VERTEX_POINT('',#27630);
#6737=VERTEX_POINT('',#27634);
#6738=VERTEX_POINT('',#27636);
#6739=VERTEX_POINT('',#27638);
#6740=VERTEX_POINT('',#27640);
#6741=VERTEX_POINT('',#27813);
#6742=VERTEX_POINT('',#27816);
#6743=VERTEX_POINT('',#27818);
#6744=VERTEX_POINT('',#27993);
#6745=VERTEX_POINT('',#27995);
#6746=VERTEX_POINT('',#27999);
#6747=VERTEX_POINT('',#28003);
#6748=VERTEX_POINT('',#28005);
#8400=EDGE_CURVE('',#6618,#6619,#3808,.T.);
#8401=EDGE_CURVE('',#6620,#6619,#186,.T.);
#8402=EDGE_CURVE('',#6620,#6621,#3809,.T.);
#8403=EDGE_CURVE('',#6621,#6618,#187,.T.);
#8404=EDGE_CURVE('',#6622,#6623,#3810,.T.);
#8405=EDGE_CURVE('',#6619,#6623,#188,.T.);
#8406=EDGE_CURVE('',#6618,#6622,#189,.T.);
#8407=EDGE_CURVE('',#6624,#6625,#3811,.T.);
#8408=EDGE_CURVE('',#6623,#6625,#190,.T.);
#8409=EDGE_CURVE('',#6622,#6624,#191,.T.);
#8410=EDGE_CURVE('',#6626,#6627,#3812,.T.);
#8411=EDGE_CURVE('',#6625,#6627,#192,.T.);
#8412=EDGE_CURVE('',#6624,#6626,#193,.T.);
#8413=EDGE_CURVE('',#6628,#6629,#3813,.T.);
#8414=EDGE_CURVE('',#6627,#6629,#194,.T.);
#8415=EDGE_CURVE('',#6626,#6628,#195,.T.);
#8416=EDGE_CURVE('',#6630,#6631,#3814,.T.);
#8417=EDGE_CURVE('',#6629,#6631,#196,.T.);
#8418=EDGE_CURVE('',#6628,#6630,#197,.T.);
#8419=EDGE_CURVE('',#6632,#6633,#3815,.T.);
#8420=EDGE_CURVE('',#6631,#6633,#198,.T.);
#8421=EDGE_CURVE('',#6630,#6632,#199,.T.);
#8422=EDGE_CURVE('',#6634,#6635,#3816,.T.);
#8423=EDGE_CURVE('',#6633,#6635,#200,.T.);
#8424=EDGE_CURVE('',#6632,#6634,#201,.T.);
#8425=EDGE_CURVE('',#6636,#6637,#3817,.T.);
#8426=EDGE_CURVE('',#6635,#6637,#202,.T.);
#8427=EDGE_CURVE('',#6634,#6636,#203,.T.);
#8428=EDGE_CURVE('',#6638,#6639,#3818,.T.);
#8429=EDGE_CURVE('',#6637,#6639,#204,.T.);
#8430=EDGE_CURVE('',#6636,#6638,#205,.T.);
#8431=EDGE_CURVE('',#6640,#6641,#3819,.T.);
#8432=EDGE_CURVE('',#6639,#6641,#206,.T.);
#8433=EDGE_CURVE('',#6638,#6640,#207,.T.);
#8434=EDGE_CURVE('',#6642,#6643,#3820,.T.);
#8435=EDGE_CURVE('',#6641,#6643,#208,.T.);
#8436=EDGE_CURVE('',#6640,#6642,#209,.T.);
#8437=EDGE_CURVE('',#6644,#6645,#3821,.T.);
#8438=EDGE_CURVE('',#6643,#6645,#210,.T.);
#8439=EDGE_CURVE('',#6642,#6644,#211,.T.);
#8440=EDGE_CURVE('',#6646,#6647,#3822,.T.);
#8441=EDGE_CURVE('',#6645,#6647,#212,.T.);
#8442=EDGE_CURVE('',#6644,#6646,#213,.T.);
#8443=EDGE_CURVE('',#6648,#6649,#3823,.T.);
#8444=EDGE_CURVE('',#6647,#6649,#214,.T.);
#8445=EDGE_CURVE('',#6646,#6648,#215,.T.);
#8446=EDGE_CURVE('',#6650,#6651,#3824,.T.);
#8447=EDGE_CURVE('',#6649,#6651,#216,.T.);
#8448=EDGE_CURVE('',#6648,#6650,#217,.T.);
#8449=EDGE_CURVE('',#6652,#6653,#3825,.T.);
#8450=EDGE_CURVE('',#6651,#6653,#218,.T.);
#8451=EDGE_CURVE('',#6650,#6652,#219,.T.);
#8452=EDGE_CURVE('',#6654,#6655,#3826,.T.);
#8453=EDGE_CURVE('',#6653,#6655,#220,.T.);
#8454=EDGE_CURVE('',#6652,#6654,#221,.T.);
#8455=EDGE_CURVE('',#6656,#6657,#3827,.T.);
#8456=EDGE_CURVE('',#6655,#6657,#222,.T.);
#8457=EDGE_CURVE('',#6654,#6656,#223,.T.);
#8458=EDGE_CURVE('',#6658,#6659,#3828,.T.);
#8459=EDGE_CURVE('',#6657,#6659,#224,.T.);
#8460=EDGE_CURVE('',#6656,#6658,#225,.T.);
#8461=EDGE_CURVE('',#6660,#6661,#3829,.T.);
#8462=EDGE_CURVE('',#6659,#6661,#226,.T.);
#8463=EDGE_CURVE('',#6658,#6660,#227,.T.);
#8464=EDGE_CURVE('',#6662,#6663,#3830,.T.);
#8465=EDGE_CURVE('',#6661,#6663,#228,.T.);
#8466=EDGE_CURVE('',#6660,#6662,#229,.T.);
#8467=EDGE_CURVE('',#6664,#6665,#3831,.T.);
#8468=EDGE_CURVE('',#6663,#6665,#230,.T.);
#8469=EDGE_CURVE('',#6662,#6664,#231,.T.);
#8470=EDGE_CURVE('',#6666,#6667,#3832,.T.);
#8471=EDGE_CURVE('',#6665,#6667,#232,.T.);
#8472=EDGE_CURVE('',#6664,#6666,#233,.T.);
#8473=EDGE_CURVE('',#6668,#6669,#3833,.T.);
#8474=EDGE_CURVE('',#6668,#6670,#234,.T.);
#8475=EDGE_CURVE('',#6671,#6670,#5634,.T.);
#8476=EDGE_CURVE('',#6669,#6671,#235,.T.);
#8477=EDGE_CURVE('',#6672,#6673,#3834,.T.);
#8478=EDGE_CURVE('',#6673,#6674,#5635,.T.);
#8479=EDGE_CURVE('',#6674,#6672,#908,.T.);
#8480=EDGE_CURVE('',#6675,#6676,#3835,.T.);
#8481=EDGE_CURVE('',#6677,#6676,#909,.F.);
#8482=EDGE_CURVE('',#6677,#6674,#3836,.T.);
#8483=EDGE_CURVE('',#6674,#6673,#5636,.T.);
#8484=EDGE_CURVE('',#6672,#6675,#910,.T.);
#8485=EDGE_CURVE('',#6678,#6679,#3837,.T.);
#8486=EDGE_CURVE('',#6676,#6679,#911,.F.);
#8487=EDGE_CURVE('',#6675,#6678,#912,.T.);
#8488=EDGE_CURVE('',#6680,#6681,#3838,.T.);
#8489=EDGE_CURVE('',#6679,#6681,#913,.F.);
#8490=EDGE_CURVE('',#6678,#6680,#914,.T.);
#8491=EDGE_CURVE('',#6682,#6683,#3839,.T.);
#8492=EDGE_CURVE('',#6681,#6683,#915,.F.);
#8493=EDGE_CURVE('',#6680,#6682,#916,.T.);
#8494=EDGE_CURVE('',#6684,#6685,#3840,.T.);
#8495=EDGE_CURVE('',#6683,#6685,#917,.F.);
#8496=EDGE_CURVE('',#6682,#6684,#918,.T.);
#8497=EDGE_CURVE('',#6686,#6687,#3841,.T.);
#8498=EDGE_CURVE('',#6685,#6687,#919,.F.);
#8499=EDGE_CURVE('',#6684,#6686,#920,.T.);
#8500=EDGE_CURVE('',#6688,#6689,#3842,.T.);
#8501=EDGE_CURVE('',#6687,#6689,#921,.F.);
#8502=EDGE_CURVE('',#6686,#6688,#922,.T.);
#8503=EDGE_CURVE('',#6690,#6691,#3843,.T.);
#8504=EDGE_CURVE('',#6689,#6691,#923,.F.);
#8505=EDGE_CURVE('',#6688,#6690,#924,.T.);
#8506=EDGE_CURVE('',#6692,#6693,#3844,.T.);
#8507=EDGE_CURVE('',#6691,#6693,#925,.F.);
#8508=EDGE_CURVE('',#6690,#6692,#926,.T.);
#8509=EDGE_CURVE('',#6694,#6695,#3845,.T.);
#8510=EDGE_CURVE('',#6693,#6695,#927,.F.);
#8511=EDGE_CURVE('',#6692,#6694,#928,.T.);
#8512=EDGE_CURVE('',#6696,#6697,#3846,.T.);
#8513=EDGE_CURVE('',#6695,#6697,#929,.F.);
#8514=EDGE_CURVE('',#6694,#6696,#930,.T.);
#8515=EDGE_CURVE('',#6698,#6699,#3847,.T.);
#8516=EDGE_CURVE('',#6697,#6699,#931,.F.);
#8517=EDGE_CURVE('',#6696,#6698,#932,.T.);
#8518=EDGE_CURVE('',#6700,#6701,#3848,.T.);
#8519=EDGE_CURVE('',#6699,#6701,#933,.F.);
#8520=EDGE_CURVE('',#6698,#6700,#934,.T.);
#8521=EDGE_CURVE('',#6702,#6703,#3849,.T.);
#8522=EDGE_CURVE('',#6701,#6703,#935,.F.);
#8523=EDGE_CURVE('',#6700,#6702,#936,.T.);
#8524=EDGE_CURVE('',#6704,#6705,#3850,.T.);
#8525=EDGE_CURVE('',#6703,#6705,#937,.F.);
#8526=EDGE_CURVE('',#6702,#6704,#938,.T.);
#8527=EDGE_CURVE('',#6706,#6707,#3851,.T.);
#8528=EDGE_CURVE('',#6705,#6707,#939,.F.);
#8529=EDGE_CURVE('',#6704,#6706,#940,.T.);
#8530=EDGE_CURVE('',#6708,#6709,#3852,.T.);
#8531=EDGE_CURVE('',#6707,#6709,#941,.F.);
#8532=EDGE_CURVE('',#6706,#6708,#942,.T.);
#8533=EDGE_CURVE('',#6710,#6711,#3853,.T.);
#8534=EDGE_CURVE('',#6709,#6711,#943,.F.);
#8535=EDGE_CURVE('',#6708,#6710,#944,.T.);
#8536=EDGE_CURVE('',#6712,#6713,#3854,.T.);
#8537=EDGE_CURVE('',#6711,#6713,#945,.F.);
#8538=EDGE_CURVE('',#6710,#6712,#946,.T.);
#8539=EDGE_CURVE('',#6714,#6715,#3855,.T.);
#8540=EDGE_CURVE('',#6713,#6715,#947,.F.);
#8541=EDGE_CURVE('',#6712,#6714,#948,.T.);
#8542=EDGE_CURVE('',#6716,#6717,#3856,.T.);
#8543=EDGE_CURVE('',#6715,#6717,#949,.F.);
#8544=EDGE_CURVE('',#6714,#6716,#950,.T.);
#8545=EDGE_CURVE('',#6718,#6719,#3857,.T.);
#8546=EDGE_CURVE('',#6717,#6719,#951,.F.);
#8547=EDGE_CURVE('',#6716,#6718,#952,.T.);
#8548=EDGE_CURVE('',#6720,#6721,#3858,.T.);
#8549=EDGE_CURVE('',#6719,#6721,#953,.F.);
#8550=EDGE_CURVE('',#6718,#6720,#954,.T.);
#8551=EDGE_CURVE('',#6722,#6723,#3859,.T.);
#8552=EDGE_CURVE('',#6722,#6724,#955,.T.);
#8553=EDGE_CURVE('',#6724,#6725,#5637,.T.);
#8554=EDGE_CURVE('',#6723,#6725,#956,.F.);
#8555=EDGE_CURVE('',#6673,#6726,#3860,.T.);
#8556=EDGE_CURVE('',#6726,#6726,#5638,.T.);
#8557=EDGE_CURVE('',#6727,#6727,#5639,.T.);
#8558=EDGE_CURVE('',#6727,#6728,#3861,.T.);
#8559=EDGE_CURVE('',#6729,#6728,#5640,.T.);
#8560=EDGE_CURVE('',#6730,#6729,#957,.T.);
#8561=EDGE_CURVE('',#6731,#6730,#5641,.T.);
#8562=EDGE_CURVE('',#6731,#6732,#3862,.T.);
#8563=EDGE_CURVE('',#6732,#6732,#5642,.T.);
#8564=EDGE_CURVE('',#6733,#6731,#5643,.T.);
#8565=EDGE_CURVE('',#6734,#6733,#958,.T.);
#8566=EDGE_CURVE('',#6728,#6734,#5644,.T.);
#8567=EDGE_CURVE('',#6735,#6735,#5645,.T.);
#8568=EDGE_CURVE('',#6735,#6736,#5646,.T.);
#8569=EDGE_CURVE('',#6736,#6736,#5647,.T.);
#8570=EDGE_CURVE('',#6737,#6737,#5648,.T.);
#8571=EDGE_CURVE('',#6737,#6738,#3863,.T.);
#8572=EDGE_CURVE('',#6738,#6739,#5649,.T.);
#8573=EDGE_CURVE('',#6740,#6739,#959,.T.);
#8574=EDGE_CURVE('',#6741,#6740,#5650,.T.);
#8575=EDGE_CURVE('',#6741,#6735,#3864,.T.);
#8576=EDGE_CURVE('',#6742,#6741,#5651,.T.);
#8577=EDGE_CURVE('',#6743,#6742,#960,.T.);
#8578=EDGE_CURVE('',#6743,#6738,#5652,.T.);
#8579=EDGE_CURVE('',#6744,#6744,#5653,.T.);
#8580=EDGE_CURVE('',#6744,#6745,#5654,.T.);
#8581=EDGE_CURVE('',#6745,#6745,#5655,.T.);
#8582=EDGE_CURVE('',#6746,#6746,#5656,.T.);
#8583=EDGE_CURVE('',#6746,#6744,#3865,.T.);
#8584=EDGE_CURVE('',#6747,#6747,#5657,.T.);
#8585=EDGE_CURVE('',#6747,#6748,#3866,.T.);
#8586=EDGE_CURVE('',#6748,#6748,#5658,.T.);
#8587=EDGE_CURVE('',#6721,#6723,#961,.F.);
#8588=EDGE_CURVE('',#6720,#6722,#962,.T.);
#8589=EDGE_CURVE('',#6724,#6671,#963,.T.);
#8590=EDGE_CURVE('',#6670,#6725,#964,.T.);
#8591=EDGE_CURVE('',#6733,#6743,#3867,.T.);
#8592=EDGE_CURVE('',#6734,#6742,#3868,.T.);
#8593=EDGE_CURVE('',#6729,#6740,#3869,.T.);
#8594=EDGE_CURVE('',#6730,#6739,#3870,.T.);
#8595=EDGE_CURVE('',#6674,#6620,#3871,.T.);
#8596=EDGE_CURVE('',#6621,#6677,#3872,.T.);
#8597=EDGE_CURVE('',#6667,#6669,#236,.T.);
#8598=EDGE_CURVE('',#6666,#6668,#237,.T.);
#11227=ORIENTED_EDGE('',*,*,#8400,.T.);
#11228=ORIENTED_EDGE('',*,*,#8401,.F.);
#11229=ORIENTED_EDGE('',*,*,#8402,.T.);
#11230=ORIENTED_EDGE('',*,*,#8403,.T.);
#11231=ORIENTED_EDGE('',*,*,#8404,.T.);
#11232=ORIENTED_EDGE('',*,*,#8405,.F.);
#11233=ORIENTED_EDGE('',*,*,#8400,.F.);
#11234=ORIENTED_EDGE('',*,*,#8406,.T.);
#11235=ORIENTED_EDGE('',*,*,#8407,.T.);
#11236=ORIENTED_EDGE('',*,*,#8408,.F.);
#11237=ORIENTED_EDGE('',*,*,#8404,.F.);
#11238=ORIENTED_EDGE('',*,*,#8409,.T.);
#11239=ORIENTED_EDGE('',*,*,#8410,.T.);
#11240=ORIENTED_EDGE('',*,*,#8411,.F.);
#11241=ORIENTED_EDGE('',*,*,#8407,.F.);
#11242=ORIENTED_EDGE('',*,*,#8412,.T.);
#11243=ORIENTED_EDGE('',*,*,#8413,.T.);
#11244=ORIENTED_EDGE('',*,*,#8414,.F.);
#11245=ORIENTED_EDGE('',*,*,#8410,.F.);
#11246=ORIENTED_EDGE('',*,*,#8415,.T.);
#11247=ORIENTED_EDGE('',*,*,#8416,.T.);
#11248=ORIENTED_EDGE('',*,*,#8417,.F.);
#11249=ORIENTED_EDGE('',*,*,#8413,.F.);
#11250=ORIENTED_EDGE('',*,*,#8418,.T.);
#11251=ORIENTED_EDGE('',*,*,#8419,.T.);
#11252=ORIENTED_EDGE('',*,*,#8420,.F.);
#11253=ORIENTED_EDGE('',*,*,#8416,.F.);
#11254=ORIENTED_EDGE('',*,*,#8421,.T.);
#11255=ORIENTED_EDGE('',*,*,#8422,.T.);
#11256=ORIENTED_EDGE('',*,*,#8423,.F.);
#11257=ORIENTED_EDGE('',*,*,#8419,.F.);
#11258=ORIENTED_EDGE('',*,*,#8424,.T.);
#11259=ORIENTED_EDGE('',*,*,#8425,.T.);
#11260=ORIENTED_EDGE('',*,*,#8426,.F.);
#11261=ORIENTED_EDGE('',*,*,#8422,.F.);
#11262=ORIENTED_EDGE('',*,*,#8427,.T.);
#11263=ORIENTED_EDGE('',*,*,#8428,.T.);
#11264=ORIENTED_EDGE('',*,*,#8429,.F.);
#11265=ORIENTED_EDGE('',*,*,#8425,.F.);
#11266=ORIENTED_EDGE('',*,*,#8430,.T.);
#11267=ORIENTED_EDGE('',*,*,#8431,.T.);
#11268=ORIENTED_EDGE('',*,*,#8432,.F.);
#11269=ORIENTED_EDGE('',*,*,#8428,.F.);
#11270=ORIENTED_EDGE('',*,*,#8433,.T.);
#11271=ORIENTED_EDGE('',*,*,#8434,.T.);
#11272=ORIENTED_EDGE('',*,*,#8435,.F.);
#11273=ORIENTED_EDGE('',*,*,#8431,.F.);
#11274=ORIENTED_EDGE('',*,*,#8436,.T.);
#11275=ORIENTED_EDGE('',*,*,#8437,.T.);
#11276=ORIENTED_EDGE('',*,*,#8438,.F.);
#11277=ORIENTED_EDGE('',*,*,#8434,.F.);
#11278=ORIENTED_EDGE('',*,*,#8439,.T.);
#11279=ORIENTED_EDGE('',*,*,#8440,.T.);
#11280=ORIENTED_EDGE('',*,*,#8441,.F.);
#11281=ORIENTED_EDGE('',*,*,#8437,.F.);
#11282=ORIENTED_EDGE('',*,*,#8442,.T.);
#11283=ORIENTED_EDGE('',*,*,#8443,.T.);
#11284=ORIENTED_EDGE('',*,*,#8444,.F.);
#11285=ORIENTED_EDGE('',*,*,#8440,.F.);
#11286=ORIENTED_EDGE('',*,*,#8445,.T.);
#11287=ORIENTED_EDGE('',*,*,#8446,.T.);
#11288=ORIENTED_EDGE('',*,*,#8447,.F.);
#11289=ORIENTED_EDGE('',*,*,#8443,.F.);
#11290=ORIENTED_EDGE('',*,*,#8448,.T.);
#11291=ORIENTED_EDGE('',*,*,#8449,.T.);
#11292=ORIENTED_EDGE('',*,*,#8450,.F.);
#11293=ORIENTED_EDGE('',*,*,#8446,.F.);
#11294=ORIENTED_EDGE('',*,*,#8451,.T.);
#11295=ORIENTED_EDGE('',*,*,#8452,.T.);
#11296=ORIENTED_EDGE('',*,*,#8453,.F.);
#11297=ORIENTED_EDGE('',*,*,#8449,.F.);
#11298=ORIENTED_EDGE('',*,*,#8454,.T.);
#11299=ORIENTED_EDGE('',*,*,#8455,.T.);
#11300=ORIENTED_EDGE('',*,*,#8456,.F.);
#11301=ORIENTED_EDGE('',*,*,#8452,.F.);
#11302=ORIENTED_EDGE('',*,*,#8457,.T.);
#11303=ORIENTED_EDGE('',*,*,#8458,.T.);
#11304=ORIENTED_EDGE('',*,*,#8459,.F.);
#11305=ORIENTED_EDGE('',*,*,#8455,.F.);
#11306=ORIENTED_EDGE('',*,*,#8460,.T.);
#11307=ORIENTED_EDGE('',*,*,#8461,.T.);
#11308=ORIENTED_EDGE('',*,*,#8462,.F.);
#11309=ORIENTED_EDGE('',*,*,#8458,.F.);
#11310=ORIENTED_EDGE('',*,*,#8463,.T.);
#11311=ORIENTED_EDGE('',*,*,#8464,.T.);
#11312=ORIENTED_EDGE('',*,*,#8465,.F.);
#11313=ORIENTED_EDGE('',*,*,#8461,.F.);
#11314=ORIENTED_EDGE('',*,*,#8466,.T.);
#11315=ORIENTED_EDGE('',*,*,#8467,.T.);
#11316=ORIENTED_EDGE('',*,*,#8468,.F.);
#11317=ORIENTED_EDGE('',*,*,#8464,.F.);
#11318=ORIENTED_EDGE('',*,*,#8469,.T.);
#11319=ORIENTED_EDGE('',*,*,#8470,.T.);
#11320=ORIENTED_EDGE('',*,*,#8471,.F.);
#11321=ORIENTED_EDGE('',*,*,#8467,.F.);
#11322=ORIENTED_EDGE('',*,*,#8472,.T.);
#11323=ORIENTED_EDGE('',*,*,#8473,.F.);
#11324=ORIENTED_EDGE('',*,*,#8474,.T.);
#11325=ORIENTED_EDGE('',*,*,#8475,.F.);
#11326=ORIENTED_EDGE('',*,*,#8476,.F.);
#11327=ORIENTED_EDGE('',*,*,#8477,.T.);
#11328=ORIENTED_EDGE('',*,*,#8478,.T.);
#11329=ORIENTED_EDGE('',*,*,#8479,.T.);
#11330=ORIENTED_EDGE('',*,*,#8480,.T.);
#11331=ORIENTED_EDGE('',*,*,#8481,.F.);
#11332=ORIENTED_EDGE('',*,*,#8482,.T.);
#11333=ORIENTED_EDGE('',*,*,#8483,.T.);
#11334=ORIENTED_EDGE('',*,*,#8477,.F.);
#11335=ORIENTED_EDGE('',*,*,#8484,.T.);
#11336=ORIENTED_EDGE('',*,*,#8485,.T.);
#11337=ORIENTED_EDGE('',*,*,#8486,.F.);
#11338=ORIENTED_EDGE('',*,*,#8480,.F.);
#11339=ORIENTED_EDGE('',*,*,#8487,.T.);
#11340=ORIENTED_EDGE('',*,*,#8488,.T.);
#11341=ORIENTED_EDGE('',*,*,#8489,.F.);
#11342=ORIENTED_EDGE('',*,*,#8485,.F.);
#11343=ORIENTED_EDGE('',*,*,#8490,.T.);
#11344=ORIENTED_EDGE('',*,*,#8491,.T.);
#11345=ORIENTED_EDGE('',*,*,#8492,.F.);
#11346=ORIENTED_EDGE('',*,*,#8488,.F.);
#11347=ORIENTED_EDGE('',*,*,#8493,.T.);
#11348=ORIENTED_EDGE('',*,*,#8494,.T.);
#11349=ORIENTED_EDGE('',*,*,#8495,.F.);
#11350=ORIENTED_EDGE('',*,*,#8491,.F.);
#11351=ORIENTED_EDGE('',*,*,#8496,.T.);
#11352=ORIENTED_EDGE('',*,*,#8497,.T.);
#11353=ORIENTED_EDGE('',*,*,#8498,.F.);
#11354=ORIENTED_EDGE('',*,*,#8494,.F.);
#11355=ORIENTED_EDGE('',*,*,#8499,.T.);
#11356=ORIENTED_EDGE('',*,*,#8500,.T.);
#11357=ORIENTED_EDGE('',*,*,#8501,.F.);
#11358=ORIENTED_EDGE('',*,*,#8497,.F.);
#11359=ORIENTED_EDGE('',*,*,#8502,.T.);
#11360=ORIENTED_EDGE('',*,*,#8503,.T.);
#11361=ORIENTED_EDGE('',*,*,#8504,.F.);
#11362=ORIENTED_EDGE('',*,*,#8500,.F.);
#11363=ORIENTED_EDGE('',*,*,#8505,.T.);
#11364=ORIENTED_EDGE('',*,*,#8506,.T.);
#11365=ORIENTED_EDGE('',*,*,#8507,.F.);
#11366=ORIENTED_EDGE('',*,*,#8503,.F.);
#11367=ORIENTED_EDGE('',*,*,#8508,.T.);
#11368=ORIENTED_EDGE('',*,*,#8509,.T.);
#11369=ORIENTED_EDGE('',*,*,#8510,.F.);
#11370=ORIENTED_EDGE('',*,*,#8506,.F.);
#11371=ORIENTED_EDGE('',*,*,#8511,.T.);
#11372=ORIENTED_EDGE('',*,*,#8512,.T.);
#11373=ORIENTED_EDGE('',*,*,#8513,.F.);
#11374=ORIENTED_EDGE('',*,*,#8509,.F.);
#11375=ORIENTED_EDGE('',*,*,#8514,.T.);
#11376=ORIENTED_EDGE('',*,*,#8515,.T.);
#11377=ORIENTED_EDGE('',*,*,#8516,.F.);
#11378=ORIENTED_EDGE('',*,*,#8512,.F.);
#11379=ORIENTED_EDGE('',*,*,#8517,.T.);
#11380=ORIENTED_EDGE('',*,*,#8518,.T.);
#11381=ORIENTED_EDGE('',*,*,#8519,.F.);
#11382=ORIENTED_EDGE('',*,*,#8515,.F.);
#11383=ORIENTED_EDGE('',*,*,#8520,.T.);
#11384=ORIENTED_EDGE('',*,*,#8521,.T.);
#11385=ORIENTED_EDGE('',*,*,#8522,.F.);
#11386=ORIENTED_EDGE('',*,*,#8518,.F.);
#11387=ORIENTED_EDGE('',*,*,#8523,.T.);
#11388=ORIENTED_EDGE('',*,*,#8524,.T.);
#11389=ORIENTED_EDGE('',*,*,#8525,.F.);
#11390=ORIENTED_EDGE('',*,*,#8521,.F.);
#11391=ORIENTED_EDGE('',*,*,#8526,.T.);
#11392=ORIENTED_EDGE('',*,*,#8527,.T.);
#11393=ORIENTED_EDGE('',*,*,#8528,.F.);
#11394=ORIENTED_EDGE('',*,*,#8524,.F.);
#11395=ORIENTED_EDGE('',*,*,#8529,.T.);
#11396=ORIENTED_EDGE('',*,*,#8530,.T.);
#11397=ORIENTED_EDGE('',*,*,#8531,.F.);
#11398=ORIENTED_EDGE('',*,*,#8527,.F.);
#11399=ORIENTED_EDGE('',*,*,#8532,.T.);
#11400=ORIENTED_EDGE('',*,*,#8533,.T.);
#11401=ORIENTED_EDGE('',*,*,#8534,.F.);
#11402=ORIENTED_EDGE('',*,*,#8530,.F.);
#11403=ORIENTED_EDGE('',*,*,#8535,.T.);
#11404=ORIENTED_EDGE('',*,*,#8536,.T.);
#11405=ORIENTED_EDGE('',*,*,#8537,.F.);
#11406=ORIENTED_EDGE('',*,*,#8533,.F.);
#11407=ORIENTED_EDGE('',*,*,#8538,.T.);
#11408=ORIENTED_EDGE('',*,*,#8539,.T.);
#11409=ORIENTED_EDGE('',*,*,#8540,.F.);
#11410=ORIENTED_EDGE('',*,*,#8536,.F.);
#11411=ORIENTED_EDGE('',*,*,#8541,.T.);
#11412=ORIENTED_EDGE('',*,*,#8542,.T.);
#11413=ORIENTED_EDGE('',*,*,#8543,.F.);
#11414=ORIENTED_EDGE('',*,*,#8539,.F.);
#11415=ORIENTED_EDGE('',*,*,#8544,.T.);
#11416=ORIENTED_EDGE('',*,*,#8545,.T.);
#11417=ORIENTED_EDGE('',*,*,#8546,.F.);
#11418=ORIENTED_EDGE('',*,*,#8542,.F.);
#11419=ORIENTED_EDGE('',*,*,#8547,.T.);
#11420=ORIENTED_EDGE('',*,*,#8548,.T.);
#11421=ORIENTED_EDGE('',*,*,#8549,.F.);
#11422=ORIENTED_EDGE('',*,*,#8545,.F.);
#11423=ORIENTED_EDGE('',*,*,#8550,.T.);
#11424=ORIENTED_EDGE('',*,*,#8551,.F.);
#11425=ORIENTED_EDGE('',*,*,#8552,.T.);
#11426=ORIENTED_EDGE('',*,*,#8553,.T.);
#11427=ORIENTED_EDGE('',*,*,#8554,.F.);
#11428=ORIENTED_EDGE('',*,*,#8483,.F.);
#11429=ORIENTED_EDGE('',*,*,#8478,.F.);
#11430=ORIENTED_EDGE('',*,*,#8555,.T.);
#11431=ORIENTED_EDGE('',*,*,#8556,.T.);
#11432=ORIENTED_EDGE('',*,*,#8555,.F.);
#11433=ORIENTED_EDGE('',*,*,#8557,.F.);
#11434=ORIENTED_EDGE('',*,*,#8558,.T.);
#11435=ORIENTED_EDGE('',*,*,#8559,.F.);
#11436=ORIENTED_EDGE('',*,*,#8560,.F.);
#11437=ORIENTED_EDGE('',*,*,#8561,.F.);
#11438=ORIENTED_EDGE('',*,*,#8562,.T.);
#11439=ORIENTED_EDGE('',*,*,#8563,.T.);
#11440=ORIENTED_EDGE('',*,*,#8562,.F.);
#11441=ORIENTED_EDGE('',*,*,#8564,.F.);
#11442=ORIENTED_EDGE('',*,*,#8565,.F.);
#11443=ORIENTED_EDGE('',*,*,#8566,.F.);
#11444=ORIENTED_EDGE('',*,*,#8558,.F.);
#11445=ORIENTED_EDGE('',*,*,#8567,.F.);
#11446=ORIENTED_EDGE('',*,*,#8568,.T.);
#11447=ORIENTED_EDGE('',*,*,#8569,.T.);
#11448=ORIENTED_EDGE('',*,*,#8568,.F.);
#11449=ORIENTED_EDGE('',*,*,#8570,.F.);
#11450=ORIENTED_EDGE('',*,*,#8571,.T.);
#11451=ORIENTED_EDGE('',*,*,#8572,.T.);
#11452=ORIENTED_EDGE('',*,*,#8573,.F.);
#11453=ORIENTED_EDGE('',*,*,#8574,.F.);
#11454=ORIENTED_EDGE('',*,*,#8575,.T.);
#11455=ORIENTED_EDGE('',*,*,#8567,.T.);
#11456=ORIENTED_EDGE('',*,*,#8575,.F.);
#11457=ORIENTED_EDGE('',*,*,#8576,.F.);
#11458=ORIENTED_EDGE('',*,*,#8577,.F.);
#11459=ORIENTED_EDGE('',*,*,#8578,.T.);
#11460=ORIENTED_EDGE('',*,*,#8571,.F.);
#11461=ORIENTED_EDGE('',*,*,#8579,.F.);
#11462=ORIENTED_EDGE('',*,*,#8580,.T.);
#11463=ORIENTED_EDGE('',*,*,#8581,.T.);
#11464=ORIENTED_EDGE('',*,*,#8580,.F.);
#11465=ORIENTED_EDGE('',*,*,#8582,.F.);
#11466=ORIENTED_EDGE('',*,*,#8583,.T.);
#11467=ORIENTED_EDGE('',*,*,#8579,.T.);
#11468=ORIENTED_EDGE('',*,*,#8583,.F.);
#11469=ORIENTED_EDGE('',*,*,#8584,.F.);
#11470=ORIENTED_EDGE('',*,*,#8585,.T.);
#11471=ORIENTED_EDGE('',*,*,#8586,.T.);
#11472=ORIENTED_EDGE('',*,*,#8585,.F.);
#11473=ORIENTED_EDGE('',*,*,#8551,.T.);
#11474=ORIENTED_EDGE('',*,*,#8587,.F.);
#11475=ORIENTED_EDGE('',*,*,#8548,.F.);
#11476=ORIENTED_EDGE('',*,*,#8588,.T.);
#11477=ORIENTED_EDGE('',*,*,#8557,.T.);
#11478=ORIENTED_EDGE('',*,*,#8553,.F.);
#11479=ORIENTED_EDGE('',*,*,#8589,.T.);
#11480=ORIENTED_EDGE('',*,*,#8475,.T.);
#11481=ORIENTED_EDGE('',*,*,#8590,.T.);
#11482=ORIENTED_EDGE('',*,*,#8584,.T.);
#11483=ORIENTED_EDGE('',*,*,#8563,.F.);
#11484=ORIENTED_EDGE('',*,*,#8582,.T.);
#11485=ORIENTED_EDGE('',*,*,#8586,.F.);
#11486=ORIENTED_EDGE('',*,*,#8581,.F.);
#11487=ORIENTED_EDGE('',*,*,#8570,.T.);
#11488=ORIENTED_EDGE('',*,*,#8569,.F.);
#11489=ORIENTED_EDGE('',*,*,#8556,.F.);
#11490=ORIENTED_EDGE('',*,*,#8565,.T.);
#11491=ORIENTED_EDGE('',*,*,#8591,.T.);
#11492=ORIENTED_EDGE('',*,*,#8577,.T.);
#11493=ORIENTED_EDGE('',*,*,#8592,.F.);
#11494=ORIENTED_EDGE('',*,*,#8559,.T.);
#11495=ORIENTED_EDGE('',*,*,#8566,.T.);
#11496=ORIENTED_EDGE('',*,*,#8592,.T.);
#11497=ORIENTED_EDGE('',*,*,#8576,.T.);
#11498=ORIENTED_EDGE('',*,*,#8574,.T.);
#11499=ORIENTED_EDGE('',*,*,#8593,.F.);
#11500=ORIENTED_EDGE('',*,*,#8560,.T.);
#11501=ORIENTED_EDGE('',*,*,#8593,.T.);
#11502=ORIENTED_EDGE('',*,*,#8573,.T.);
#11503=ORIENTED_EDGE('',*,*,#8594,.F.);
#11504=ORIENTED_EDGE('',*,*,#8564,.T.);
#11505=ORIENTED_EDGE('',*,*,#8561,.T.);
#11506=ORIENTED_EDGE('',*,*,#8594,.T.);
#11507=ORIENTED_EDGE('',*,*,#8572,.F.);
#11508=ORIENTED_EDGE('',*,*,#8578,.F.);
#11509=ORIENTED_EDGE('',*,*,#8591,.F.);
#11510=ORIENTED_EDGE('',*,*,#8402,.F.);
#11511=ORIENTED_EDGE('',*,*,#8595,.F.);
#11512=ORIENTED_EDGE('',*,*,#8482,.F.);
#11513=ORIENTED_EDGE('',*,*,#8596,.F.);
#11514=ORIENTED_EDGE('',*,*,#8473,.T.);
#11515=ORIENTED_EDGE('',*,*,#8597,.F.);
#11516=ORIENTED_EDGE('',*,*,#8470,.F.);
#11517=ORIENTED_EDGE('',*,*,#8598,.T.);
#11518=ORIENTED_EDGE('',*,*,#8479,.F.);
#11519=ORIENTED_EDGE('',*,*,#8595,.T.);
#11520=ORIENTED_EDGE('',*,*,#8401,.T.);
#11521=ORIENTED_EDGE('',*,*,#8405,.T.);
#11522=ORIENTED_EDGE('',*,*,#8408,.T.);
#11523=ORIENTED_EDGE('',*,*,#8411,.T.);
#11524=ORIENTED_EDGE('',*,*,#8414,.T.);
#11525=ORIENTED_EDGE('',*,*,#8417,.T.);
#11526=ORIENTED_EDGE('',*,*,#8420,.T.);
#11527=ORIENTED_EDGE('',*,*,#8423,.T.);
#11528=ORIENTED_EDGE('',*,*,#8426,.T.);
#11529=ORIENTED_EDGE('',*,*,#8429,.T.);
#11530=ORIENTED_EDGE('',*,*,#8432,.T.);
#11531=ORIENTED_EDGE('',*,*,#8435,.T.);
#11532=ORIENTED_EDGE('',*,*,#8438,.T.);
#11533=ORIENTED_EDGE('',*,*,#8441,.T.);
#11534=ORIENTED_EDGE('',*,*,#8444,.T.);
#11535=ORIENTED_EDGE('',*,*,#8447,.T.);
#11536=ORIENTED_EDGE('',*,*,#8450,.T.);
#11537=ORIENTED_EDGE('',*,*,#8453,.T.);
#11538=ORIENTED_EDGE('',*,*,#8456,.T.);
#11539=ORIENTED_EDGE('',*,*,#8459,.T.);
#11540=ORIENTED_EDGE('',*,*,#8462,.T.);
#11541=ORIENTED_EDGE('',*,*,#8465,.T.);
#11542=ORIENTED_EDGE('',*,*,#8468,.T.);
#11543=ORIENTED_EDGE('',*,*,#8471,.T.);
#11544=ORIENTED_EDGE('',*,*,#8597,.T.);
#11545=ORIENTED_EDGE('',*,*,#8476,.T.);
#11546=ORIENTED_EDGE('',*,*,#8589,.F.);
#11547=ORIENTED_EDGE('',*,*,#8552,.F.);
#11548=ORIENTED_EDGE('',*,*,#8588,.F.);
#11549=ORIENTED_EDGE('',*,*,#8550,.F.);
#11550=ORIENTED_EDGE('',*,*,#8547,.F.);
#11551=ORIENTED_EDGE('',*,*,#8544,.F.);
#11552=ORIENTED_EDGE('',*,*,#8541,.F.);
#11553=ORIENTED_EDGE('',*,*,#8538,.F.);
#11554=ORIENTED_EDGE('',*,*,#8535,.F.);
#11555=ORIENTED_EDGE('',*,*,#8532,.F.);
#11556=ORIENTED_EDGE('',*,*,#8529,.F.);
#11557=ORIENTED_EDGE('',*,*,#8526,.F.);
#11558=ORIENTED_EDGE('',*,*,#8523,.F.);
#11559=ORIENTED_EDGE('',*,*,#8520,.F.);
#11560=ORIENTED_EDGE('',*,*,#8517,.F.);
#11561=ORIENTED_EDGE('',*,*,#8514,.F.);
#11562=ORIENTED_EDGE('',*,*,#8511,.F.);
#11563=ORIENTED_EDGE('',*,*,#8508,.F.);
#11564=ORIENTED_EDGE('',*,*,#8505,.F.);
#11565=ORIENTED_EDGE('',*,*,#8502,.F.);
#11566=ORIENTED_EDGE('',*,*,#8499,.F.);
#11567=ORIENTED_EDGE('',*,*,#8496,.F.);
#11568=ORIENTED_EDGE('',*,*,#8493,.F.);
#11569=ORIENTED_EDGE('',*,*,#8490,.F.);
#11570=ORIENTED_EDGE('',*,*,#8487,.F.);
#11571=ORIENTED_EDGE('',*,*,#8484,.F.);
#11572=ORIENTED_EDGE('',*,*,#8403,.F.);
#11573=ORIENTED_EDGE('',*,*,#8596,.T.);
#11574=ORIENTED_EDGE('',*,*,#8481,.T.);
#11575=ORIENTED_EDGE('',*,*,#8486,.T.);
#11576=ORIENTED_EDGE('',*,*,#8489,.T.);
#11577=ORIENTED_EDGE('',*,*,#8492,.T.);
#11578=ORIENTED_EDGE('',*,*,#8495,.T.);
#11579=ORIENTED_EDGE('',*,*,#8498,.T.);
#11580=ORIENTED_EDGE('',*,*,#8501,.T.);
#11581=ORIENTED_EDGE('',*,*,#8504,.T.);
#11582=ORIENTED_EDGE('',*,*,#8507,.T.);
#11583=ORIENTED_EDGE('',*,*,#8510,.T.);
#11584=ORIENTED_EDGE('',*,*,#8513,.T.);
#11585=ORIENTED_EDGE('',*,*,#8516,.T.);
#11586=ORIENTED_EDGE('',*,*,#8519,.T.);
#11587=ORIENTED_EDGE('',*,*,#8522,.T.);
#11588=ORIENTED_EDGE('',*,*,#8525,.T.);
#11589=ORIENTED_EDGE('',*,*,#8528,.T.);
#11590=ORIENTED_EDGE('',*,*,#8531,.T.);
#11591=ORIENTED_EDGE('',*,*,#8534,.T.);
#11592=ORIENTED_EDGE('',*,*,#8537,.T.);
#11593=ORIENTED_EDGE('',*,*,#8540,.T.);
#11594=ORIENTED_EDGE('',*,*,#8543,.T.);
#11595=ORIENTED_EDGE('',*,*,#8546,.T.);
#11596=ORIENTED_EDGE('',*,*,#8549,.T.);
#11597=ORIENTED_EDGE('',*,*,#8587,.T.);
#11598=ORIENTED_EDGE('',*,*,#8554,.T.);
#11599=ORIENTED_EDGE('',*,*,#8590,.F.);
#11600=ORIENTED_EDGE('',*,*,#8474,.F.);
#11601=ORIENTED_EDGE('',*,*,#8598,.F.);
#11602=ORIENTED_EDGE('',*,*,#8472,.F.);
#11603=ORIENTED_EDGE('',*,*,#8469,.F.);
#11604=ORIENTED_EDGE('',*,*,#8466,.F.);
#11605=ORIENTED_EDGE('',*,*,#8463,.F.);
#11606=ORIENTED_EDGE('',*,*,#8460,.F.);
#11607=ORIENTED_EDGE('',*,*,#8457,.F.);
#11608=ORIENTED_EDGE('',*,*,#8454,.F.);
#11609=ORIENTED_EDGE('',*,*,#8451,.F.);
#11610=ORIENTED_EDGE('',*,*,#8448,.F.);
#11611=ORIENTED_EDGE('',*,*,#8445,.F.);
#11612=ORIENTED_EDGE('',*,*,#8442,.F.);
#11613=ORIENTED_EDGE('',*,*,#8439,.F.);
#11614=ORIENTED_EDGE('',*,*,#8436,.F.);
#11615=ORIENTED_EDGE('',*,*,#8433,.F.);
#11616=ORIENTED_EDGE('',*,*,#8430,.F.);
#11617=ORIENTED_EDGE('',*,*,#8427,.F.);
#11618=ORIENTED_EDGE('',*,*,#8424,.F.);
#11619=ORIENTED_EDGE('',*,*,#8421,.F.);
#11620=ORIENTED_EDGE('',*,*,#8418,.F.);
#11621=ORIENTED_EDGE('',*,*,#8415,.F.);
#11622=ORIENTED_EDGE('',*,*,#8412,.F.);
#11623=ORIENTED_EDGE('',*,*,#8409,.F.);
#11624=ORIENTED_EDGE('',*,*,#8406,.F.);
#16267=CYLINDRICAL_SURFACE('',#17910,4.29685191531258);
#16268=CYLINDRICAL_SURFACE('',#17911,4.29685191531258);
#16269=CYLINDRICAL_SURFACE('',#17912,4.29685191531258);
#16270=CYLINDRICAL_SURFACE('',#17913,4.29685191531258);
#16271=CYLINDRICAL_SURFACE('',#17914,4.29685191531258);
#16272=CYLINDRICAL_SURFACE('',#17915,4.29685191531258);
#16273=CYLINDRICAL_SURFACE('',#17916,4.29685191531258);
#16274=CYLINDRICAL_SURFACE('',#17917,4.29685191531258);
#16275=CYLINDRICAL_SURFACE('',#17918,4.29685191531258);
#16276=CYLINDRICAL_SURFACE('',#17919,4.29685191531258);
#16277=CYLINDRICAL_SURFACE('',#17920,4.29685191531258);
#16278=CYLINDRICAL_SURFACE('',#17921,4.29685191531258);
#16279=CYLINDRICAL_SURFACE('',#17922,4.29685191531258);
#16280=CYLINDRICAL_SURFACE('',#17923,4.29685191531258);
#16281=CYLINDRICAL_SURFACE('',#17924,4.29685191531258);
#16282=CYLINDRICAL_SURFACE('',#17925,4.29685191531258);
#16283=CYLINDRICAL_SURFACE('',#17926,4.29685191531258);
#16284=CYLINDRICAL_SURFACE('',#17927,4.29685191531258);
#16285=CYLINDRICAL_SURFACE('',#17928,4.29685191531258);
#16286=CYLINDRICAL_SURFACE('',#17929,4.29685191531258);
#16287=CYLINDRICAL_SURFACE('',#17930,4.29685191531258);
#16288=CYLINDRICAL_SURFACE('',#17931,4.29685191531258);
#16289=CYLINDRICAL_SURFACE('',#17932,4.29685191531258);
#16290=CYLINDRICAL_SURFACE('',#17933,4.29685191531258);
#16291=CYLINDRICAL_SURFACE('',#17934,4.29685191531258);
#16292=CYLINDRICAL_SURFACE('',#17936,4.12499999999999);
#16293=CYLINDRICAL_SURFACE('',#17938,4.12499999999999);
#16294=CYLINDRICAL_SURFACE('',#17940,4.12499999999999);
#16295=CYLINDRICAL_SURFACE('',#17941,4.12499999999999);
#16296=CYLINDRICAL_SURFACE('',#17942,4.12499999999999);
#16297=CYLINDRICAL_SURFACE('',#17943,4.12499999999999);
#16298=CYLINDRICAL_SURFACE('',#17944,4.12499999999999);
#16299=CYLINDRICAL_SURFACE('',#17945,4.12499999999999);
#16300=CYLINDRICAL_SURFACE('',#17946,4.12499999999999);
#16301=CYLINDRICAL_SURFACE('',#17947,4.12499999999999);
#16302=CYLINDRICAL_SURFACE('',#17948,4.12499999999999);
#16303=CYLINDRICAL_SURFACE('',#17949,4.12499999999999);
#16304=CYLINDRICAL_SURFACE('',#17950,4.12499999999999);
#16305=CYLINDRICAL_SURFACE('',#17951,4.12499999999999);
#16306=CYLINDRICAL_SURFACE('',#17952,4.12499999999999);
#16307=CYLINDRICAL_SURFACE('',#17953,4.12499999999999);
#16308=CYLINDRICAL_SURFACE('',#17954,4.12499999999999);
#16309=CYLINDRICAL_SURFACE('',#17955,4.12499999999999);
#16310=CYLINDRICAL_SURFACE('',#17956,4.12499999999999);
#16311=CYLINDRICAL_SURFACE('',#17957,4.12499999999999);
#16312=CYLINDRICAL_SURFACE('',#17958,4.12499999999999);
#16313=CYLINDRICAL_SURFACE('',#17959,4.12499999999999);
#16314=CYLINDRICAL_SURFACE('',#17960,4.12499999999999);
#16315=CYLINDRICAL_SURFACE('',#17961,4.12499999999999);
#16316=CYLINDRICAL_SURFACE('',#17962,4.12499999999999);
#16317=CYLINDRICAL_SURFACE('',#17966,8.);
#16318=CYLINDRICAL_SURFACE('',#17977,12.5);
#16319=CYLINDRICAL_SURFACE('',#17987,25.);
#16320=CYLINDRICAL_SURFACE('',#17989,22.5);
#16321=CYLINDRICAL_SURFACE('',#17992,4.12499999999999);
#16322=CYLINDRICAL_SURFACE('',#18001,4.29685191531258);
#16671=ADVANCED_FACE('',(#1712),#16267,.F.);
#16672=ADVANCED_FACE('',(#1713),#16268,.F.);
#16673=ADVANCED_FACE('',(#1714),#16269,.F.);
#16674=ADVANCED_FACE('',(#1715),#16270,.F.);
#16675=ADVANCED_FACE('',(#1716),#16271,.F.);
#16676=ADVANCED_FACE('',(#1717),#16272,.F.);
#16677=ADVANCED_FACE('',(#1718),#16273,.F.);
#16678=ADVANCED_FACE('',(#1719),#16274,.F.);
#16679=ADVANCED_FACE('',(#1720),#16275,.F.);
#16680=ADVANCED_FACE('',(#1721),#16276,.F.);
#16681=ADVANCED_FACE('',(#1722),#16277,.F.);
#16682=ADVANCED_FACE('',(#1723),#16278,.F.);
#16683=ADVANCED_FACE('',(#1724),#16279,.F.);
#16684=ADVANCED_FACE('',(#1725),#16280,.F.);
#16685=ADVANCED_FACE('',(#1726),#16281,.F.);
#16686=ADVANCED_FACE('',(#1727),#16282,.F.);
#16687=ADVANCED_FACE('',(#1728),#16283,.F.);
#16688=ADVANCED_FACE('',(#1729),#16284,.F.);
#16689=ADVANCED_FACE('',(#1730),#16285,.F.);
#16690=ADVANCED_FACE('',(#1731),#16286,.F.);
#16691=ADVANCED_FACE('',(#1732),#16287,.F.);
#16692=ADVANCED_FACE('',(#1733),#16288,.F.);
#16693=ADVANCED_FACE('',(#1734),#16289,.F.);
#16694=ADVANCED_FACE('',(#1735),#16290,.F.);
#16695=ADVANCED_FACE('',(#1736),#16291,.F.);
#16696=ADVANCED_FACE('',(#1737),#16292,.F.);
#16697=ADVANCED_FACE('',(#1738),#16293,.F.);
#16698=ADVANCED_FACE('',(#1739),#16294,.F.);
#16699=ADVANCED_FACE('',(#1740),#16295,.F.);
#16700=ADVANCED_FACE('',(#1741),#16296,.F.);
#16701=ADVANCED_FACE('',(#1742),#16297,.F.);
#16702=ADVANCED_FACE('',(#1743),#16298,.F.);
#16703=ADVANCED_FACE('',(#1744),#16299,.F.);
#16704=ADVANCED_FACE('',(#1745),#16300,.F.);
#16705=ADVANCED_FACE('',(#1746),#16301,.F.);
#16706=ADVANCED_FACE('',(#1747),#16302,.F.);
#16707=ADVANCED_FACE('',(#1748),#16303,.F.);
#16708=ADVANCED_FACE('',(#1749),#16304,.F.);
#16709=ADVANCED_FACE('',(#1750),#16305,.F.);
#16710=ADVANCED_FACE('',(#1751),#16306,.F.);
#16711=ADVANCED_FACE('',(#1752),#16307,.F.);
#16712=ADVANCED_FACE('',(#1753),#16308,.F.);
#16713=ADVANCED_FACE('',(#1754),#16309,.F.);
#16714=ADVANCED_FACE('',(#1755),#16310,.F.);
#16715=ADVANCED_FACE('',(#1756),#16311,.F.);
#16716=ADVANCED_FACE('',(#1757),#16312,.F.);
#16717=ADVANCED_FACE('',(#1758),#16313,.F.);
#16718=ADVANCED_FACE('',(#1759),#16314,.F.);
#16719=ADVANCED_FACE('',(#1760),#16315,.F.);
#16720=ADVANCED_FACE('',(#1761),#16316,.F.);
#16721=ADVANCED_FACE('',(#1762),#1022,.F.);
#16722=ADVANCED_FACE('',(#1763),#16317,.F.);
#16723=ADVANCED_FACE('',(#1764),#140,.T.);
#16724=ADVANCED_FACE('',(#1765),#16318,.T.);
#16725=ADVANCED_FACE('',(#1766),#141,.T.);
#16726=ADVANCED_FACE('',(#1767),#16319,.T.);
#16727=ADVANCED_FACE('',(#1768),#16320,.F.);
#16728=ADVANCED_FACE('',(#1769),#16321,.F.);
#16729=ADVANCED_FACE('',(#1770,#864),#1237,.T.);
#16730=ADVANCED_FACE('',(#1771,#865),#1238,.T.);
#16731=ADVANCED_FACE('',(#1772,#866),#1239,.T.);
#16732=ADVANCED_FACE('',(#1773,#867),#1240,.T.);
#16733=ADVANCED_FACE('',(#1774,#868),#1241,.T.);
#16734=ADVANCED_FACE('',(#1775),#138,.F.);
#16735=ADVANCED_FACE('',(#1776),#1242,.F.);
#16736=ADVANCED_FACE('',(#1777),#139,.F.);
#16737=ADVANCED_FACE('',(#1778),#1243,.T.);
#16738=ADVANCED_FACE('',(#1779),#1244,.F.);
#16739=ADVANCED_FACE('',(#1780),#16322,.F.);
#16740=ADVANCED_FACE('',(#1781),#124,.T.);
#16741=ADVANCED_FACE('',(#1782),#125,.T.);
#17614=CLOSED_SHELL('',(#16671,#16672,#16673,#16674,#16675,#16676,#16677,
#16678,#16679,#16680,#16681,#16682,#16683,#16684,#16685,#16686,#16687,#16688,
#16689,#16690,#16691,#16692,#16693,#16694,#16695,#16696,#16697,#16698,#16699,
#16700,#16701,#16702,#16703,#16704,#16705,#16706,#16707,#16708,#16709,#16710,
#16711,#16712,#16713,#16714,#16715,#16716,#16717,#16718,#16719,#16720,#16721,
#16722,#16723,#16724,#16725,#16726,#16727,#16728,#16729,#16730,#16731,#16732,
#16733,#16734,#16735,#16736,#16737,#16738,#16739,#16740,#16741));
#17909=AXIS2_PLACEMENT_3D('',#24971,#20097,#20098);
#17910=AXIS2_PLACEMENT_3D('',#24972,#20099,#20100);
#17911=AXIS2_PLACEMENT_3D('',#24993,#20103,#20104);
#17912=AXIS2_PLACEMENT_3D('',#25023,#20106,#20107);
#17913=AXIS2_PLACEMENT_3D('',#25053,#20109,#20110);
#17914=AXIS2_PLACEMENT_3D('',#25083,#20112,#20113);
#17915=AXIS2_PLACEMENT_3D('',#25113,#20115,#20116);
#17916=AXIS2_PLACEMENT_3D('',#25143,#20118,#20119);
#17917=AXIS2_PLACEMENT_3D('',#25173,#20121,#20122);
#17918=AXIS2_PLACEMENT_3D('',#25203,#20124,#20125);
#17919=AXIS2_PLACEMENT_3D('',#25233,#20127,#20128);
#17920=AXIS2_PLACEMENT_3D('',#25263,#20130,#20131);
#17921=AXIS2_PLACEMENT_3D('',#25293,#20133,#20134);
#17922=AXIS2_PLACEMENT_3D('',#25323,#20136,#20137);
#17923=AXIS2_PLACEMENT_3D('',#25353,#20139,#20140);
#17924=AXIS2_PLACEMENT_3D('',#25383,#20142,#20143);
#17925=AXIS2_PLACEMENT_3D('',#25413,#20145,#20146);
#17926=AXIS2_PLACEMENT_3D('',#25443,#20148,#20149);
#17927=AXIS2_PLACEMENT_3D('',#25473,#20151,#20152);
#17928=AXIS2_PLACEMENT_3D('',#25503,#20154,#20155);
#17929=AXIS2_PLACEMENT_3D('',#25533,#20157,#20158);
#17930=AXIS2_PLACEMENT_3D('',#25563,#20160,#20161);
#17931=AXIS2_PLACEMENT_3D('',#25593,#20163,#20164);
#17932=AXIS2_PLACEMENT_3D('',#25623,#20166,#20167);
#17933=AXIS2_PLACEMENT_3D('',#25653,#20169,#20170);
#17934=AXIS2_PLACEMENT_3D('',#25683,#20172,#20173);
#17935=AXIS2_PLACEMENT_3D('',#25694,#20175,#20176);
#17936=AXIS2_PLACEMENT_3D('',#25700,#20177,#20178);
#17937=AXIS2_PLACEMENT_3D('',#25705,#20180,#20181);
#17938=AXIS2_PLACEMENT_3D('',#25742,#20182,#20183);
#17939=AXIS2_PLACEMENT_3D('',#25784,#20186,#20187);
#17940=AXIS2_PLACEMENT_3D('',#25823,#20188,#20189);
#17941=AXIS2_PLACEMENT_3D('',#25899,#20191,#20192);
#17942=AXIS2_PLACEMENT_3D('',#25975,#20194,#20195);
#17943=AXIS2_PLACEMENT_3D('',#26051,#20197,#20198);
#17944=AXIS2_PLACEMENT_3D('',#26127,#20200,#20201);
#17945=AXIS2_PLACEMENT_3D('',#26205,#20203,#20204);
#17946=AXIS2_PLACEMENT_3D('',#26283,#20206,#20207);
#17947=AXIS2_PLACEMENT_3D('',#26359,#20209,#20210);
#17948=AXIS2_PLACEMENT_3D('',#26435,#20212,#20213);
#17949=AXIS2_PLACEMENT_3D('',#26511,#20215,#20216);
#17950=AXIS2_PLACEMENT_3D('',#26587,#20218,#20219);
#17951=AXIS2_PLACEMENT_3D('',#26667,#20221,#20222);
#17952=AXIS2_PLACEMENT_3D('',#26743,#20224,#20225);
#17953=AXIS2_PLACEMENT_3D('',#26819,#20227,#20228);
#17954=AXIS2_PLACEMENT_3D('',#26895,#20230,#20231);
#17955=AXIS2_PLACEMENT_3D('',#26971,#20233,#20234);
#17956=AXIS2_PLACEMENT_3D('',#27047,#20236,#20237);
#17957=AXIS2_PLACEMENT_3D('',#27127,#20239,#20240);
#17958=AXIS2_PLACEMENT_3D('',#27203,#20242,#20243);
#17959=AXIS2_PLACEMENT_3D('',#27279,#20245,#20246);
#17960=AXIS2_PLACEMENT_3D('',#27355,#20248,#20249);
#17961=AXIS2_PLACEMENT_3D('',#27431,#20251,#20252);
#17962=AXIS2_PLACEMENT_3D('',#27507,#20254,#20255);
#17963=AXIS2_PLACEMENT_3D('',#27521,#20257,#20258);
#17964=AXIS2_PLACEMENT_3D('',#27538,#20259,#20260);
#17965=AXIS2_PLACEMENT_3D('',#27541,#20262,#20263);
#17966=AXIS2_PLACEMENT_3D('',#27542,#20264,#20265);
#17967=AXIS2_PLACEMENT_3D('',#27544,#20266,#20267);
#17968=AXIS2_PLACEMENT_3D('',#27548,#20269,#20270);
#17969=AXIS2_PLACEMENT_3D('',#27585,#20271,#20272);
#17970=AXIS2_PLACEMENT_3D('',#27588,#20274,#20275);
#17971=AXIS2_PLACEMENT_3D('',#27590,#20276,#20277);
#17972=AXIS2_PLACEMENT_3D('',#27626,#20278,#20279);
#17973=AXIS2_PLACEMENT_3D('',#27627,#20280,#20281);
#17974=AXIS2_PLACEMENT_3D('',#27629,#20282,#20283);
#17975=AXIS2_PLACEMENT_3D('',#27631,#20284,#20285);
#17976=AXIS2_PLACEMENT_3D('',#27632,#20286,#20287);
#17977=AXIS2_PLACEMENT_3D('',#27633,#20288,#20289);
#17978=AXIS2_PLACEMENT_3D('',#27635,#20290,#20291);
#17979=AXIS2_PLACEMENT_3D('',#27639,#20293,#20294);
#17980=AXIS2_PLACEMENT_3D('',#27814,#20295,#20296);
#17981=AXIS2_PLACEMENT_3D('',#27817,#20298,#20299);
#17982=AXIS2_PLACEMENT_3D('',#27991,#20300,#20301);
#17983=AXIS2_PLACEMENT_3D('',#27992,#20302,#20303);
#17984=AXIS2_PLACEMENT_3D('',#27994,#20304,#20305);
#17985=AXIS2_PLACEMENT_3D('',#27996,#20306,#20307);
#17986=AXIS2_PLACEMENT_3D('',#27997,#20308,#20309);
#17987=AXIS2_PLACEMENT_3D('',#27998,#20310,#20311);
#17988=AXIS2_PLACEMENT_3D('',#28000,#20312,#20313);
#17989=AXIS2_PLACEMENT_3D('',#28002,#20315,#20316);
#17990=AXIS2_PLACEMENT_3D('',#28004,#20317,#20318);
#17991=AXIS2_PLACEMENT_3D('',#28007,#20320,#20321);
#17992=AXIS2_PLACEMENT_3D('',#28008,#20322,#20323);
#17993=AXIS2_PLACEMENT_3D('',#28085,#20324,#20325);
#17994=AXIS2_PLACEMENT_3D('',#28114,#20326,#20327);
#17995=AXIS2_PLACEMENT_3D('',#28115,#20328,#20329);
#17996=AXIS2_PLACEMENT_3D('',#28116,#20330,#20331);
#17997=AXIS2_PLACEMENT_3D('',#28117,#20332,#20333);
#17998=AXIS2_PLACEMENT_3D('',#28228,#20336,#20337);
#17999=AXIS2_PLACEMENT_3D('',#28339,#20340,#20341);
#18000=AXIS2_PLACEMENT_3D('',#28340,#20342,#20343);
#18001=AXIS2_PLACEMENT_3D('',#28343,#20346,#20347);
#20097=DIRECTION('axis',(0.,0.,1.));
#20098=DIRECTION('refdir',(1.,0.,0.));
#20099=DIRECTION('center_axis',(1.,4.0668225646129E-15,-2.78321068817773E-14));
#20100=DIRECTION('ref_axis',(-2.89386232545955E-14,0.0348994967025012,-0.999390827019096));
#20101=DIRECTION('',(-1.,-4.0668225646129E-15,2.78321068817773E-14));
#20102=DIRECTION('',(1.,0.,-2.18547839493123E-14));
#20103=DIRECTION('center_axis',(1.,4.0668225646129E-15,-2.78321068817773E-14));
#20104=DIRECTION('ref_axis',(-2.89386232545955E-14,0.0348994967025012,-0.999390827019096));
#20105=DIRECTION('',(-1.,-4.0668225646129E-15,2.78321068817773E-14));
#20106=DIRECTION('center_axis',(1.,4.0668225646129E-15,-2.78321068817773E-14));
#20107=DIRECTION('ref_axis',(-2.89386232545955E-14,0.0348994967025012,-0.999390827019096));
#20108=DIRECTION('',(-1.,-4.0668225646129E-15,2.78321068817773E-14));
#20109=DIRECTION('center_axis',(1.,4.0668225646129E-15,-2.78321068817773E-14));
#20110=DIRECTION('ref_axis',(-2.89386232545955E-14,0.0348994967025012,-0.999390827019096));
#20111=DIRECTION('',(-1.,-4.0668225646129E-15,2.78321068817773E-14));
#20112=DIRECTION('center_axis',(1.,4.0668225646129E-15,-2.78321068817773E-14));
#20113=DIRECTION('ref_axis',(-2.89386232545955E-14,0.0348994967025012,-0.999390827019096));
#20114=DIRECTION('',(-1.,-4.0668225646129E-15,2.78321068817773E-14));
#20115=DIRECTION('center_axis',(1.,4.0668225646129E-15,-2.78321068817773E-14));
#20116=DIRECTION('ref_axis',(-2.89386232545955E-14,0.0348994967025012,-0.999390827019096));
#20117=DIRECTION('',(-1.,-4.0668225646129E-15,2.78321068817773E-14));
#20118=DIRECTION('center_axis',(1.,4.0668225646129E-15,-2.78321068817773E-14));
#20119=DIRECTION('ref_axis',(-2.89386232545955E-14,0.0348994967025012,-0.999390827019096));
#20120=DIRECTION('',(-1.,-4.0668225646129E-15,2.78321068817773E-14));
#20121=DIRECTION('center_axis',(1.,4.0668225646129E-15,-2.78321068817773E-14));
#20122=DIRECTION('ref_axis',(-2.89386232545955E-14,0.0348994967025012,-0.999390827019096));
#20123=DIRECTION('',(-1.,-4.0668225646129E-15,2.78321068817773E-14));
#20124=DIRECTION('center_axis',(1.,4.0668225646129E-15,-2.78321068817773E-14));
#20125=DIRECTION('ref_axis',(-2.89386232545955E-14,0.0348994967025012,-0.999390827019096));
#20126=DIRECTION('',(-1.,-4.0668225646129E-15,2.78321068817773E-14));
#20127=DIRECTION('center_axis',(1.,4.0668225646129E-15,-2.78321068817773E-14));
#20128=DIRECTION('ref_axis',(-2.89386232545955E-14,0.0348994967025012,-0.999390827019096));
#20129=DIRECTION('',(-1.,-4.0668225646129E-15,2.78321068817773E-14));
#20130=DIRECTION('center_axis',(1.,4.0668225646129E-15,-2.78321068817773E-14));
#20131=DIRECTION('ref_axis',(-2.89386232545955E-14,0.0348994967025012,-0.999390827019096));
#20132=DIRECTION('',(-1.,-4.0668225646129E-15,2.78321068817773E-14));
#20133=DIRECTION('center_axis',(1.,4.0668225646129E-15,-2.78321068817773E-14));
#20134=DIRECTION('ref_axis',(-2.89386232545955E-14,0.0348994967025012,-0.999390827019096));
#20135=DIRECTION('',(-1.,-4.0668225646129E-15,2.78321068817773E-14));
#20136=DIRECTION('center_axis',(1.,4.0668225646129E-15,-2.78321068817773E-14));
#20137=DIRECTION('ref_axis',(-2.89386232545955E-14,0.0348994967025012,-0.999390827019096));
#20138=DIRECTION('',(-1.,-4.0668225646129E-15,2.78321068817773E-14));
#20139=DIRECTION('center_axis',(1.,4.0668225646129E-15,-2.78321068817773E-14));
#20140=DIRECTION('ref_axis',(-2.89386232545955E-14,0.0348994967025012,-0.999390827019096));
#20141=DIRECTION('',(-1.,-4.0668225646129E-15,2.78321068817773E-14));
#20142=DIRECTION('center_axis',(1.,4.0668225646129E-15,-2.78321068817773E-14));
#20143=DIRECTION('ref_axis',(-2.89386232545955E-14,0.0348994967025012,-0.999390827019096));
#20144=DIRECTION('',(-1.,-4.0668225646129E-15,2.78321068817773E-14));
#20145=DIRECTION('center_axis',(1.,4.0668225646129E-15,-2.78321068817773E-14));
#20146=DIRECTION('ref_axis',(-2.89386232545955E-14,0.0348994967025012,-0.999390827019096));
#20147=DIRECTION('',(-1.,-4.0668225646129E-15,2.78321068817773E-14));
#20148=DIRECTION('center_axis',(1.,4.0668225646129E-15,-2.78321068817773E-14));
#20149=DIRECTION('ref_axis',(-2.89386232545955E-14,0.0348994967025012,-0.999390827019096));
#20150=DIRECTION('',(-1.,-4.0668225646129E-15,2.78321068817773E-14));
#20151=DIRECTION('center_axis',(1.,4.0668225646129E-15,-2.78321068817773E-14));
#20152=DIRECTION('ref_axis',(-2.89386232545955E-14,0.0348994967025012,-0.999390827019096));
#20153=DIRECTION('',(-1.,-4.0668225646129E-15,2.78321068817773E-14));
#20154=DIRECTION('center_axis',(1.,4.0668225646129E-15,-2.78321068817773E-14));
#20155=DIRECTION('ref_axis',(-2.89386232545955E-14,0.0348994967025012,-0.999390827019096));
#20156=DIRECTION('',(-1.,-4.0668225646129E-15,2.78321068817773E-14));
#20157=DIRECTION('center_axis',(1.,4.0668225646129E-15,-2.78321068817773E-14));
#20158=DIRECTION('ref_axis',(-2.89386232545955E-14,0.0348994967025012,-0.999390827019096));
#20159=DIRECTION('',(-1.,-4.0668225646129E-15,2.78321068817773E-14));
#20160=DIRECTION('center_axis',(1.,4.0668225646129E-15,-2.78321068817773E-14));
#20161=DIRECTION('ref_axis',(-2.89386232545955E-14,0.0348994967025012,-0.999390827019096));
#20162=DIRECTION('',(-1.,-4.0668225646129E-15,2.78321068817773E-14));
#20163=DIRECTION('center_axis',(1.,4.0668225646129E-15,-2.78321068817773E-14));
#20164=DIRECTION('ref_axis',(-2.89386232545955E-14,0.0348994967025012,-0.999390827019096));
#20165=DIRECTION('',(-1.,-4.0668225646129E-15,2.78321068817773E-14));
#20166=DIRECTION('center_axis',(1.,4.0668225646129E-15,-2.78321068817773E-14));
#20167=DIRECTION('ref_axis',(-2.89386232545955E-14,0.0348994967025012,-0.999390827019096));
#20168=DIRECTION('',(-1.,-4.0668225646129E-15,2.78321068817773E-14));
#20169=DIRECTION('center_axis',(1.,4.0668225646129E-15,-2.78321068817773E-14));
#20170=DIRECTION('ref_axis',(-2.89386232545955E-14,0.0348994967025012,-0.999390827019096));
#20171=DIRECTION('',(-1.,-4.0668225646129E-15,2.78321068817773E-14));
#20172=DIRECTION('center_axis',(1.,4.0668225646129E-15,-2.78321068817773E-14));
#20173=DIRECTION('ref_axis',(-2.89386232545955E-14,0.0348994967025012,-0.999390827019096));
#20174=DIRECTION('',(-1.,-4.0668225646129E-15,2.78321068817773E-14));
#20175=DIRECTION('center_axis',(-1.,4.23441820549806E-14,-5.91799305310465E-15));
#20176=DIRECTION('ref_axis',(-4.13408903637085E-14,-0.92318579281223,0.384353993019006));
#20177=DIRECTION('center_axis',(-1.,0.,0.));
#20178=DIRECTION('ref_axis',(0.,0.,1.));
#20179=DIRECTION('',(-1.,0.,0.));
#20180=DIRECTION('center_axis',(-1.,0.,0.));
#20181=DIRECTION('ref_axis',(0.,0.,1.));
#20182=DIRECTION('center_axis',(-1.,0.,0.));
#20183=DIRECTION('ref_axis',(0.,0.,1.));
#20184=DIRECTION('',(-1.,0.,0.));
#20185=DIRECTION('',(-1.,0.,0.));
#20186=DIRECTION('center_axis',(-1.,0.,0.));
#20187=DIRECTION('ref_axis',(0.,0.,1.));
#20188=DIRECTION('center_axis',(-1.,0.,0.));
#20189=DIRECTION('ref_axis',(0.,0.,1.));
#20190=DIRECTION('',(-1.,0.,0.));
#20191=DIRECTION('center_axis',(-1.,0.,0.));
#20192=DIRECTION('ref_axis',(0.,0.,1.));
#20193=DIRECTION('',(-1.,0.,0.));
#20194=DIRECTION('center_axis',(-1.,0.,0.));
#20195=DIRECTION('ref_axis',(0.,0.,1.));
#20196=DIRECTION('',(-1.,0.,0.));
#20197=DIRECTION('center_axis',(-1.,0.,0.));
#20198=DIRECTION('ref_axis',(0.,0.,1.));
#20199=DIRECTION('',(-1.,0.,0.));
#20200=DIRECTION('center_axis',(-1.,0.,0.));
#20201=DIRECTION('ref_axis',(0.,0.,1.));
#20202=DIRECTION('',(-1.,0.,0.));
#20203=DIRECTION('center_axis',(-1.,0.,0.));
#20204=DIRECTION('ref_axis',(0.,0.,1.));
#20205=DIRECTION('',(-1.,0.,0.));
#20206=DIRECTION('center_axis',(-1.,0.,0.));
#20207=DIRECTION('ref_axis',(0.,0.,1.));
#20208=DIRECTION('',(-1.,0.,0.));
#20209=DIRECTION('center_axis',(-1.,0.,0.));
#20210=DIRECTION('ref_axis',(0.,0.,1.));
#20211=DIRECTION('',(-1.,0.,0.));
#20212=DIRECTION('center_axis',(-1.,0.,0.));
#20213=DIRECTION('ref_axis',(0.,0.,1.));
#20214=DIRECTION('',(-1.,0.,0.));
#20215=DIRECTION('center_axis',(-1.,0.,0.));
#20216=DIRECTION('ref_axis',(0.,0.,1.));
#20217=DIRECTION('',(-1.,0.,0.));
#20218=DIRECTION('center_axis',(-1.,0.,0.));
#20219=DIRECTION('ref_axis',(0.,0.,1.));
#20220=DIRECTION('',(-1.,0.,0.));
#20221=DIRECTION('center_axis',(-1.,0.,0.));
#20222=DIRECTION('ref_axis',(0.,0.,1.));
#20223=DIRECTION('',(-1.,0.,0.));
#20224=DIRECTION('center_axis',(-1.,0.,0.));
#20225=DIRECTION('ref_axis',(0.,0.,1.));
#20226=DIRECTION('',(-1.,0.,0.));
#20227=DIRECTION('center_axis',(-1.,0.,0.));
#20228=DIRECTION('ref_axis',(0.,0.,1.));
#20229=DIRECTION('',(-1.,0.,0.));
#20230=DIRECTION('center_axis',(-1.,0.,0.));
#20231=DIRECTION('ref_axis',(0.,0.,1.));
#20232=DIRECTION('',(-1.,0.,0.));
#20233=DIRECTION('center_axis',(-1.,0.,0.));
#20234=DIRECTION('ref_axis',(0.,0.,1.));
#20235=DIRECTION('',(-1.,0.,0.));
#20236=DIRECTION('center_axis',(-1.,0.,0.));
#20237=DIRECTION('ref_axis',(0.,0.,1.));
#20238=DIRECTION('',(-1.,0.,0.));
#20239=DIRECTION('center_axis',(-1.,0.,0.));
#20240=DIRECTION('ref_axis',(0.,0.,1.));
#20241=DIRECTION('',(-1.,0.,0.));
#20242=DIRECTION('center_axis',(-1.,0.,0.));
#20243=DIRECTION('ref_axis',(0.,0.,1.));
#20244=DIRECTION('',(-1.,0.,0.));
#20245=DIRECTION('center_axis',(-1.,0.,0.));
#20246=DIRECTION('ref_axis',(0.,0.,1.));
#20247=DIRECTION('',(-1.,0.,0.));
#20248=DIRECTION('center_axis',(-1.,0.,0.));
#20249=DIRECTION('ref_axis',(0.,0.,1.));
#20250=DIRECTION('',(-1.,0.,0.));
#20251=DIRECTION('center_axis',(-1.,0.,0.));
#20252=DIRECTION('ref_axis',(0.,0.,1.));
#20253=DIRECTION('',(-1.,0.,0.));
#20254=DIRECTION('center_axis',(-1.,0.,0.));
#20255=DIRECTION('ref_axis',(0.,0.,1.));
#20256=DIRECTION('',(-1.,0.,0.));
#20257=DIRECTION('center_axis',(1.,0.,0.));
#20258=DIRECTION('ref_axis',(0.,0.,-1.));
#20259=DIRECTION('center_axis',(-1.,0.,0.));
#20260=DIRECTION('ref_axis',(0.,0.,1.));
#20261=DIRECTION('',(-0.707106781186486,-8.65956056235569E-17,-0.707106781186609));
#20262=DIRECTION('center_axis',(-1.,0.,0.));
#20263=DIRECTION('ref_axis',(0.,0.,1.));
#20264=DIRECTION('center_axis',(1.,0.,0.));
#20265=DIRECTION('ref_axis',(0.,0.,-1.));
#20266=DIRECTION('center_axis',(1.,0.,0.));
#20267=DIRECTION('ref_axis',(0.,0.,-1.));
#20268=DIRECTION('',(1.,0.,0.));
#20269=DIRECTION('center_axis',(-1.,0.,0.));
#20270=DIRECTION('ref_axis',(0.,0.,1.));
#20271=DIRECTION('center_axis',(1.,0.,0.));
#20272=DIRECTION('ref_axis',(0.,0.,1.));
#20273=DIRECTION('',(1.,0.,0.));
#20274=DIRECTION('center_axis',(1.,0.,0.));
#20275=DIRECTION('ref_axis',(0.,0.,-1.));
#20276=DIRECTION('center_axis',(1.,0.,0.));
#20277=DIRECTION('ref_axis',(0.,0.,1.));
#20278=DIRECTION('center_axis',(-1.,0.,0.));
#20279=DIRECTION('ref_axis',(0.,0.,1.));
#20280=DIRECTION('center_axis',(1.,0.,0.));
#20281=DIRECTION('ref_axis',(0.,0.,-1.));
#20282=DIRECTION('center_axis',(1.,0.,0.));
#20283=DIRECTION('ref_axis',(0.,0.,-1.));
#20284=DIRECTION('center_axis',(0.,-1.,-1.22464679914735E-16));
#20285=DIRECTION('ref_axis',(0.,-1.22464679914735E-16,1.));
#20286=DIRECTION('center_axis',(1.,0.,0.));
#20287=DIRECTION('ref_axis',(0.,0.,-1.));
#20288=DIRECTION('center_axis',(1.,0.,0.));
#20289=DIRECTION('ref_axis',(0.,0.,-1.));
#20290=DIRECTION('center_axis',(1.,0.,0.));
#20291=DIRECTION('ref_axis',(0.,0.,-1.));
#20292=DIRECTION('',(-1.,0.,0.));
#20293=DIRECTION('center_axis',(1.,0.,0.));
#20294=DIRECTION('ref_axis',(0.,-0.308832433911277,0.951116463827873));
#20295=DIRECTION('center_axis',(1.,0.,0.));
#20296=DIRECTION('ref_axis',(0.,-0.308832433911277,0.951116463827873));
#20297=DIRECTION('',(-1.,0.,0.));
#20298=DIRECTION('center_axis',(1.,0.,0.));
#20299=DIRECTION('ref_axis',(0.,-0.308832433911277,0.951116463827873));
#20300=DIRECTION('center_axis',(1.,0.,0.));
#20301=DIRECTION('ref_axis',(0.,-0.308832433911277,0.951116463827873));
#20302=DIRECTION('center_axis',(1.,0.,0.));
#20303=DIRECTION('ref_axis',(0.,0.,-1.));
#20304=DIRECTION('center_axis',(1.,0.,0.));
#20305=DIRECTION('ref_axis',(0.,0.,-1.));
#20306=DIRECTION('center_axis',(0.,-1.,-1.22464679914735E-16));
#20307=DIRECTION('ref_axis',(0.,-1.22464679914735E-16,1.));
#20308=DIRECTION('center_axis',(1.,0.,0.));
#20309=DIRECTION('ref_axis',(0.,0.,-1.));
#20310=DIRECTION('center_axis',(1.,0.,0.));
#20311=DIRECTION('ref_axis',(0.,0.,-1.));
#20312=DIRECTION('center_axis',(1.,0.,0.));
#20313=DIRECTION('ref_axis',(0.,0.,-1.));
#20314=DIRECTION('',(-1.,0.,0.));
#20315=DIRECTION('center_axis',(1.,0.,0.));
#20316=DIRECTION('ref_axis',(0.,0.,-1.));
#20317=DIRECTION('center_axis',(1.,0.,0.));
#20318=DIRECTION('ref_axis',(0.,0.,-1.));
#20319=DIRECTION('',(1.,0.,0.));
#20320=DIRECTION('center_axis',(1.,0.,0.));
#20321=DIRECTION('ref_axis',(0.,0.,-1.));
#20322=DIRECTION('center_axis',(-1.,0.,0.));
#20323=DIRECTION('ref_axis',(0.,0.,1.));
#20324=DIRECTION('center_axis',(1.,0.,0.));
#20325=DIRECTION('ref_axis',(0.,0.,-1.));
#20326=DIRECTION('center_axis',(1.,0.,0.));
#20327=DIRECTION('ref_axis',(0.,0.,-1.));
#20328=DIRECTION('center_axis',(1.,0.,0.));
#20329=DIRECTION('ref_axis',(0.,0.,-1.));
#20330=DIRECTION('center_axis',(-1.,0.,0.));
#20331=DIRECTION('ref_axis',(0.,0.,1.));
#20332=DIRECTION('center_axis',(-1.,0.,0.));
#20333=DIRECTION('ref_axis',(0.,0.,1.));
#20334=DIRECTION('',(-3.94745964311166E-15,0.774569892332855,0.632488325498163));
#20335=DIRECTION('',(-9.86864910777916E-16,0.774569892332855,0.632488325498162));
#20336=DIRECTION('center_axis',(-1.,0.,0.));
#20337=DIRECTION('ref_axis',(0.,0.,1.));
#20338=DIRECTION('',(0.,-0.308832433911277,0.951116463827873));
#20339=DIRECTION('',(0.,-0.308832433911277,0.951116463827873));
#20340=DIRECTION('center_axis',(-1.,0.,0.));
#20341=DIRECTION('ref_axis',(0.,0.,1.));
#20342=DIRECTION('center_axis',(-7.62720960372908E-16,-0.999390827019096,
-0.0348994967025015));
#20343=DIRECTION('ref_axis',(3.27874698101124E-34,0.0348994967025015,-0.999390827019096));
#20344=DIRECTION('',(0.499999999999987,0.0302238507236574,-0.865497844507684));
#20345=DIRECTION('',(0.499999999999985,-0.0302238507236573,0.865497844507685));
#20346=DIRECTION('center_axis',(1.,4.0668225646129E-15,-2.78321068817773E-14));
#20347=DIRECTION('ref_axis',(-2.89386232545955E-14,0.0348994967025012,-0.999390827019096));
#24971=CARTESIAN_POINT('',(0.,0.,0.));
#24972=CARTESIAN_POINT('Origin',(-43.8559375004335,-3.93782229046735E-15,
8.32667268468867E-14));
#24973=CARTESIAN_POINT('',(-43.6773437504336,-0.149957969249584,4.29423438922274));
#24974=CARTESIAN_POINT('',(-43.7170312504336,-0.149957969249584,4.29423438922274));
#24975=CARTESIAN_POINT('',(-43.8559375004333,-0.149957969249592,4.2942343892229));
#24976=CARTESIAN_POINT('',(-43.8757812504336,0.149957969249583,-4.29423438922274));
#24977=CARTESIAN_POINT('Ctrl Pts',(-43.8757812504336,0.149957969249583,
-4.29423438922274));
#24978=CARTESIAN_POINT('Ctrl Pts',(-43.8493229171003,2.62923534983068,-4.20765611530936));
#24979=CARTESIAN_POINT('Ctrl Pts',(-43.8228645837669,3.79389505549643,-2.0172497837413));
#24980=CARTESIAN_POINT('Ctrl Pts',(-43.7964062504336,4.95855476116219,0.173156547826753));
#24981=CARTESIAN_POINT('Ctrl Pts',(-43.7699479171003,3.64393708624685,2.27698460548143));
#24982=CARTESIAN_POINT('Ctrl Pts',(-43.7434895837669,2.32931941133151,4.38081266313611));
#24983=CARTESIAN_POINT('Ctrl Pts',(-43.7170312504336,-0.149957969249583,
4.29423438922274));
#24984=CARTESIAN_POINT('',(-43.8360937504336,0.149957969249583,-4.29423438922274));
#24985=CARTESIAN_POINT('',(-43.8559375004336,0.149957969249583,-4.29423438922274));
#24986=CARTESIAN_POINT('Ctrl Pts',(-43.8360937504336,0.149957969249583,
-4.29423438922274));
#24987=CARTESIAN_POINT('Ctrl Pts',(-43.8096354171003,2.62923534983068,-4.20765611530936));
#24988=CARTESIAN_POINT('Ctrl Pts',(-43.7831770837669,3.79389505549644,-2.0172497837413));
#24989=CARTESIAN_POINT('Ctrl Pts',(-43.7567187504336,4.95855476116219,0.173156547826753));
#24990=CARTESIAN_POINT('Ctrl Pts',(-43.7302604171003,3.64393708624685,2.27698460548143));
#24991=CARTESIAN_POINT('Ctrl Pts',(-43.7038020837669,2.32931941133151,4.38081266313611));
#24992=CARTESIAN_POINT('Ctrl Pts',(-43.6773437504336,-0.149957969249583,
4.29423438922274));
#24993=CARTESIAN_POINT('Origin',(-43.8559375004335,-3.93782229046735E-15,
8.32667268468867E-14));
#24994=CARTESIAN_POINT('',(-43.3598437504336,-0.149957969249584,4.29423438922274));
#24995=CARTESIAN_POINT('',(-43.3995312504336,-0.149957969249584,4.29423438922274));
#24996=CARTESIAN_POINT('',(-43.8559375004333,-0.149957969249592,4.2942343892229));
#24997=CARTESIAN_POINT('Ctrl Pts',(-43.7170312504336,-0.149957969249583,
4.29423438922274));
#24998=CARTESIAN_POINT('Ctrl Pts',(-43.6905729171003,-2.62923534983068,
4.20765611530936));
#24999=CARTESIAN_POINT('Ctrl Pts',(-43.6641145837669,-3.79389505549643,
2.01724978374131));
#25000=CARTESIAN_POINT('Ctrl Pts',(-43.6376562504336,-4.95855476116219,
-0.173156547826752));
#25001=CARTESIAN_POINT('Ctrl Pts',(-43.6111979171003,-3.64393708624685,
-2.27698460548143));
#25002=CARTESIAN_POINT('Ctrl Pts',(-43.5847395837669,-2.32931941133151,
-4.38081266313611));
#25003=CARTESIAN_POINT('Ctrl Pts',(-43.5582812504336,0.149957969249583,
-4.29423438922274));
#25004=CARTESIAN_POINT('Ctrl Pts',(-43.5318229171003,2.62923534983068,-4.20765611530936));
#25005=CARTESIAN_POINT('Ctrl Pts',(-43.5053645837669,3.79389505549643,-2.0172497837413));
#25006=CARTESIAN_POINT('Ctrl Pts',(-43.4789062504336,4.95855476116219,0.173156547826753));
#25007=CARTESIAN_POINT('Ctrl Pts',(-43.4524479171003,3.64393708624685,2.27698460548143));
#25008=CARTESIAN_POINT('Ctrl Pts',(-43.4259895837669,2.32931941133151,4.38081266313611));
#25009=CARTESIAN_POINT('Ctrl Pts',(-43.3995312504336,-0.149957969249583,
4.29423438922274));
#25010=CARTESIAN_POINT('Ctrl Pts',(-43.6773437504336,-0.149957969249583,
4.29423438922274));
#25011=CARTESIAN_POINT('Ctrl Pts',(-43.6508854171003,-2.62923534983068,
4.20765611530936));
#25012=CARTESIAN_POINT('Ctrl Pts',(-43.6244270837669,-3.79389505549643,
2.01724978374131));
#25013=CARTESIAN_POINT('Ctrl Pts',(-43.5979687504336,-4.95855476116219,
-0.173156547826752));
#25014=CARTESIAN_POINT('Ctrl Pts',(-43.5715104171003,-3.64393708624685,
-2.27698460548143));
#25015=CARTESIAN_POINT('Ctrl Pts',(-43.5450520837669,-2.32931941133151,
-4.38081266313611));
#25016=CARTESIAN_POINT('Ctrl Pts',(-43.5185937504336,0.149957969249583,
-4.29423438922274));
#25017=CARTESIAN_POINT('Ctrl Pts',(-43.4921354171003,2.62923534983068,-4.20765611530936));
#25018=CARTESIAN_POINT('Ctrl Pts',(-43.4656770837669,3.79389505549644,-2.0172497837413));
#25019=CARTESIAN_POINT('Ctrl Pts',(-43.4392187504336,4.95855476116219,0.173156547826753));
#25020=CARTESIAN_POINT('Ctrl Pts',(-43.4127604171003,3.64393708624685,2.27698460548143));
#25021=CARTESIAN_POINT('Ctrl Pts',(-43.3863020837669,2.32931941133151,4.38081266313611));
#25022=CARTESIAN_POINT('Ctrl Pts',(-43.3598437504336,-0.149957969249583,
4.29423438922274));
#25023=CARTESIAN_POINT('Origin',(-43.8559375004335,-3.93782229046735E-15,
8.32667268468867E-14));
#25024=CARTESIAN_POINT('',(-43.0423437504336,-0.149957969249583,4.29423438922274));
#25025=CARTESIAN_POINT('',(-43.0820312504336,-0.149957969249583,4.29423438922274));
#25026=CARTESIAN_POINT('',(-43.8559375004333,-0.149957969249592,4.2942343892229));
#25027=CARTESIAN_POINT('Ctrl Pts',(-43.3995312504336,-0.149957969249583,
4.29423438922274));
#25028=CARTESIAN_POINT('Ctrl Pts',(-43.3730729171003,-2.62923534983068,
4.20765611530936));
#25029=CARTESIAN_POINT('Ctrl Pts',(-43.3466145837669,-3.79389505549643,
2.01724978374131));
#25030=CARTESIAN_POINT('Ctrl Pts',(-43.3201562504336,-4.95855476116219,
-0.173156547826752));
#25031=CARTESIAN_POINT('Ctrl Pts',(-43.2936979171003,-3.64393708624685,
-2.27698460548143));
#25032=CARTESIAN_POINT('Ctrl Pts',(-43.2672395837669,-2.32931941133151,
-4.38081266313611));
#25033=CARTESIAN_POINT('Ctrl Pts',(-43.2407812504336,0.149957969249583,
-4.29423438922274));
#25034=CARTESIAN_POINT('Ctrl Pts',(-43.2143229171003,2.62923534983068,-4.20765611530936));
#25035=CARTESIAN_POINT('Ctrl Pts',(-43.1878645837669,3.79389505549643,-2.0172497837413));
#25036=CARTESIAN_POINT('Ctrl Pts',(-43.1614062504336,4.95855476116219,0.173156547826753));
#25037=CARTESIAN_POINT('Ctrl Pts',(-43.1349479171003,3.64393708624685,2.27698460548143));
#25038=CARTESIAN_POINT('Ctrl Pts',(-43.1084895837669,2.32931941133151,4.38081266313611));
#25039=CARTESIAN_POINT('Ctrl Pts',(-43.0820312504336,-0.149957969249583,
4.29423438922274));
#25040=CARTESIAN_POINT('Ctrl Pts',(-43.3598437504336,-0.149957969249583,
4.29423438922274));
#25041=CARTESIAN_POINT('Ctrl Pts',(-43.3333854171003,-2.62923534983068,
4.20765611530936));
#25042=CARTESIAN_POINT('Ctrl Pts',(-43.3069270837669,-3.79389505549643,
2.01724978374131));
#25043=CARTESIAN_POINT('Ctrl Pts',(-43.2804687504336,-4.95855476116219,
-0.173156547826752));
#25044=CARTESIAN_POINT('Ctrl Pts',(-43.2540104171003,-3.64393708624685,
-2.27698460548143));
#25045=CARTESIAN_POINT('Ctrl Pts',(-43.2275520837669,-2.32931941133151,
-4.38081266313611));
#25046=CARTESIAN_POINT('Ctrl Pts',(-43.2010937504336,0.149957969249583,
-4.29423438922274));
#25047=CARTESIAN_POINT('Ctrl Pts',(-43.1746354171003,2.62923534983068,-4.20765611530936));
#25048=CARTESIAN_POINT('Ctrl Pts',(-43.1481770837669,3.79389505549644,-2.0172497837413));
#25049=CARTESIAN_POINT('Ctrl Pts',(-43.1217187504336,4.95855476116219,0.173156547826753));
#25050=CARTESIAN_POINT('Ctrl Pts',(-43.0952604171003,3.64393708624685,2.27698460548143));
#25051=CARTESIAN_POINT('Ctrl Pts',(-43.0688020837669,2.32931941133151,4.38081266313611));
#25052=CARTESIAN_POINT('Ctrl Pts',(-43.0423437504336,-0.149957969249583,
4.29423438922274));
#25053=CARTESIAN_POINT('Origin',(-43.8559375004335,-3.93782229046735E-15,
8.32667268468867E-14));
#25054=CARTESIAN_POINT('',(-42.7248437504336,-0.149957969249583,4.29423438922274));
#25055=CARTESIAN_POINT('',(-42.7645312504336,-0.149957969249583,4.29423438922274));
#25056=CARTESIAN_POINT('',(-43.8559375004333,-0.149957969249592,4.2942343892229));
#25057=CARTESIAN_POINT('Ctrl Pts',(-43.0820312504336,-0.149957969249583,
4.29423438922274));
#25058=CARTESIAN_POINT('Ctrl Pts',(-43.0555729171003,-2.62923534983068,
4.20765611530936));
#25059=CARTESIAN_POINT('Ctrl Pts',(-43.0291145837669,-3.79389505549643,
2.01724978374131));
#25060=CARTESIAN_POINT('Ctrl Pts',(-43.0026562504336,-4.95855476116219,
-0.173156547826752));
#25061=CARTESIAN_POINT('Ctrl Pts',(-42.9761979171003,-3.64393708624685,
-2.27698460548143));
#25062=CARTESIAN_POINT('Ctrl Pts',(-42.9497395837669,-2.32931941133151,
-4.38081266313611));
#25063=CARTESIAN_POINT('Ctrl Pts',(-42.9232812504336,0.149957969249583,
-4.29423438922274));
#25064=CARTESIAN_POINT('Ctrl Pts',(-42.8968229171003,2.62923534983068,-4.20765611530936));
#25065=CARTESIAN_POINT('Ctrl Pts',(-42.8703645837669,3.79389505549643,-2.0172497837413));
#25066=CARTESIAN_POINT('Ctrl Pts',(-42.8439062504336,4.95855476116219,0.173156547826753));
#25067=CARTESIAN_POINT('Ctrl Pts',(-42.8174479171003,3.64393708624685,2.27698460548143));
#25068=CARTESIAN_POINT('Ctrl Pts',(-42.7909895837669,2.32931941133151,4.38081266313611));
#25069=CARTESIAN_POINT('Ctrl Pts',(-42.7645312504336,-0.149957969249583,
4.29423438922274));
#25070=CARTESIAN_POINT('Ctrl Pts',(-43.0423437504336,-0.149957969249583,
4.29423438922274));
#25071=CARTESIAN_POINT('Ctrl Pts',(-43.0158854171003,-2.62923534983068,
4.20765611530936));
#25072=CARTESIAN_POINT('Ctrl Pts',(-42.9894270837669,-3.79389505549643,
2.01724978374131));
#25073=CARTESIAN_POINT('Ctrl Pts',(-42.9629687504336,-4.95855476116219,
-0.173156547826752));
#25074=CARTESIAN_POINT('Ctrl Pts',(-42.9365104171003,-3.64393708624685,
-2.27698460548143));
#25075=CARTESIAN_POINT('Ctrl Pts',(-42.9100520837669,-2.32931941133151,
-4.38081266313611));
#25076=CARTESIAN_POINT('Ctrl Pts',(-42.8835937504336,0.149957969249583,
-4.29423438922274));
#25077=CARTESIAN_POINT('Ctrl Pts',(-42.8571354171003,2.62923534983068,-4.20765611530936));
#25078=CARTESIAN_POINT('Ctrl Pts',(-42.8306770837669,3.79389505549644,-2.0172497837413));
#25079=CARTESIAN_POINT('Ctrl Pts',(-42.8042187504336,4.95855476116219,0.173156547826753));
#25080=CARTESIAN_POINT('Ctrl Pts',(-42.7777604171003,3.64393708624685,2.27698460548143));
#25081=CARTESIAN_POINT('Ctrl Pts',(-42.7513020837669,2.32931941133151,4.38081266313611));
#25082=CARTESIAN_POINT('Ctrl Pts',(-42.7248437504336,-0.149957969249583,
4.29423438922274));
#25083=CARTESIAN_POINT('Origin',(-43.8559375004335,-3.93782229046735E-15,
8.32667268468867E-14));
#25084=CARTESIAN_POINT('',(-42.4073437504336,-0.149957969249582,4.29423438922274));
#25085=CARTESIAN_POINT('',(-42.4470312504336,-0.149957969249582,4.29423438922274));
#25086=CARTESIAN_POINT('',(-43.8559375004333,-0.149957969249592,4.2942343892229));
#25087=CARTESIAN_POINT('Ctrl Pts',(-42.7645312504336,-0.149957969249583,
4.29423438922274));
#25088=CARTESIAN_POINT('Ctrl Pts',(-42.7380729171003,-2.62923534983068,
4.20765611530936));
#25089=CARTESIAN_POINT('Ctrl Pts',(-42.7116145837669,-3.79389505549643,
2.01724978374131));
#25090=CARTESIAN_POINT('Ctrl Pts',(-42.6851562504336,-4.95855476116219,
-0.173156547826752));
#25091=CARTESIAN_POINT('Ctrl Pts',(-42.6586979171003,-3.64393708624685,
-2.27698460548143));
#25092=CARTESIAN_POINT('Ctrl Pts',(-42.6322395837669,-2.32931941133151,
-4.38081266313611));
#25093=CARTESIAN_POINT('Ctrl Pts',(-42.6057812504336,0.149957969249583,
-4.29423438922274));
#25094=CARTESIAN_POINT('Ctrl Pts',(-42.5793229171003,2.62923534983068,-4.20765611530936));
#25095=CARTESIAN_POINT('Ctrl Pts',(-42.5528645837669,3.79389505549643,-2.0172497837413));
#25096=CARTESIAN_POINT('Ctrl Pts',(-42.5264062504336,4.95855476116219,0.173156547826753));
#25097=CARTESIAN_POINT('Ctrl Pts',(-42.4999479171003,3.64393708624685,2.27698460548143));
#25098=CARTESIAN_POINT('Ctrl Pts',(-42.4734895837669,2.32931941133151,4.38081266313611));
#25099=CARTESIAN_POINT('Ctrl Pts',(-42.4470312504336,-0.149957969249583,
4.29423438922274));
#25100=CARTESIAN_POINT('Ctrl Pts',(-42.7248437504336,-0.149957969249583,
4.29423438922274));
#25101=CARTESIAN_POINT('Ctrl Pts',(-42.6983854171003,-2.62923534983068,
4.20765611530936));
#25102=CARTESIAN_POINT('Ctrl Pts',(-42.6719270837669,-3.79389505549643,
2.01724978374131));
#25103=CARTESIAN_POINT('Ctrl Pts',(-42.6454687504336,-4.95855476116219,
-0.173156547826752));
#25104=CARTESIAN_POINT('Ctrl Pts',(-42.6190104171003,-3.64393708624685,
-2.27698460548143));
#25105=CARTESIAN_POINT('Ctrl Pts',(-42.5925520837669,-2.32931941133151,
-4.38081266313611));
#25106=CARTESIAN_POINT('Ctrl Pts',(-42.5660937504336,0.149957969249583,
-4.29423438922274));
#25107=CARTESIAN_POINT('Ctrl Pts',(-42.5396354171003,2.62923534983068,-4.20765611530936));
#25108=CARTESIAN_POINT('Ctrl Pts',(-42.5131770837669,3.79389505549644,-2.0172497837413));
#25109=CARTESIAN_POINT('Ctrl Pts',(-42.4867187504336,4.95855476116219,0.173156547826753));
#25110=CARTESIAN_POINT('Ctrl Pts',(-42.4602604171003,3.64393708624685,2.27698460548143));
#25111=CARTESIAN_POINT('Ctrl Pts',(-42.4338020837669,2.32931941133151,4.38081266313611));
#25112=CARTESIAN_POINT('Ctrl Pts',(-42.4073437504336,-0.149957969249583,
4.29423438922274));
#25113=CARTESIAN_POINT('Origin',(-43.8559375004335,-3.93782229046735E-15,
8.32667268468867E-14));
#25114=CARTESIAN_POINT('',(-42.0898437504336,-0.149957969249582,4.29423438922274));
#25115=CARTESIAN_POINT('',(-42.1295312504336,-0.149957969249582,4.29423438922274));
#25116=CARTESIAN_POINT('',(-43.8559375004333,-0.149957969249592,4.2942343892229));
#25117=CARTESIAN_POINT('Ctrl Pts',(-42.4470312504336,-0.149957969249583,
4.29423438922274));
#25118=CARTESIAN_POINT('Ctrl Pts',(-42.4205729171003,-2.62923534983068,
4.20765611530936));
#25119=CARTESIAN_POINT('Ctrl Pts',(-42.3941145837669,-3.79389505549643,
2.01724978374131));
#25120=CARTESIAN_POINT('Ctrl Pts',(-42.3676562504336,-4.95855476116219,
-0.173156547826752));
#25121=CARTESIAN_POINT('Ctrl Pts',(-42.3411979171003,-3.64393708624685,
-2.27698460548143));
#25122=CARTESIAN_POINT('Ctrl Pts',(-42.3147395837669,-2.32931941133151,
-4.38081266313611));
#25123=CARTESIAN_POINT('Ctrl Pts',(-42.2882812504336,0.149957969249583,
-4.29423438922274));
#25124=CARTESIAN_POINT('Ctrl Pts',(-42.2618229171003,2.62923534983068,-4.20765611530936));
#25125=CARTESIAN_POINT('Ctrl Pts',(-42.2353645837669,3.79389505549643,-2.0172497837413));
#25126=CARTESIAN_POINT('Ctrl Pts',(-42.2089062504336,4.95855476116219,0.173156547826753));
#25127=CARTESIAN_POINT('Ctrl Pts',(-42.1824479171003,3.64393708624685,2.27698460548143));
#25128=CARTESIAN_POINT('Ctrl Pts',(-42.1559895837669,2.32931941133151,4.38081266313611));
#25129=CARTESIAN_POINT('Ctrl Pts',(-42.1295312504336,-0.149957969249583,
4.29423438922274));
#25130=CARTESIAN_POINT('Ctrl Pts',(-42.4073437504336,-0.149957969249583,
4.29423438922274));
#25131=CARTESIAN_POINT('Ctrl Pts',(-42.3808854171003,-2.62923534983068,
4.20765611530936));
#25132=CARTESIAN_POINT('Ctrl Pts',(-42.3544270837669,-3.79389505549643,
2.01724978374131));
#25133=CARTESIAN_POINT('Ctrl Pts',(-42.3279687504336,-4.95855476116219,
-0.173156547826752));
#25134=CARTESIAN_POINT('Ctrl Pts',(-42.3015104171003,-3.64393708624685,
-2.27698460548143));
#25135=CARTESIAN_POINT('Ctrl Pts',(-42.2750520837669,-2.32931941133151,
-4.38081266313611));
#25136=CARTESIAN_POINT('Ctrl Pts',(-42.2485937504336,0.149957969249583,
-4.29423438922274));
#25137=CARTESIAN_POINT('Ctrl Pts',(-42.2221354171003,2.62923534983068,-4.20765611530936));
#25138=CARTESIAN_POINT('Ctrl Pts',(-42.1956770837669,3.79389505549644,-2.0172497837413));
#25139=CARTESIAN_POINT('Ctrl Pts',(-42.1692187504336,4.95855476116219,0.173156547826753));
#25140=CARTESIAN_POINT('Ctrl Pts',(-42.1427604171003,3.64393708624685,2.27698460548143));
#25141=CARTESIAN_POINT('Ctrl Pts',(-42.1163020837669,2.32931941133151,4.38081266313611));
#25142=CARTESIAN_POINT('Ctrl Pts',(-42.0898437504336,-0.149957969249583,
4.29423438922274));
#25143=CARTESIAN_POINT('Origin',(-43.8559375004335,-3.93782229046735E-15,
8.32667268468867E-14));
#25144=CARTESIAN_POINT('',(-41.7723437504336,-0.149957969249581,4.29423438922274));
#25145=CARTESIAN_POINT('',(-41.8120312504336,-0.149957969249581,4.29423438922274));
#25146=CARTESIAN_POINT('',(-43.8559375004333,-0.149957969249592,4.2942343892229));
#25147=CARTESIAN_POINT('Ctrl Pts',(-42.1295312504336,-0.149957969249583,
4.29423438922274));
#25148=CARTESIAN_POINT('Ctrl Pts',(-42.1030729171003,-2.62923534983068,
4.20765611530936));
#25149=CARTESIAN_POINT('Ctrl Pts',(-42.0766145837669,-3.79389505549643,
2.01724978374131));
#25150=CARTESIAN_POINT('Ctrl Pts',(-42.0501562504336,-4.95855476116219,
-0.173156547826752));
#25151=CARTESIAN_POINT('Ctrl Pts',(-42.0236979171003,-3.64393708624685,
-2.27698460548143));
#25152=CARTESIAN_POINT('Ctrl Pts',(-41.9972395837669,-2.32931941133151,
-4.38081266313611));
#25153=CARTESIAN_POINT('Ctrl Pts',(-41.9707812504336,0.149957969249583,
-4.29423438922274));
#25154=CARTESIAN_POINT('Ctrl Pts',(-41.9443229171003,2.62923534983068,-4.20765611530936));
#25155=CARTESIAN_POINT('Ctrl Pts',(-41.9178645837669,3.79389505549643,-2.0172497837413));
#25156=CARTESIAN_POINT('Ctrl Pts',(-41.8914062504336,4.95855476116219,0.173156547826753));
#25157=CARTESIAN_POINT('Ctrl Pts',(-41.8649479171003,3.64393708624685,2.27698460548143));
#25158=CARTESIAN_POINT('Ctrl Pts',(-41.8384895837669,2.32931941133151,4.38081266313611));
#25159=CARTESIAN_POINT('Ctrl Pts',(-41.8120312504336,-0.149957969249583,
4.29423438922274));
#25160=CARTESIAN_POINT('Ctrl Pts',(-42.0898437504336,-0.149957969249583,
4.29423438922274));
#25161=CARTESIAN_POINT('Ctrl Pts',(-42.0633854171003,-2.62923534983068,
4.20765611530936));
#25162=CARTESIAN_POINT('Ctrl Pts',(-42.0369270837669,-3.79389505549643,
2.01724978374131));
#25163=CARTESIAN_POINT('Ctrl Pts',(-42.0104687504336,-4.95855476116219,
-0.173156547826752));
#25164=CARTESIAN_POINT('Ctrl Pts',(-41.9840104171003,-3.64393708624685,
-2.27698460548143));
#25165=CARTESIAN_POINT('Ctrl Pts',(-41.9575520837669,-2.32931941133151,
-4.38081266313611));
#25166=CARTESIAN_POINT('Ctrl Pts',(-41.9310937504336,0.149957969249583,
-4.29423438922274));
#25167=CARTESIAN_POINT('Ctrl Pts',(-41.9046354171003,2.62923534983068,-4.20765611530936));
#25168=CARTESIAN_POINT('Ctrl Pts',(-41.8781770837669,3.79389505549644,-2.0172497837413));
#25169=CARTESIAN_POINT('Ctrl Pts',(-41.8517187504336,4.95855476116219,0.173156547826753));
#25170=CARTESIAN_POINT('Ctrl Pts',(-41.8252604171003,3.64393708624685,2.27698460548143));
#25171=CARTESIAN_POINT('Ctrl Pts',(-41.7988020837669,2.32931941133151,4.38081266313611));
#25172=CARTESIAN_POINT('Ctrl Pts',(-41.7723437504336,-0.149957969249583,
4.29423438922274));
#25173=CARTESIAN_POINT('Origin',(-43.8559375004335,-3.93782229046735E-15,
8.32667268468867E-14));
#25174=CARTESIAN_POINT('',(-41.4548437504336,-0.149957969249581,4.29423438922274));
#25175=CARTESIAN_POINT('',(-41.4945312504336,-0.149957969249581,4.29423438922274));
#25176=CARTESIAN_POINT('',(-43.8559375004333,-0.149957969249592,4.2942343892229));
#25177=CARTESIAN_POINT('Ctrl Pts',(-41.8120312504336,-0.149957969249583,
4.29423438922274));
#25178=CARTESIAN_POINT('Ctrl Pts',(-41.7855729171003,-2.62923534983068,
4.20765611530936));
#25179=CARTESIAN_POINT('Ctrl Pts',(-41.7591145837669,-3.79389505549643,
2.01724978374131));
#25180=CARTESIAN_POINT('Ctrl Pts',(-41.7326562504336,-4.95855476116219,
-0.173156547826752));
#25181=CARTESIAN_POINT('Ctrl Pts',(-41.7061979171003,-3.64393708624685,
-2.27698460548143));
#25182=CARTESIAN_POINT('Ctrl Pts',(-41.6797395837669,-2.32931941133151,
-4.38081266313611));
#25183=CARTESIAN_POINT('Ctrl Pts',(-41.6532812504336,0.149957969249583,
-4.29423438922274));
#25184=CARTESIAN_POINT('Ctrl Pts',(-41.6268229171003,2.62923534983068,-4.20765611530936));
#25185=CARTESIAN_POINT('Ctrl Pts',(-41.6003645837669,3.79389505549643,-2.0172497837413));
#25186=CARTESIAN_POINT('Ctrl Pts',(-41.5739062504336,4.95855476116219,0.173156547826753));
#25187=CARTESIAN_POINT('Ctrl Pts',(-41.5474479171003,3.64393708624685,2.27698460548143));
#25188=CARTESIAN_POINT('Ctrl Pts',(-41.5209895837669,2.32931941133151,4.38081266313611));
#25189=CARTESIAN_POINT('Ctrl Pts',(-41.4945312504336,-0.149957969249583,
4.29423438922274));
#25190=CARTESIAN_POINT('Ctrl Pts',(-41.7723437504336,-0.149957969249583,
4.29423438922274));
#25191=CARTESIAN_POINT('Ctrl Pts',(-41.7458854171003,-2.62923534983068,
4.20765611530936));
#25192=CARTESIAN_POINT('Ctrl Pts',(-41.7194270837669,-3.79389505549643,
2.01724978374131));
#25193=CARTESIAN_POINT('Ctrl Pts',(-41.6929687504336,-4.95855476116219,
-0.173156547826752));
#25194=CARTESIAN_POINT('Ctrl Pts',(-41.6665104171003,-3.64393708624685,
-2.27698460548143));
#25195=CARTESIAN_POINT('Ctrl Pts',(-41.6400520837669,-2.32931941133151,
-4.38081266313611));
#25196=CARTESIAN_POINT('Ctrl Pts',(-41.6135937504336,0.149957969249583,
-4.29423438922274));
#25197=CARTESIAN_POINT('Ctrl Pts',(-41.5871354171003,2.62923534983068,-4.20765611530936));
#25198=CARTESIAN_POINT('Ctrl Pts',(-41.5606770837669,3.79389505549644,-2.0172497837413));
#25199=CARTESIAN_POINT('Ctrl Pts',(-41.5342187504336,4.95855476116219,0.173156547826753));
#25200=CARTESIAN_POINT('Ctrl Pts',(-41.5077604171003,3.64393708624685,2.27698460548143));
#25201=CARTESIAN_POINT('Ctrl Pts',(-41.4813020837669,2.32931941133151,4.38081266313611));
#25202=CARTESIAN_POINT('Ctrl Pts',(-41.4548437504336,-0.149957969249583,
4.29423438922274));
#25203=CARTESIAN_POINT('Origin',(-43.8559375004335,-3.93782229046735E-15,
8.32667268468867E-14));
#25204=CARTESIAN_POINT('',(-41.1373437504336,-0.14995796924958,4.29423438922274));
#25205=CARTESIAN_POINT('',(-41.1770312504336,-0.14995796924958,4.29423438922274));
#25206=CARTESIAN_POINT('',(-43.8559375004333,-0.149957969249592,4.2942343892229));
#25207=CARTESIAN_POINT('Ctrl Pts',(-41.4945312504336,-0.149957969249583,
4.29423438922274));
#25208=CARTESIAN_POINT('Ctrl Pts',(-41.4680729171003,-2.62923534983068,
4.20765611530936));
#25209=CARTESIAN_POINT('Ctrl Pts',(-41.4416145837669,-3.79389505549643,
2.01724978374131));
#25210=CARTESIAN_POINT('Ctrl Pts',(-41.4151562504336,-4.95855476116219,
-0.173156547826752));
#25211=CARTESIAN_POINT('Ctrl Pts',(-41.3886979171003,-3.64393708624685,
-2.27698460548143));
#25212=CARTESIAN_POINT('Ctrl Pts',(-41.3622395837669,-2.32931941133151,
-4.38081266313611));
#25213=CARTESIAN_POINT('Ctrl Pts',(-41.3357812504336,0.149957969249583,
-4.29423438922274));
#25214=CARTESIAN_POINT('Ctrl Pts',(-41.3093229171003,2.62923534983068,-4.20765611530936));
#25215=CARTESIAN_POINT('Ctrl Pts',(-41.2828645837669,3.79389505549643,-2.0172497837413));
#25216=CARTESIAN_POINT('Ctrl Pts',(-41.2564062504336,4.95855476116219,0.173156547826753));
#25217=CARTESIAN_POINT('Ctrl Pts',(-41.2299479171003,3.64393708624685,2.27698460548143));
#25218=CARTESIAN_POINT('Ctrl Pts',(-41.2034895837669,2.32931941133151,4.38081266313611));
#25219=CARTESIAN_POINT('Ctrl Pts',(-41.1770312504336,-0.149957969249583,
4.29423438922274));
#25220=CARTESIAN_POINT('Ctrl Pts',(-41.4548437504336,-0.149957969249583,
4.29423438922274));
#25221=CARTESIAN_POINT('Ctrl Pts',(-41.4283854171003,-2.62923534983068,
4.20765611530936));
#25222=CARTESIAN_POINT('Ctrl Pts',(-41.4019270837669,-3.79389505549643,
2.01724978374131));
#25223=CARTESIAN_POINT('Ctrl Pts',(-41.3754687504336,-4.95855476116219,
-0.173156547826752));
#25224=CARTESIAN_POINT('Ctrl Pts',(-41.3490104171003,-3.64393708624685,
-2.27698460548143));
#25225=CARTESIAN_POINT('Ctrl Pts',(-41.3225520837669,-2.32931941133151,
-4.38081266313611));
#25226=CARTESIAN_POINT('Ctrl Pts',(-41.2960937504336,0.149957969249583,
-4.29423438922274));
#25227=CARTESIAN_POINT('Ctrl Pts',(-41.2696354171003,2.62923534983068,-4.20765611530936));
#25228=CARTESIAN_POINT('Ctrl Pts',(-41.2431770837669,3.79389505549644,-2.0172497837413));
#25229=CARTESIAN_POINT('Ctrl Pts',(-41.2167187504336,4.95855476116219,0.173156547826753));
#25230=CARTESIAN_POINT('Ctrl Pts',(-41.1902604171003,3.64393708624685,2.27698460548143));
#25231=CARTESIAN_POINT('Ctrl Pts',(-41.1638020837669,2.32931941133151,4.38081266313611));
#25232=CARTESIAN_POINT('Ctrl Pts',(-41.1373437504336,-0.149957969249583,
4.29423438922274));
#25233=CARTESIAN_POINT('Origin',(-43.8559375004335,-3.93782229046735E-15,
8.32667268468867E-14));
#25234=CARTESIAN_POINT('',(-40.8198437504336,-0.14995796924958,4.29423438922274));
#25235=CARTESIAN_POINT('',(-40.8595312504336,-0.14995796924958,4.29423438922274));
#25236=CARTESIAN_POINT('',(-43.8559375004333,-0.149957969249592,4.2942343892229));
#25237=CARTESIAN_POINT('Ctrl Pts',(-41.1770312504336,-0.149957969249583,
4.29423438922274));
#25238=CARTESIAN_POINT('Ctrl Pts',(-41.1505729171003,-2.62923534983068,
4.20765611530936));
#25239=CARTESIAN_POINT('Ctrl Pts',(-41.1241145837669,-3.79389505549643,
2.01724978374131));
#25240=CARTESIAN_POINT('Ctrl Pts',(-41.0976562504336,-4.95855476116219,
-0.173156547826752));
#25241=CARTESIAN_POINT('Ctrl Pts',(-41.0711979171003,-3.64393708624685,
-2.27698460548143));
#25242=CARTESIAN_POINT('Ctrl Pts',(-41.0447395837669,-2.32931941133151,
-4.38081266313611));
#25243=CARTESIAN_POINT('Ctrl Pts',(-41.0182812504336,0.149957969249583,
-4.29423438922274));
#25244=CARTESIAN_POINT('Ctrl Pts',(-40.9918229171003,2.62923534983068,-4.20765611530936));
#25245=CARTESIAN_POINT('Ctrl Pts',(-40.9653645837669,3.79389505549643,-2.0172497837413));
#25246=CARTESIAN_POINT('Ctrl Pts',(-40.9389062504336,4.95855476116219,0.173156547826753));
#25247=CARTESIAN_POINT('Ctrl Pts',(-40.9124479171003,3.64393708624685,2.27698460548143));
#25248=CARTESIAN_POINT('Ctrl Pts',(-40.8859895837669,2.32931941133151,4.38081266313611));
#25249=CARTESIAN_POINT('Ctrl Pts',(-40.8595312504336,-0.149957969249583,
4.29423438922274));
#25250=CARTESIAN_POINT('Ctrl Pts',(-41.1373437504336,-0.149957969249583,
4.29423438922274));
#25251=CARTESIAN_POINT('Ctrl Pts',(-41.1108854171003,-2.62923534983068,
4.20765611530936));
#25252=CARTESIAN_POINT('Ctrl Pts',(-41.0844270837669,-3.79389505549643,
2.01724978374131));
#25253=CARTESIAN_POINT('Ctrl Pts',(-41.0579687504336,-4.95855476116219,
-0.173156547826752));
#25254=CARTESIAN_POINT('Ctrl Pts',(-41.0315104171003,-3.64393708624685,
-2.27698460548143));
#25255=CARTESIAN_POINT('Ctrl Pts',(-41.0050520837669,-2.32931941133151,
-4.38081266313611));
#25256=CARTESIAN_POINT('Ctrl Pts',(-40.9785937504336,0.149957969249583,
-4.29423438922274));
#25257=CARTESIAN_POINT('Ctrl Pts',(-40.9521354171003,2.62923534983068,-4.20765611530936));
#25258=CARTESIAN_POINT('Ctrl Pts',(-40.9256770837669,3.79389505549644,-2.0172497837413));
#25259=CARTESIAN_POINT('Ctrl Pts',(-40.8992187504336,4.95855476116219,0.173156547826753));
#25260=CARTESIAN_POINT('Ctrl Pts',(-40.8727604171003,3.64393708624685,2.27698460548143));
#25261=CARTESIAN_POINT('Ctrl Pts',(-40.8463020837669,2.32931941133151,4.38081266313611));
#25262=CARTESIAN_POINT('Ctrl Pts',(-40.8198437504336,-0.149957969249583,
4.29423438922274));
#25263=CARTESIAN_POINT('Origin',(-43.8559375004335,-3.93782229046735E-15,
8.32667268468867E-14));
#25264=CARTESIAN_POINT('',(-40.5023437504336,-0.149957969249579,4.29423438922274));
#25265=CARTESIAN_POINT('',(-40.5420312504336,-0.149957969249579,4.29423438922274));
#25266=CARTESIAN_POINT('',(-43.8559375004333,-0.149957969249592,4.2942343892229));
#25267=CARTESIAN_POINT('Ctrl Pts',(-40.8595312504336,-0.149957969249583,
4.29423438922274));
#25268=CARTESIAN_POINT('Ctrl Pts',(-40.8330729171003,-2.62923534983068,
4.20765611530936));
#25269=CARTESIAN_POINT('Ctrl Pts',(-40.8066145837669,-3.79389505549643,
2.01724978374131));
#25270=CARTESIAN_POINT('Ctrl Pts',(-40.7801562504336,-4.95855476116219,
-0.173156547826752));
#25271=CARTESIAN_POINT('Ctrl Pts',(-40.7536979171003,-3.64393708624685,
-2.27698460548143));
#25272=CARTESIAN_POINT('Ctrl Pts',(-40.7272395837669,-2.32931941133151,
-4.38081266313611));
#25273=CARTESIAN_POINT('Ctrl Pts',(-40.7007812504336,0.149957969249583,
-4.29423438922274));
#25274=CARTESIAN_POINT('Ctrl Pts',(-40.6743229171003,2.62923534983068,-4.20765611530936));
#25275=CARTESIAN_POINT('Ctrl Pts',(-40.6478645837669,3.79389505549643,-2.0172497837413));
#25276=CARTESIAN_POINT('Ctrl Pts',(-40.6214062504336,4.95855476116219,0.173156547826753));
#25277=CARTESIAN_POINT('Ctrl Pts',(-40.5949479171003,3.64393708624685,2.27698460548143));
#25278=CARTESIAN_POINT('Ctrl Pts',(-40.5684895837669,2.32931941133151,4.38081266313611));
#25279=CARTESIAN_POINT('Ctrl Pts',(-40.5420312504336,-0.149957969249583,
4.29423438922274));
#25280=CARTESIAN_POINT('Ctrl Pts',(-40.8198437504336,-0.149957969249583,
4.29423438922274));
#25281=CARTESIAN_POINT('Ctrl Pts',(-40.7933854171003,-2.62923534983068,
4.20765611530936));
#25282=CARTESIAN_POINT('Ctrl Pts',(-40.7669270837669,-3.79389505549643,
2.01724978374131));
#25283=CARTESIAN_POINT('Ctrl Pts',(-40.7404687504336,-4.95855476116219,
-0.173156547826752));
#25284=CARTESIAN_POINT('Ctrl Pts',(-40.7140104171003,-3.64393708624685,
-2.27698460548143));
#25285=CARTESIAN_POINT('Ctrl Pts',(-40.6875520837669,-2.32931941133151,
-4.38081266313611));
#25286=CARTESIAN_POINT('Ctrl Pts',(-40.6610937504336,0.149957969249583,
-4.29423438922274));
#25287=CARTESIAN_POINT('Ctrl Pts',(-40.6346354171003,2.62923534983068,-4.20765611530936));
#25288=CARTESIAN_POINT('Ctrl Pts',(-40.6081770837669,3.79389505549644,-2.0172497837413));
#25289=CARTESIAN_POINT('Ctrl Pts',(-40.5817187504336,4.95855476116219,0.173156547826753));
#25290=CARTESIAN_POINT('Ctrl Pts',(-40.5552604171002,3.64393708624685,2.27698460548143));
#25291=CARTESIAN_POINT('Ctrl Pts',(-40.5288020837669,2.32931941133151,4.38081266313611));
#25292=CARTESIAN_POINT('Ctrl Pts',(-40.5023437504336,-0.149957969249583,
4.29423438922274));
#25293=CARTESIAN_POINT('Origin',(-43.8559375004335,-3.93782229046735E-15,
8.32667268468867E-14));
#25294=CARTESIAN_POINT('',(-40.1848437504336,-0.149957969249579,4.29423438922274));
#25295=CARTESIAN_POINT('',(-40.2245312504336,-0.149957969249579,4.29423438922274));
#25296=CARTESIAN_POINT('',(-43.8559375004333,-0.149957969249592,4.2942343892229));
#25297=CARTESIAN_POINT('Ctrl Pts',(-40.5420312504336,-0.149957969249583,
4.29423438922274));
#25298=CARTESIAN_POINT('Ctrl Pts',(-40.5155729171003,-2.62923534983068,
4.20765611530936));
#25299=CARTESIAN_POINT('Ctrl Pts',(-40.4891145837669,-3.79389505549643,
2.01724978374131));
#25300=CARTESIAN_POINT('Ctrl Pts',(-40.4626562504336,-4.95855476116219,
-0.173156547826752));
#25301=CARTESIAN_POINT('Ctrl Pts',(-40.4361979171003,-3.64393708624685,
-2.27698460548143));
#25302=CARTESIAN_POINT('Ctrl Pts',(-40.4097395837669,-2.32931941133151,
-4.38081266313611));
#25303=CARTESIAN_POINT('Ctrl Pts',(-40.3832812504336,0.149957969249583,
-4.29423438922274));
#25304=CARTESIAN_POINT('Ctrl Pts',(-40.3568229171003,2.62923534983068,-4.20765611530936));
#25305=CARTESIAN_POINT('Ctrl Pts',(-40.3303645837669,3.79389505549643,-2.0172497837413));
#25306=CARTESIAN_POINT('Ctrl Pts',(-40.3039062504336,4.95855476116219,0.173156547826753));
#25307=CARTESIAN_POINT('Ctrl Pts',(-40.2774479171003,3.64393708624685,2.27698460548143));
#25308=CARTESIAN_POINT('Ctrl Pts',(-40.2509895837669,2.32931941133151,4.38081266313611));
#25309=CARTESIAN_POINT('Ctrl Pts',(-40.2245312504336,-0.149957969249583,
4.29423438922274));
#25310=CARTESIAN_POINT('Ctrl Pts',(-40.5023437504336,-0.149957969249583,
4.29423438922274));
#25311=CARTESIAN_POINT('Ctrl Pts',(-40.4758854171003,-2.62923534983068,
4.20765611530936));
#25312=CARTESIAN_POINT('Ctrl Pts',(-40.4494270837669,-3.79389505549643,
2.01724978374131));
#25313=CARTESIAN_POINT('Ctrl Pts',(-40.4229687504336,-4.95855476116219,
-0.173156547826752));
#25314=CARTESIAN_POINT('Ctrl Pts',(-40.3965104171003,-3.64393708624685,
-2.27698460548143));
#25315=CARTESIAN_POINT('Ctrl Pts',(-40.3700520837669,-2.32931941133151,
-4.38081266313611));
#25316=CARTESIAN_POINT('Ctrl Pts',(-40.3435937504336,0.149957969249583,
-4.29423438922274));
#25317=CARTESIAN_POINT('Ctrl Pts',(-40.3171354171003,2.62923534983068,-4.20765611530936));
#25318=CARTESIAN_POINT('Ctrl Pts',(-40.2906770837669,3.79389505549644,-2.0172497837413));
#25319=CARTESIAN_POINT('Ctrl Pts',(-40.2642187504336,4.95855476116219,0.173156547826753));
#25320=CARTESIAN_POINT('Ctrl Pts',(-40.2377604171003,3.64393708624685,2.27698460548143));
#25321=CARTESIAN_POINT('Ctrl Pts',(-40.2113020837669,2.32931941133151,4.38081266313611));
#25322=CARTESIAN_POINT('Ctrl Pts',(-40.1848437504336,-0.149957969249583,
4.29423438922274));
#25323=CARTESIAN_POINT('Origin',(-43.8559375004335,-3.93782229046735E-15,
8.32667268468867E-14));
#25324=CARTESIAN_POINT('',(-39.8673437504336,-0.149957969249578,4.29423438922274));
#25325=CARTESIAN_POINT('',(-39.9070312504336,-0.149957969249578,4.29423438922274));
#25326=CARTESIAN_POINT('',(-43.8559375004333,-0.149957969249592,4.2942343892229));
#25327=CARTESIAN_POINT('Ctrl Pts',(-40.2245312504336,-0.149957969249583,
4.29423438922274));
#25328=CARTESIAN_POINT('Ctrl Pts',(-40.1980729171003,-2.62923534983068,
4.20765611530936));
#25329=CARTESIAN_POINT('Ctrl Pts',(-40.1716145837669,-3.79389505549643,
2.01724978374131));
#25330=CARTESIAN_POINT('Ctrl Pts',(-40.1451562504336,-4.95855476116219,
-0.173156547826752));
#25331=CARTESIAN_POINT('Ctrl Pts',(-40.1186979171003,-3.64393708624685,
-2.27698460548143));
#25332=CARTESIAN_POINT('Ctrl Pts',(-40.0922395837669,-2.32931941133151,
-4.38081266313611));
#25333=CARTESIAN_POINT('Ctrl Pts',(-40.0657812504336,0.149957969249583,
-4.29423438922274));
#25334=CARTESIAN_POINT('Ctrl Pts',(-40.0393229171003,2.62923534983068,-4.20765611530936));
#25335=CARTESIAN_POINT('Ctrl Pts',(-40.0128645837669,3.79389505549643,-2.0172497837413));
#25336=CARTESIAN_POINT('Ctrl Pts',(-39.9864062504336,4.95855476116219,0.173156547826753));
#25337=CARTESIAN_POINT('Ctrl Pts',(-39.9599479171003,3.64393708624685,2.27698460548143));
#25338=CARTESIAN_POINT('Ctrl Pts',(-39.9334895837669,2.32931941133151,4.38081266313611));
#25339=CARTESIAN_POINT('Ctrl Pts',(-39.9070312504336,-0.149957969249583,
4.29423438922274));
#25340=CARTESIAN_POINT('Ctrl Pts',(-40.1848437504336,-0.149957969249583,
4.29423438922274));
#25341=CARTESIAN_POINT('Ctrl Pts',(-40.1583854171003,-2.62923534983068,
4.20765611530936));
#25342=CARTESIAN_POINT('Ctrl Pts',(-40.1319270837669,-3.79389505549643,
2.01724978374131));
#25343=CARTESIAN_POINT('Ctrl Pts',(-40.1054687504336,-4.95855476116219,
-0.173156547826752));
#25344=CARTESIAN_POINT('Ctrl Pts',(-40.0790104171003,-3.64393708624685,
-2.27698460548143));
#25345=CARTESIAN_POINT('Ctrl Pts',(-40.0525520837669,-2.32931941133151,
-4.38081266313611));
#25346=CARTESIAN_POINT('Ctrl Pts',(-40.0260937504336,0.149957969249583,
-4.29423438922274));
#25347=CARTESIAN_POINT('Ctrl Pts',(-39.9996354171003,2.62923534983068,-4.20765611530936));
#25348=CARTESIAN_POINT('Ctrl Pts',(-39.9731770837669,3.79389505549644,-2.0172497837413));
#25349=CARTESIAN_POINT('Ctrl Pts',(-39.9467187504336,4.95855476116219,0.173156547826753));
#25350=CARTESIAN_POINT('Ctrl Pts',(-39.9202604171003,3.64393708624685,2.27698460548143));
#25351=CARTESIAN_POINT('Ctrl Pts',(-39.8938020837669,2.32931941133151,4.38081266313611));
#25352=CARTESIAN_POINT('Ctrl Pts',(-39.8673437504336,-0.149957969249583,
4.29423438922274));
#25353=CARTESIAN_POINT('Origin',(-43.8559375004335,-3.93782229046735E-15,
8.32667268468867E-14));
#25354=CARTESIAN_POINT('',(-39.5498437504336,-0.149957969249578,4.29423438922274));
#25355=CARTESIAN_POINT('',(-39.5895312504336,-0.149957969249578,4.29423438922274));
#25356=CARTESIAN_POINT('',(-43.8559375004333,-0.149957969249592,4.2942343892229));
#25357=CARTESIAN_POINT('Ctrl Pts',(-39.9070312504336,-0.149957969249583,
4.29423438922274));
#25358=CARTESIAN_POINT('Ctrl Pts',(-39.8805729171003,-2.62923534983068,
4.20765611530936));
#25359=CARTESIAN_POINT('Ctrl Pts',(-39.8541145837669,-3.79389505549643,
2.01724978374131));
#25360=CARTESIAN_POINT('Ctrl Pts',(-39.8276562504336,-4.95855476116219,
-0.173156547826752));
#25361=CARTESIAN_POINT('Ctrl Pts',(-39.8011979171003,-3.64393708624685,
-2.27698460548143));
#25362=CARTESIAN_POINT('Ctrl Pts',(-39.7747395837669,-2.32931941133151,
-4.38081266313611));
#25363=CARTESIAN_POINT('Ctrl Pts',(-39.7482812504336,0.149957969249583,
-4.29423438922274));
#25364=CARTESIAN_POINT('Ctrl Pts',(-39.7218229171003,2.62923534983068,-4.20765611530936));
#25365=CARTESIAN_POINT('Ctrl Pts',(-39.6953645837669,3.79389505549643,-2.0172497837413));
#25366=CARTESIAN_POINT('Ctrl Pts',(-39.6689062504336,4.95855476116219,0.173156547826753));
#25367=CARTESIAN_POINT('Ctrl Pts',(-39.6424479171003,3.64393708624685,2.27698460548143));
#25368=CARTESIAN_POINT('Ctrl Pts',(-39.6159895837669,2.32931941133151,4.38081266313611));
#25369=CARTESIAN_POINT('Ctrl Pts',(-39.5895312504336,-0.149957969249583,
4.29423438922274));
#25370=CARTESIAN_POINT('Ctrl Pts',(-39.8673437504336,-0.149957969249583,
4.29423438922274));
#25371=CARTESIAN_POINT('Ctrl Pts',(-39.8408854171003,-2.62923534983068,
4.20765611530936));
#25372=CARTESIAN_POINT('Ctrl Pts',(-39.8144270837669,-3.79389505549643,
2.01724978374131));
#25373=CARTESIAN_POINT('Ctrl Pts',(-39.7879687504336,-4.95855476116219,
-0.173156547826752));
#25374=CARTESIAN_POINT('Ctrl Pts',(-39.7615104171003,-3.64393708624685,
-2.27698460548143));
#25375=CARTESIAN_POINT('Ctrl Pts',(-39.7350520837669,-2.32931941133151,
-4.38081266313611));
#25376=CARTESIAN_POINT('Ctrl Pts',(-39.7085937504336,0.149957969249583,
-4.29423438922274));
#25377=CARTESIAN_POINT('Ctrl Pts',(-39.6821354171003,2.62923534983068,-4.20765611530936));
#25378=CARTESIAN_POINT('Ctrl Pts',(-39.6556770837669,3.79389505549644,-2.0172497837413));
#25379=CARTESIAN_POINT('Ctrl Pts',(-39.6292187504336,4.95855476116219,0.173156547826753));
#25380=CARTESIAN_POINT('Ctrl Pts',(-39.6027604171003,3.64393708624685,2.27698460548143));
#25381=CARTESIAN_POINT('Ctrl Pts',(-39.5763020837669,2.32931941133151,4.38081266313611));
#25382=CARTESIAN_POINT('Ctrl Pts',(-39.5498437504336,-0.149957969249583,
4.29423438922274));
#25383=CARTESIAN_POINT('Origin',(-43.8559375004335,-3.93782229046735E-15,
8.32667268468867E-14));
#25384=CARTESIAN_POINT('',(-39.2323437504336,-0.149957969249577,4.29423438922274));
#25385=CARTESIAN_POINT('',(-39.2720312504336,-0.149957969249577,4.29423438922274));
#25386=CARTESIAN_POINT('',(-43.8559375004333,-0.149957969249592,4.2942343892229));
#25387=CARTESIAN_POINT('Ctrl Pts',(-39.5895312504336,-0.149957969249583,
4.29423438922274));
#25388=CARTESIAN_POINT('Ctrl Pts',(-39.5630729171003,-2.62923534983068,
4.20765611530936));
#25389=CARTESIAN_POINT('Ctrl Pts',(-39.5366145837669,-3.79389505549643,
2.01724978374131));
#25390=CARTESIAN_POINT('Ctrl Pts',(-39.5101562504336,-4.95855476116219,
-0.173156547826752));
#25391=CARTESIAN_POINT('Ctrl Pts',(-39.4836979171003,-3.64393708624685,
-2.27698460548143));
#25392=CARTESIAN_POINT('Ctrl Pts',(-39.4572395837669,-2.32931941133151,
-4.38081266313611));
#25393=CARTESIAN_POINT('Ctrl Pts',(-39.4307812504336,0.149957969249583,
-4.29423438922274));
#25394=CARTESIAN_POINT('Ctrl Pts',(-39.4043229171003,2.62923534983068,-4.20765611530936));
#25395=CARTESIAN_POINT('Ctrl Pts',(-39.3778645837669,3.79389505549643,-2.0172497837413));
#25396=CARTESIAN_POINT('Ctrl Pts',(-39.3514062504336,4.95855476116219,0.173156547826753));
#25397=CARTESIAN_POINT('Ctrl Pts',(-39.3249479171003,3.64393708624685,2.27698460548143));
#25398=CARTESIAN_POINT('Ctrl Pts',(-39.2984895837669,2.32931941133151,4.38081266313611));
#25399=CARTESIAN_POINT('Ctrl Pts',(-39.2720312504336,-0.149957969249583,
4.29423438922274));
#25400=CARTESIAN_POINT('Ctrl Pts',(-39.5498437504336,-0.149957969249583,
4.29423438922274));
#25401=CARTESIAN_POINT('Ctrl Pts',(-39.5233854171003,-2.62923534983068,
4.20765611530936));
#25402=CARTESIAN_POINT('Ctrl Pts',(-39.4969270837669,-3.79389505549643,
2.01724978374131));
#25403=CARTESIAN_POINT('Ctrl Pts',(-39.4704687504336,-4.95855476116219,
-0.173156547826752));
#25404=CARTESIAN_POINT('Ctrl Pts',(-39.4440104171003,-3.64393708624685,
-2.27698460548143));
#25405=CARTESIAN_POINT('Ctrl Pts',(-39.4175520837669,-2.32931941133151,
-4.38081266313611));
#25406=CARTESIAN_POINT('Ctrl Pts',(-39.3910937504336,0.149957969249583,
-4.29423438922274));
#25407=CARTESIAN_POINT('Ctrl Pts',(-39.3646354171003,2.62923534983068,-4.20765611530936));
#25408=CARTESIAN_POINT('Ctrl Pts',(-39.3381770837669,3.79389505549644,-2.0172497837413));
#25409=CARTESIAN_POINT('Ctrl Pts',(-39.3117187504336,4.95855476116219,0.173156547826753));
#25410=CARTESIAN_POINT('Ctrl Pts',(-39.2852604171003,3.64393708624685,2.27698460548143));
#25411=CARTESIAN_POINT('Ctrl Pts',(-39.2588020837669,2.32931941133151,4.38081266313611));
#25412=CARTESIAN_POINT('Ctrl Pts',(-39.2323437504336,-0.149957969249583,
4.29423438922274));
#25413=CARTESIAN_POINT('Origin',(-43.8559375004335,-3.93782229046735E-15,
8.32667268468867E-14));
#25414=CARTESIAN_POINT('',(-38.9148437504336,-0.149957969249577,4.29423438922274));
#25415=CARTESIAN_POINT('',(-38.9545312504336,-0.149957969249577,4.29423438922274));
#25416=CARTESIAN_POINT('',(-43.8559375004333,-0.149957969249592,4.2942343892229));
#25417=CARTESIAN_POINT('Ctrl Pts',(-39.2720312504336,-0.149957969249583,
4.29423438922274));
#25418=CARTESIAN_POINT('Ctrl Pts',(-39.2455729171003,-2.62923534983068,
4.20765611530936));
#25419=CARTESIAN_POINT('Ctrl Pts',(-39.2191145837669,-3.79389505549643,
2.01724978374131));
#25420=CARTESIAN_POINT('Ctrl Pts',(-39.1926562504336,-4.95855476116219,
-0.173156547826752));
#25421=CARTESIAN_POINT('Ctrl Pts',(-39.1661979171003,-3.64393708624685,
-2.27698460548143));
#25422=CARTESIAN_POINT('Ctrl Pts',(-39.1397395837669,-2.32931941133151,
-4.38081266313611));
#25423=CARTESIAN_POINT('Ctrl Pts',(-39.1132812504336,0.149957969249583,
-4.29423438922274));
#25424=CARTESIAN_POINT('Ctrl Pts',(-39.0868229171003,2.62923534983068,-4.20765611530936));
#25425=CARTESIAN_POINT('Ctrl Pts',(-39.0603645837669,3.79389505549643,-2.0172497837413));
#25426=CARTESIAN_POINT('Ctrl Pts',(-39.0339062504336,4.95855476116219,0.173156547826753));
#25427=CARTESIAN_POINT('Ctrl Pts',(-39.0074479171003,3.64393708624685,2.27698460548143));
#25428=CARTESIAN_POINT('Ctrl Pts',(-38.9809895837669,2.32931941133151,4.38081266313611));
#25429=CARTESIAN_POINT('Ctrl Pts',(-38.9545312504336,-0.149957969249583,
4.29423438922274));
#25430=CARTESIAN_POINT('Ctrl Pts',(-39.2323437504336,-0.149957969249583,
4.29423438922274));
#25431=CARTESIAN_POINT('Ctrl Pts',(-39.2058854171003,-2.62923534983068,
4.20765611530936));
#25432=CARTESIAN_POINT('Ctrl Pts',(-39.1794270837669,-3.79389505549643,
2.01724978374131));
#25433=CARTESIAN_POINT('Ctrl Pts',(-39.1529687504336,-4.95855476116219,
-0.173156547826752));
#25434=CARTESIAN_POINT('Ctrl Pts',(-39.1265104171003,-3.64393708624685,
-2.27698460548143));
#25435=CARTESIAN_POINT('Ctrl Pts',(-39.1000520837669,-2.32931941133151,
-4.38081266313611));
#25436=CARTESIAN_POINT('Ctrl Pts',(-39.0735937504336,0.149957969249583,
-4.29423438922274));
#25437=CARTESIAN_POINT('Ctrl Pts',(-39.0471354171003,2.62923534983068,-4.20765611530936));
#25438=CARTESIAN_POINT('Ctrl Pts',(-39.0206770837669,3.79389505549644,-2.0172497837413));
#25439=CARTESIAN_POINT('Ctrl Pts',(-38.9942187504336,4.95855476116219,0.173156547826753));
#25440=CARTESIAN_POINT('Ctrl Pts',(-38.9677604171003,3.64393708624685,2.27698460548143));
#25441=CARTESIAN_POINT('Ctrl Pts',(-38.9413020837669,2.32931941133151,4.38081266313611));
#25442=CARTESIAN_POINT('Ctrl Pts',(-38.9148437504336,-0.149957969249583,
4.29423438922274));
#25443=CARTESIAN_POINT('Origin',(-43.8559375004335,-3.93782229046735E-15,
8.32667268468867E-14));
#25444=CARTESIAN_POINT('',(-38.5973437504336,-0.149957969249576,4.29423438922274));
#25445=CARTESIAN_POINT('',(-38.6370312504336,-0.149957969249576,4.29423438922274));
#25446=CARTESIAN_POINT('',(-43.8559375004333,-0.149957969249592,4.2942343892229));
#25447=CARTESIAN_POINT('Ctrl Pts',(-38.9545312504336,-0.149957969249583,
4.29423438922274));
#25448=CARTESIAN_POINT('Ctrl Pts',(-38.9280729171003,-2.62923534983068,
4.20765611530936));
#25449=CARTESIAN_POINT('Ctrl Pts',(-38.9016145837669,-3.79389505549643,
2.01724978374131));
#25450=CARTESIAN_POINT('Ctrl Pts',(-38.8751562504336,-4.95855476116219,
-0.173156547826752));
#25451=CARTESIAN_POINT('Ctrl Pts',(-38.8486979171003,-3.64393708624685,
-2.27698460548143));
#25452=CARTESIAN_POINT('Ctrl Pts',(-38.8222395837669,-2.32931941133151,
-4.38081266313611));
#25453=CARTESIAN_POINT('Ctrl Pts',(-38.7957812504336,0.149957969249583,
-4.29423438922274));
#25454=CARTESIAN_POINT('Ctrl Pts',(-38.7693229171003,2.62923534983068,-4.20765611530936));
#25455=CARTESIAN_POINT('Ctrl Pts',(-38.7428645837669,3.79389505549643,-2.0172497837413));
#25456=CARTESIAN_POINT('Ctrl Pts',(-38.7164062504336,4.95855476116219,0.173156547826753));
#25457=CARTESIAN_POINT('Ctrl Pts',(-38.6899479171003,3.64393708624685,2.27698460548143));
#25458=CARTESIAN_POINT('Ctrl Pts',(-38.6634895837669,2.32931941133151,4.38081266313611));
#25459=CARTESIAN_POINT('Ctrl Pts',(-38.6370312504336,-0.149957969249583,
4.29423438922274));
#25460=CARTESIAN_POINT('Ctrl Pts',(-38.9148437504336,-0.149957969249583,
4.29423438922274));
#25461=CARTESIAN_POINT('Ctrl Pts',(-38.8883854171003,-2.62923534983068,
4.20765611530936));
#25462=CARTESIAN_POINT('Ctrl Pts',(-38.8619270837669,-3.79389505549643,
2.01724978374131));
#25463=CARTESIAN_POINT('Ctrl Pts',(-38.8354687504336,-4.95855476116219,
-0.173156547826752));
#25464=CARTESIAN_POINT('Ctrl Pts',(-38.8090104171003,-3.64393708624685,
-2.27698460548143));
#25465=CARTESIAN_POINT('Ctrl Pts',(-38.7825520837669,-2.32931941133151,
-4.38081266313611));
#25466=CARTESIAN_POINT('Ctrl Pts',(-38.7560937504336,0.149957969249583,
-4.29423438922274));
#25467=CARTESIAN_POINT('Ctrl Pts',(-38.7296354171002,2.62923534983068,-4.20765611530936));
#25468=CARTESIAN_POINT('Ctrl Pts',(-38.7031770837669,3.79389505549644,-2.0172497837413));
#25469=CARTESIAN_POINT('Ctrl Pts',(-38.6767187504336,4.95855476116219,0.173156547826753));
#25470=CARTESIAN_POINT('Ctrl Pts',(-38.6502604171003,3.64393708624685,2.27698460548143));
#25471=CARTESIAN_POINT('Ctrl Pts',(-38.6238020837669,2.32931941133151,4.38081266313611));
#25472=CARTESIAN_POINT('Ctrl Pts',(-38.5973437504336,-0.149957969249583,
4.29423438922274));
#25473=CARTESIAN_POINT('Origin',(-43.8559375004335,-3.93782229046735E-15,
8.32667268468867E-14));
#25474=CARTESIAN_POINT('',(-38.2798437504336,-0.149957969249576,4.29423438922274));
#25475=CARTESIAN_POINT('',(-38.3195312504336,-0.149957969249576,4.29423438922274));
#25476=CARTESIAN_POINT('',(-43.8559375004333,-0.149957969249592,4.2942343892229));
#25477=CARTESIAN_POINT('Ctrl Pts',(-38.6370312504336,-0.149957969249583,
4.29423438922274));
#25478=CARTESIAN_POINT('Ctrl Pts',(-38.6105729171003,-2.62923534983068,
4.20765611530936));
#25479=CARTESIAN_POINT('Ctrl Pts',(-38.5841145837669,-3.79389505549643,
2.01724978374131));
#25480=CARTESIAN_POINT('Ctrl Pts',(-38.5576562504336,-4.95855476116219,
-0.173156547826752));
#25481=CARTESIAN_POINT('Ctrl Pts',(-38.5311979171003,-3.64393708624685,
-2.27698460548143));
#25482=CARTESIAN_POINT('Ctrl Pts',(-38.5047395837669,-2.32931941133151,
-4.38081266313611));
#25483=CARTESIAN_POINT('Ctrl Pts',(-38.4782812504336,0.149957969249583,
-4.29423438922274));
#25484=CARTESIAN_POINT('Ctrl Pts',(-38.4518229171003,2.62923534983068,-4.20765611530936));
#25485=CARTESIAN_POINT('Ctrl Pts',(-38.4253645837669,3.79389505549643,-2.0172497837413));
#25486=CARTESIAN_POINT('Ctrl Pts',(-38.3989062504336,4.95855476116219,0.173156547826753));
#25487=CARTESIAN_POINT('Ctrl Pts',(-38.3724479171003,3.64393708624685,2.27698460548143));
#25488=CARTESIAN_POINT('Ctrl Pts',(-38.3459895837669,2.32931941133151,4.38081266313611));
#25489=CARTESIAN_POINT('Ctrl Pts',(-38.3195312504336,-0.149957969249583,
4.29423438922274));
#25490=CARTESIAN_POINT('Ctrl Pts',(-38.5973437504336,-0.149957969249583,
4.29423438922274));
#25491=CARTESIAN_POINT('Ctrl Pts',(-38.5708854171003,-2.62923534983068,
4.20765611530936));
#25492=CARTESIAN_POINT('Ctrl Pts',(-38.5444270837669,-3.79389505549643,
2.01724978374131));
#25493=CARTESIAN_POINT('Ctrl Pts',(-38.5179687504336,-4.95855476116219,
-0.173156547826752));
#25494=CARTESIAN_POINT('Ctrl Pts',(-38.4915104171003,-3.64393708624685,
-2.27698460548143));
#25495=CARTESIAN_POINT('Ctrl Pts',(-38.4650520837669,-2.32931941133151,
-4.38081266313611));
#25496=CARTESIAN_POINT('Ctrl Pts',(-38.4385937504336,0.149957969249583,
-4.29423438922274));
#25497=CARTESIAN_POINT('Ctrl Pts',(-38.4121354171003,2.62923534983068,-4.20765611530936));
#25498=CARTESIAN_POINT('Ctrl Pts',(-38.3856770837669,3.79389505549644,-2.0172497837413));
#25499=CARTESIAN_POINT('Ctrl Pts',(-38.3592187504336,4.95855476116219,0.173156547826753));
#25500=CARTESIAN_POINT('Ctrl Pts',(-38.3327604171003,3.64393708624685,2.27698460548143));
#25501=CARTESIAN_POINT('Ctrl Pts',(-38.3063020837669,2.32931941133151,4.38081266313611));
#25502=CARTESIAN_POINT('Ctrl Pts',(-38.2798437504336,-0.149957969249583,
4.29423438922274));
#25503=CARTESIAN_POINT('Origin',(-43.8559375004335,-3.93782229046735E-15,
8.32667268468867E-14));
#25504=CARTESIAN_POINT('',(-37.9623437504336,-0.149957969249575,4.29423438922274));
#25505=CARTESIAN_POINT('',(-38.0020312504336,-0.149957969249575,4.29423438922274));
#25506=CARTESIAN_POINT('',(-43.8559375004333,-0.149957969249592,4.2942343892229));
#25507=CARTESIAN_POINT('Ctrl Pts',(-38.3195312504336,-0.149957969249583,
4.29423438922274));
#25508=CARTESIAN_POINT('Ctrl Pts',(-38.2930729171002,-2.62923534983068,
4.20765611530936));
#25509=CARTESIAN_POINT('Ctrl Pts',(-38.2666145837669,-3.79389505549643,
2.01724978374131));
#25510=CARTESIAN_POINT('Ctrl Pts',(-38.2401562504336,-4.95855476116219,
-0.173156547826752));
#25511=CARTESIAN_POINT('Ctrl Pts',(-38.2136979171003,-3.64393708624685,
-2.27698460548143));
#25512=CARTESIAN_POINT('Ctrl Pts',(-38.1872395837669,-2.32931941133151,
-4.38081266313611));
#25513=CARTESIAN_POINT('Ctrl Pts',(-38.1607812504336,0.149957969249583,
-4.29423438922274));
#25514=CARTESIAN_POINT('Ctrl Pts',(-38.1343229171002,2.62923534983068,-4.20765611530936));
#25515=CARTESIAN_POINT('Ctrl Pts',(-38.1078645837669,3.79389505549643,-2.0172497837413));
#25516=CARTESIAN_POINT('Ctrl Pts',(-38.0814062504336,4.95855476116219,0.173156547826753));
#25517=CARTESIAN_POINT('Ctrl Pts',(-38.0549479171003,3.64393708624685,2.27698460548143));
#25518=CARTESIAN_POINT('Ctrl Pts',(-38.0284895837669,2.32931941133151,4.38081266313611));
#25519=CARTESIAN_POINT('Ctrl Pts',(-38.0020312504336,-0.149957969249583,
4.29423438922274));
#25520=CARTESIAN_POINT('Ctrl Pts',(-38.2798437504336,-0.149957969249583,
4.29423438922274));
#25521=CARTESIAN_POINT('Ctrl Pts',(-38.2533854171003,-2.62923534983068,
4.20765611530936));
#25522=CARTESIAN_POINT('Ctrl Pts',(-38.2269270837669,-3.79389505549643,
2.01724978374131));
#25523=CARTESIAN_POINT('Ctrl Pts',(-38.2004687504336,-4.95855476116219,
-0.173156547826752));
#25524=CARTESIAN_POINT('Ctrl Pts',(-38.1740104171002,-3.64393708624685,
-2.27698460548143));
#25525=CARTESIAN_POINT('Ctrl Pts',(-38.1475520837669,-2.32931941133151,
-4.38081266313611));
#25526=CARTESIAN_POINT('Ctrl Pts',(-38.1210937504336,0.149957969249583,
-4.29423438922274));
#25527=CARTESIAN_POINT('Ctrl Pts',(-38.0946354171003,2.62923534983068,-4.20765611530936));
#25528=CARTESIAN_POINT('Ctrl Pts',(-38.0681770837669,3.79389505549644,-2.0172497837413));
#25529=CARTESIAN_POINT('Ctrl Pts',(-38.0417187504336,4.95855476116219,0.173156547826753));
#25530=CARTESIAN_POINT('Ctrl Pts',(-38.0152604171003,3.64393708624685,2.27698460548143));
#25531=CARTESIAN_POINT('Ctrl Pts',(-37.9888020837669,2.32931941133151,4.38081266313611));
#25532=CARTESIAN_POINT('Ctrl Pts',(-37.9623437504336,-0.149957969249583,
4.29423438922274));
#25533=CARTESIAN_POINT('Origin',(-43.8559375004335,-3.93782229046735E-15,
8.32667268468867E-14));
#25534=CARTESIAN_POINT('',(-37.6448437504336,-0.149957969249575,4.29423438922274));
#25535=CARTESIAN_POINT('',(-37.6845312504336,-0.149957969249575,4.29423438922274));
#25536=CARTESIAN_POINT('',(-43.8559375004333,-0.149957969249592,4.2942343892229));
#25537=CARTESIAN_POINT('Ctrl Pts',(-38.0020312504336,-0.149957969249583,
4.29423438922274));
#25538=CARTESIAN_POINT('Ctrl Pts',(-37.9755729171003,-2.62923534983068,
4.20765611530936));
#25539=CARTESIAN_POINT('Ctrl Pts',(-37.9491145837669,-3.79389505549643,
2.01724978374131));
#25540=CARTESIAN_POINT('Ctrl Pts',(-37.9226562504336,-4.95855476116219,
-0.173156547826752));
#25541=CARTESIAN_POINT('Ctrl Pts',(-37.8961979171003,-3.64393708624685,
-2.27698460548143));
#25542=CARTESIAN_POINT('Ctrl Pts',(-37.8697395837669,-2.32931941133151,
-4.38081266313611));
#25543=CARTESIAN_POINT('Ctrl Pts',(-37.8432812504336,0.149957969249583,
-4.29423438922274));
#25544=CARTESIAN_POINT('Ctrl Pts',(-37.8168229171003,2.62923534983068,-4.20765611530936));
#25545=CARTESIAN_POINT('Ctrl Pts',(-37.7903645837669,3.79389505549643,-2.0172497837413));
#25546=CARTESIAN_POINT('Ctrl Pts',(-37.7639062504336,4.95855476116219,0.173156547826753));
#25547=CARTESIAN_POINT('Ctrl Pts',(-37.7374479171003,3.64393708624685,2.27698460548143));
#25548=CARTESIAN_POINT('Ctrl Pts',(-37.7109895837669,2.32931941133151,4.38081266313611));
#25549=CARTESIAN_POINT('Ctrl Pts',(-37.6845312504336,-0.149957969249583,
4.29423438922274));
#25550=CARTESIAN_POINT('Ctrl Pts',(-37.9623437504336,-0.149957969249583,
4.29423438922274));
#25551=CARTESIAN_POINT('Ctrl Pts',(-37.9358854171002,-2.62923534983068,
4.20765611530936));
#25552=CARTESIAN_POINT('Ctrl Pts',(-37.9094270837669,-3.79389505549643,
2.01724978374131));
#25553=CARTESIAN_POINT('Ctrl Pts',(-37.8829687504336,-4.95855476116219,
-0.173156547826752));
#25554=CARTESIAN_POINT('Ctrl Pts',(-37.8565104171003,-3.64393708624685,
-2.27698460548143));
#25555=CARTESIAN_POINT('Ctrl Pts',(-37.8300520837669,-2.32931941133151,
-4.38081266313611));
#25556=CARTESIAN_POINT('Ctrl Pts',(-37.8035937504336,0.149957969249583,
-4.29423438922274));
#25557=CARTESIAN_POINT('Ctrl Pts',(-37.7771354171003,2.62923534983068,-4.20765611530936));
#25558=CARTESIAN_POINT('Ctrl Pts',(-37.7506770837669,3.79389505549644,-2.0172497837413));
#25559=CARTESIAN_POINT('Ctrl Pts',(-37.7242187504336,4.95855476116219,0.173156547826753));
#25560=CARTESIAN_POINT('Ctrl Pts',(-37.6977604171003,3.64393708624685,2.27698460548143));
#25561=CARTESIAN_POINT('Ctrl Pts',(-37.6713020837669,2.32931941133151,4.38081266313611));
#25562=CARTESIAN_POINT('Ctrl Pts',(-37.6448437504336,-0.149957969249583,
4.29423438922274));
#25563=CARTESIAN_POINT('Origin',(-43.8559375004335,-3.93782229046735E-15,
8.32667268468867E-14));
#25564=CARTESIAN_POINT('',(-37.3273437504336,-0.149957969249574,4.29423438922274));
#25565=CARTESIAN_POINT('',(-37.3670312504336,-0.149957969249574,4.29423438922274));
#25566=CARTESIAN_POINT('',(-43.8559375004333,-0.149957969249592,4.2942343892229));
#25567=CARTESIAN_POINT('Ctrl Pts',(-37.6845312504336,-0.149957969249583,
4.29423438922274));
#25568=CARTESIAN_POINT('Ctrl Pts',(-37.6580729171003,-2.62923534983068,
4.20765611530936));
#25569=CARTESIAN_POINT('Ctrl Pts',(-37.6316145837669,-3.79389505549643,
2.01724978374131));
#25570=CARTESIAN_POINT('Ctrl Pts',(-37.6051562504336,-4.95855476116219,
-0.173156547826752));
#25571=CARTESIAN_POINT('Ctrl Pts',(-37.5786979171003,-3.64393708624685,
-2.27698460548143));
#25572=CARTESIAN_POINT('Ctrl Pts',(-37.5522395837669,-2.32931941133151,
-4.38081266313611));
#25573=CARTESIAN_POINT('Ctrl Pts',(-37.5257812504336,0.149957969249583,
-4.29423438922274));
#25574=CARTESIAN_POINT('Ctrl Pts',(-37.4993229171003,2.62923534983068,-4.20765611530936));
#25575=CARTESIAN_POINT('Ctrl Pts',(-37.4728645837669,3.79389505549643,-2.0172497837413));
#25576=CARTESIAN_POINT('Ctrl Pts',(-37.4464062504336,4.95855476116219,0.173156547826753));
#25577=CARTESIAN_POINT('Ctrl Pts',(-37.4199479171003,3.64393708624685,2.27698460548143));
#25578=CARTESIAN_POINT('Ctrl Pts',(-37.3934895837669,2.32931941133151,4.38081266313611));
#25579=CARTESIAN_POINT('Ctrl Pts',(-37.3670312504336,-0.149957969249583,
4.29423438922274));
#25580=CARTESIAN_POINT('Ctrl Pts',(-37.6448437504336,-0.149957969249583,
4.29423438922274));
#25581=CARTESIAN_POINT('Ctrl Pts',(-37.6183854171003,-2.62923534983068,
4.20765611530936));
#25582=CARTESIAN_POINT('Ctrl Pts',(-37.5919270837669,-3.79389505549643,
2.01724978374131));
#25583=CARTESIAN_POINT('Ctrl Pts',(-37.5654687504336,-4.95855476116219,
-0.173156547826752));
#25584=CARTESIAN_POINT('Ctrl Pts',(-37.5390104171003,-3.64393708624685,
-2.27698460548143));
#25585=CARTESIAN_POINT('Ctrl Pts',(-37.5125520837669,-2.32931941133151,
-4.38081266313611));
#25586=CARTESIAN_POINT('Ctrl Pts',(-37.4860937504336,0.149957969249583,
-4.29423438922274));
#25587=CARTESIAN_POINT('Ctrl Pts',(-37.4596354171003,2.62923534983068,-4.20765611530936));
#25588=CARTESIAN_POINT('Ctrl Pts',(-37.4331770837669,3.79389505549644,-2.0172497837413));
#25589=CARTESIAN_POINT('Ctrl Pts',(-37.4067187504336,4.95855476116219,0.173156547826753));
#25590=CARTESIAN_POINT('Ctrl Pts',(-37.3802604171003,3.64393708624685,2.27698460548143));
#25591=CARTESIAN_POINT('Ctrl Pts',(-37.3538020837669,2.32931941133151,4.38081266313611));
#25592=CARTESIAN_POINT('Ctrl Pts',(-37.3273437504336,-0.149957969249583,
4.29423438922274));
#25593=CARTESIAN_POINT('Origin',(-43.8559375004335,-3.93782229046735E-15,
8.32667268468867E-14));
#25594=CARTESIAN_POINT('',(-37.0098437504336,-0.149957969249574,4.29423438922274));
#25595=CARTESIAN_POINT('',(-37.0495312504336,-0.149957969249574,4.29423438922274));
#25596=CARTESIAN_POINT('',(-43.8559375004333,-0.149957969249592,4.2942343892229));
#25597=CARTESIAN_POINT('Ctrl Pts',(-37.3670312504336,-0.149957969249583,
4.29423438922274));
#25598=CARTESIAN_POINT('Ctrl Pts',(-37.3405729171003,-2.62923534983068,
4.20765611530936));
#25599=CARTESIAN_POINT('Ctrl Pts',(-37.3141145837669,-3.79389505549643,
2.01724978374131));
#25600=CARTESIAN_POINT('Ctrl Pts',(-37.2876562504336,-4.95855476116219,
-0.173156547826752));
#25601=CARTESIAN_POINT('Ctrl Pts',(-37.2611979171003,-3.64393708624685,
-2.27698460548143));
#25602=CARTESIAN_POINT('Ctrl Pts',(-37.2347395837669,-2.32931941133151,
-4.38081266313611));
#25603=CARTESIAN_POINT('Ctrl Pts',(-37.2082812504336,0.149957969249583,
-4.29423438922274));
#25604=CARTESIAN_POINT('Ctrl Pts',(-37.1818229171003,2.62923534983068,-4.20765611530936));
#25605=CARTESIAN_POINT('Ctrl Pts',(-37.1553645837669,3.79389505549643,-2.0172497837413));
#25606=CARTESIAN_POINT('Ctrl Pts',(-37.1289062504336,4.95855476116219,0.173156547826753));
#25607=CARTESIAN_POINT('Ctrl Pts',(-37.1024479171003,3.64393708624685,2.27698460548143));
#25608=CARTESIAN_POINT('Ctrl Pts',(-37.0759895837669,2.32931941133151,4.38081266313611));
#25609=CARTESIAN_POINT('Ctrl Pts',(-37.0495312504336,-0.149957969249583,
4.29423438922274));
#25610=CARTESIAN_POINT('Ctrl Pts',(-37.3273437504336,-0.149957969249583,
4.29423438922274));
#25611=CARTESIAN_POINT('Ctrl Pts',(-37.3008854171003,-2.62923534983068,
4.20765611530936));
#25612=CARTESIAN_POINT('Ctrl Pts',(-37.2744270837669,-3.79389505549643,
2.01724978374131));
#25613=CARTESIAN_POINT('Ctrl Pts',(-37.2479687504336,-4.95855476116219,
-0.173156547826752));
#25614=CARTESIAN_POINT('Ctrl Pts',(-37.2215104171003,-3.64393708624685,
-2.27698460548143));
#25615=CARTESIAN_POINT('Ctrl Pts',(-37.1950520837669,-2.32931941133151,
-4.38081266313611));
#25616=CARTESIAN_POINT('Ctrl Pts',(-37.1685937504336,0.149957969249583,
-4.29423438922274));
#25617=CARTESIAN_POINT('Ctrl Pts',(-37.1421354171003,2.62923534983068,-4.20765611530936));
#25618=CARTESIAN_POINT('Ctrl Pts',(-37.1156770837669,3.79389505549644,-2.0172497837413));
#25619=CARTESIAN_POINT('Ctrl Pts',(-37.0892187504336,4.95855476116219,0.173156547826753));
#25620=CARTESIAN_POINT('Ctrl Pts',(-37.0627604171003,3.64393708624685,2.27698460548143));
#25621=CARTESIAN_POINT('Ctrl Pts',(-37.0363020837669,2.32931941133151,4.38081266313611));
#25622=CARTESIAN_POINT('Ctrl Pts',(-37.0098437504336,-0.149957969249583,
4.29423438922274));
#25623=CARTESIAN_POINT('Origin',(-43.8559375004335,-3.93782229046735E-15,
8.32667268468867E-14));
#25624=CARTESIAN_POINT('',(-36.6923437504336,-0.149957969249573,4.29423438922274));
#25625=CARTESIAN_POINT('',(-36.7320312504336,-0.149957969249573,4.29423438922274));
#25626=CARTESIAN_POINT('',(-43.8559375004333,-0.149957969249592,4.2942343892229));
#25627=CARTESIAN_POINT('Ctrl Pts',(-37.0495312504336,-0.149957969249583,
4.29423438922274));
#25628=CARTESIAN_POINT('Ctrl Pts',(-37.0230729171003,-2.62923534983068,
4.20765611530936));
#25629=CARTESIAN_POINT('Ctrl Pts',(-36.9966145837669,-3.79389505549643,
2.01724978374131));
#25630=CARTESIAN_POINT('Ctrl Pts',(-36.9701562504336,-4.95855476116219,
-0.173156547826752));
#25631=CARTESIAN_POINT('Ctrl Pts',(-36.9436979171003,-3.64393708624685,
-2.27698460548143));
#25632=CARTESIAN_POINT('Ctrl Pts',(-36.9172395837669,-2.32931941133151,
-4.38081266313611));
#25633=CARTESIAN_POINT('Ctrl Pts',(-36.8907812504336,0.149957969249583,
-4.29423438922274));
#25634=CARTESIAN_POINT('Ctrl Pts',(-36.8643229171003,2.62923534983068,-4.20765611530936));
#25635=CARTESIAN_POINT('Ctrl Pts',(-36.8378645837669,3.79389505549643,-2.0172497837413));
#25636=CARTESIAN_POINT('Ctrl Pts',(-36.8114062504336,4.95855476116219,0.173156547826753));
#25637=CARTESIAN_POINT('Ctrl Pts',(-36.7849479171003,3.64393708624685,2.27698460548143));
#25638=CARTESIAN_POINT('Ctrl Pts',(-36.7584895837669,2.32931941133151,4.38081266313611));
#25639=CARTESIAN_POINT('Ctrl Pts',(-36.7320312504336,-0.149957969249583,
4.29423438922274));
#25640=CARTESIAN_POINT('Ctrl Pts',(-37.0098437504336,-0.149957969249583,
4.29423438922274));
#25641=CARTESIAN_POINT('Ctrl Pts',(-36.9833854171003,-2.62923534983068,
4.20765611530936));
#25642=CARTESIAN_POINT('Ctrl Pts',(-36.9569270837669,-3.79389505549643,
2.01724978374131));
#25643=CARTESIAN_POINT('Ctrl Pts',(-36.9304687504336,-4.95855476116219,
-0.173156547826752));
#25644=CARTESIAN_POINT('Ctrl Pts',(-36.9040104171003,-3.64393708624685,
-2.27698460548143));
#25645=CARTESIAN_POINT('Ctrl Pts',(-36.8775520837669,-2.32931941133151,
-4.38081266313611));
#25646=CARTESIAN_POINT('Ctrl Pts',(-36.8510937504336,0.149957969249583,
-4.29423438922274));
#25647=CARTESIAN_POINT('Ctrl Pts',(-36.8246354171003,2.62923534983068,-4.20765611530936));
#25648=CARTESIAN_POINT('Ctrl Pts',(-36.7981770837669,3.79389505549644,-2.0172497837413));
#25649=CARTESIAN_POINT('Ctrl Pts',(-36.7717187504336,4.95855476116219,0.173156547826753));
#25650=CARTESIAN_POINT('Ctrl Pts',(-36.7452604171003,3.64393708624685,2.27698460548143));
#25651=CARTESIAN_POINT('Ctrl Pts',(-36.7188020837669,2.32931941133151,4.38081266313611));
#25652=CARTESIAN_POINT('Ctrl Pts',(-36.6923437504336,-0.149957969249583,
4.29423438922274));
#25653=CARTESIAN_POINT('Origin',(-43.8559375004335,-3.93782229046735E-15,
8.32667268468867E-14));
#25654=CARTESIAN_POINT('',(-36.3748437504336,-0.149957969249573,4.29423438922274));
#25655=CARTESIAN_POINT('',(-36.4145312504336,-0.149957969249573,4.29423438922274));
#25656=CARTESIAN_POINT('',(-43.8559375004333,-0.149957969249592,4.2942343892229));
#25657=CARTESIAN_POINT('Ctrl Pts',(-36.7320312504336,-0.149957969249583,
4.29423438922274));
#25658=CARTESIAN_POINT('Ctrl Pts',(-36.7055729171003,-2.62923534983068,
4.20765611530936));
#25659=CARTESIAN_POINT('Ctrl Pts',(-36.6791145837669,-3.79389505549643,
2.01724978374131));
#25660=CARTESIAN_POINT('Ctrl Pts',(-36.6526562504336,-4.95855476116219,
-0.173156547826752));
#25661=CARTESIAN_POINT('Ctrl Pts',(-36.6261979171003,-3.64393708624685,
-2.27698460548143));
#25662=CARTESIAN_POINT('Ctrl Pts',(-36.5997395837669,-2.32931941133151,
-4.38081266313611));
#25663=CARTESIAN_POINT('Ctrl Pts',(-36.5732812504336,0.149957969249583,
-4.29423438922274));
#25664=CARTESIAN_POINT('Ctrl Pts',(-36.5468229171003,2.62923534983068,-4.20765611530936));
#25665=CARTESIAN_POINT('Ctrl Pts',(-36.5203645837669,3.79389505549643,-2.0172497837413));
#25666=CARTESIAN_POINT('Ctrl Pts',(-36.4939062504336,4.95855476116219,0.173156547826753));
#25667=CARTESIAN_POINT('Ctrl Pts',(-36.4674479171003,3.64393708624685,2.27698460548143));
#25668=CARTESIAN_POINT('Ctrl Pts',(-36.4409895837669,2.32931941133151,4.38081266313611));
#25669=CARTESIAN_POINT('Ctrl Pts',(-36.4145312504336,-0.149957969249583,
4.29423438922274));
#25670=CARTESIAN_POINT('Ctrl Pts',(-36.6923437504336,-0.149957969249583,
4.29423438922274));
#25671=CARTESIAN_POINT('Ctrl Pts',(-36.6658854171003,-2.62923534983068,
4.20765611530936));
#25672=CARTESIAN_POINT('Ctrl Pts',(-36.6394270837669,-3.79389505549643,
2.01724978374131));
#25673=CARTESIAN_POINT('Ctrl Pts',(-36.6129687504336,-4.95855476116219,
-0.173156547826752));
#25674=CARTESIAN_POINT('Ctrl Pts',(-36.5865104171002,-3.64393708624685,
-2.27698460548143));
#25675=CARTESIAN_POINT('Ctrl Pts',(-36.5600520837669,-2.32931941133151,
-4.38081266313611));
#25676=CARTESIAN_POINT('Ctrl Pts',(-36.5335937504336,0.149957969249583,
-4.29423438922274));
#25677=CARTESIAN_POINT('Ctrl Pts',(-36.5071354171003,2.62923534983068,-4.20765611530936));
#25678=CARTESIAN_POINT('Ctrl Pts',(-36.4806770837669,3.79389505549644,-2.0172497837413));
#25679=CARTESIAN_POINT('Ctrl Pts',(-36.4542187504336,4.95855476116219,0.173156547826753));
#25680=CARTESIAN_POINT('Ctrl Pts',(-36.4277604171003,3.64393708624685,2.27698460548143));
#25681=CARTESIAN_POINT('Ctrl Pts',(-36.4013020837669,2.32931941133151,4.38081266313611));
#25682=CARTESIAN_POINT('Ctrl Pts',(-36.3748437504336,-0.149957969249583,
4.29423438922274));
#25683=CARTESIAN_POINT('Origin',(-43.8559375004335,-3.93782229046735E-15,
8.32667268468867E-14));
#25684=CARTESIAN_POINT('',(-36.0573437504336,-0.149957969249572,4.29423438922274));
#25685=CARTESIAN_POINT('',(-36.0970312504336,-0.149957969249572,4.29423438922274));
#25686=CARTESIAN_POINT('',(-43.8559375004333,-0.149957969249592,4.2942343892229));
#25687=CARTESIAN_POINT('',(-36.,-3.96679264203451,1.65151219106173));
#25688=CARTESIAN_POINT('Ctrl Pts',(-36.0573437504336,-0.149957969249583,
4.29423438922274));
#25689=CARTESIAN_POINT('Ctrl Pts',(-36.0308854171003,-2.62923534983068,
4.20765611530936));
#25690=CARTESIAN_POINT('Ctrl Pts',(-36.0044270837669,-3.79389505549643,
2.01724978374131));
#25691=CARTESIAN_POINT('Ctrl Pts',(-36.0022673883541,-3.88896189860283,
1.83845505593417));
#25692=CARTESIAN_POINT('Ctrl Pts',(-36.,-3.96679264203451,1.65151219106173));
#25693=CARTESIAN_POINT('',(-36.,-3.99810942017506,-1.57418469260506));
#25694=CARTESIAN_POINT('Origin',(-35.9999999999998,1.55431223447522E-14,
3.88578058618805E-15));
#25695=CARTESIAN_POINT('Ctrl Pts',(-36.0970312504336,-0.149957969249583,
4.29423438922274));
#25696=CARTESIAN_POINT('Ctrl Pts',(-36.0705729171003,-2.62923534983068,
4.20765611530936));
#25697=CARTESIAN_POINT('Ctrl Pts',(-36.0441145837669,-3.79389505549643,
2.01724978374131));
#25698=CARTESIAN_POINT('Ctrl Pts',(-36.0229922517456,-4.72367126947973,
0.268595051253399));
#25699=CARTESIAN_POINT('Ctrl Pts',(-36.,-3.99810942017506,-1.57418469260506));
#25700=CARTESIAN_POINT('Origin',(-44.,0.,0.));
#25701=CARTESIAN_POINT('',(-43.6591154631359,-2.96734935548908E-14,-4.12499999999999));
#25702=CARTESIAN_POINT('',(-43.975,-5.05166804648283E-16,-4.125));
#25703=CARTESIAN_POINT('',(-44.,-5.05166804648282E-16,-4.12499999999999));
#25704=CARTESIAN_POINT('',(-43.975,0.143960423897816,-4.12248716145376));
#25705=CARTESIAN_POINT('Origin',(-43.975,0.,0.));
#25706=CARTESIAN_POINT('Ctrl Pts',(-43.975,0.143960423897817,-4.12248716145376));
#25707=CARTESIAN_POINT('Ctrl Pts',(-43.97183047655,0.42908205717337,-4.11253049462104));
#25708=CARTESIAN_POINT('Ctrl Pts',(-43.9684796639578,0.712401235868628,
-4.07302110630467));
#25709=CARTESIAN_POINT('Ctrl Pts',(-43.9614044274671,1.27578409938326,-3.93383307652861));
#25710=CARTESIAN_POINT('Ctrl Pts',(-43.9576915174157,1.5537851359483,-3.83254723024597));
#25711=CARTESIAN_POINT('Ctrl Pts',(-43.9469595135523,2.30860116593424,-3.46179456351789));
#25712=CARTESIAN_POINT('Ctrl Pts',(-43.9399198814115,2.74599034187203,-3.12621199461402));
#25713=CARTESIAN_POINT('Ctrl Pts',(-43.926701044641,3.45463635345407,-2.31575107321194));
#25714=CARTESIAN_POINT('Ctrl Pts',(-43.9210432976051,3.72358343109977,-1.85260371719902));
#25715=CARTESIAN_POINT('Ctrl Pts',(-43.9083349580575,4.07146299165201,-0.849201559422838));
#25716=CARTESIAN_POINT('Ctrl Pts',(-43.9015615552565,4.1468869566712,-0.318240438634118));
#25717=CARTESIAN_POINT('Ctrl Pts',(-43.8877402455277,4.09140360287742,0.757887952165817));
#25718=CARTESIAN_POINT('Ctrl Pts',(-43.8808265278912,3.95520891889208,1.29240378216373));
#25719=CARTESIAN_POINT('Ctrl Pts',(-43.8682704646471,3.49291086949633,2.2556363213478));
#25720=CARTESIAN_POINT('Ctrl Pts',(-43.862586857156,3.17960346670654,2.67926241239808));
#25721=CARTESIAN_POINT('Ctrl Pts',(-43.8494371722728,2.40047974876652,3.39736504387608));
#25722=CARTESIAN_POINT('Ctrl Pts',(-43.8424910107108,1.93795931290139,3.68085640262762));
#25723=CARTESIAN_POINT('Ctrl Pts',(-43.8287169242127,0.922157190792934,
4.05750959759151));
#25724=CARTESIAN_POINT('Ctrl Pts',(-43.8220687964696,0.37758007752296,4.1438107711559));
#25725=CARTESIAN_POINT('Ctrl Pts',(-43.8101464836354,-0.691107827936443,
4.1002599887138));
#25726=CARTESIAN_POINT('Ctrl Pts',(-43.8037303692132,-1.20543875210143,
3.97953133305015));
#25727=CARTESIAN_POINT('Ctrl Pts',(-43.7901672681873,-2.17995049430338,
3.54390218815809));
#25728=CARTESIAN_POINT('Ctrl Pts',(-43.7831344521376,-2.62771130704635,
3.22592037575174));
#25729=CARTESIAN_POINT('Ctrl Pts',(-43.7697429236182,-3.36811592255533,
2.44088035666596));
#25730=CARTESIAN_POINT('Ctrl Pts',(-43.7639441873864,-3.65607854757604,
1.98373089093437));
#25731=CARTESIAN_POINT('Ctrl Pts',(-43.7513792883756,-4.039229064548,0.990285445042111));
#25732=CARTESIAN_POINT('Ctrl Pts',(-43.7446755248126,-4.13287097726785,
0.464120018982602));
#25733=CARTESIAN_POINT('Ctrl Pts',(-43.7308201405905,-4.11575799333123,
-0.616006114386392));
#25734=CARTESIAN_POINT('Ctrl Pts',(-43.7238005094659,-3.99684332011726,
-1.15938665648937));
#25735=CARTESIAN_POINT('Ctrl Pts',(-43.7110028898235,-3.56364185673055,
-2.14247673551862));
#25736=CARTESIAN_POINT('Ctrl Pts',(-43.7053995962841,-3.2632209128958,-2.57704110067067));
#25737=CARTESIAN_POINT('Ctrl Pts',(-43.6923686904007,-2.50729211492382,
-3.31904453736047));
#25738=CARTESIAN_POINT('Ctrl Pts',(-43.6854620394096,-2.05555241197391,
-3.61625102775665));
#25739=CARTESIAN_POINT('Ctrl Pts',(-43.6717983243574,-1.06445018626301,
-4.02103149758079));
#25740=CARTESIAN_POINT('Ctrl Pts',(-43.665171886146,-0.534703156090073,
-4.12499999999998));
#25741=CARTESIAN_POINT('Ctrl Pts',(-43.6591154631359,-5.91193760612896E-14,
-4.12499999999999));
#25742=CARTESIAN_POINT('Origin',(-44.,0.,0.));
#25743=CARTESIAN_POINT('',(-43.3416154631359,-7.91110547264604E-17,-4.12499999999999));
#25744=CARTESIAN_POINT('',(-43.4209904640031,1.3975723041988E-15,-4.12499999999999));
#25745=CARTESIAN_POINT('',(-44.,-5.05166804648282E-16,-4.12499999999999));
#25746=CARTESIAN_POINT('',(-43.7368750008672,0.143960423897816,-4.12248716145376));
#25747=CARTESIAN_POINT('Ctrl Pts',(-43.4209904640031,2.15305958091061E-15,
-4.12499999999999));
#25748=CARTESIAN_POINT('Ctrl Pts',(-43.4217841869206,-0.0700753808536829,
-4.12499999999999));
#25749=CARTESIAN_POINT('Ctrl Pts',(-43.4225893565914,-0.140211920515319,
-4.12321436266605));
#25750=CARTESIAN_POINT('Ctrl Pts',(-43.4297513900091,-0.755813543173842,
-4.09178269975688));
#25751=CARTESIAN_POINT('Ctrl Pts',(-43.4366245347121,-1.29035673936744,
-3.9558704357677));
#25752=CARTESIAN_POINT('Ctrl Pts',(-43.4504515973494,-2.26318535354331,
-3.48959947740471));
#25753=CARTESIAN_POINT('Ctrl Pts',(-43.4572693723953,-2.69439006697297,
-3.16852957206712));
#25754=CARTESIAN_POINT('Ctrl Pts',(-43.4700762553883,-3.40773676952694,
-2.38363843237575));
#25755=CARTESIAN_POINT('Ctrl Pts',(-43.4756773460284,-3.68454947045869,
-1.92834064584949));
#25756=CARTESIAN_POINT('Ctrl Pts',(-43.4887723270657,-4.0581868735389,-0.919976274451078));
#25757=CARTESIAN_POINT('Ctrl Pts',(-43.4958111522624,-4.14432035210699,
-0.373953844976087));
#25758=CARTESIAN_POINT('Ctrl Pts',(-43.5095479626073,-4.09929622803357,
0.699093369405077));
#25759=CARTESIAN_POINT('Ctrl Pts',(-43.5161225895255,-3.97666071527261,
1.21619858092205));
#25760=CARTESIAN_POINT('Ctrl Pts',(-43.5284456204229,-3.53610661035621,
2.19278282575447));
#25761=CARTESIAN_POINT('Ctrl Pts',(-43.5346273063288,-3.2159594271141,2.64006840117702));
#25762=CARTESIAN_POINT('Ctrl Pts',(-43.548289156452,-2.42346414910966,3.38151107493627));
#25763=CARTESIAN_POINT('Ctrl Pts',(-43.5552899990205,-1.95998718715836,
3.66963839353035));
#25764=CARTESIAN_POINT('Ctrl Pts',(-43.568648828934,-0.966014596552634,
4.04407476096784));
#25765=CARTESIAN_POINT('Ctrl Pts',(-43.5746204731358,-0.447397812110882,
4.13370889184485));
#25766=CARTESIAN_POINT('Ctrl Pts',(-43.5868280322708,0.620166584767352,
4.11451824490259));
#25767=CARTESIAN_POINT('Ctrl Pts',(-43.5936410341835,1.15884306831965,3.99636589021096));
#25768=CARTESIAN_POINT('Ctrl Pts',(-43.6074622740015,2.1480569720669,3.56187802156145));
#25769=CARTESIAN_POINT('Ctrl Pts',(-43.6143324413542,2.59089238020419,3.25398286351057));
#25770=CARTESIAN_POINT('Ctrl Pts',(-43.6272659039809,3.32812620798997,2.49299913232278));
#25771=CARTESIAN_POINT('Ctrl Pts',(-43.6328450895579,3.61818537549182,2.04943959497307));
#25772=CARTESIAN_POINT('Ctrl Pts',(-43.6457747740852,4.0254168025233,1.05514152540184));
#25773=CARTESIAN_POINT('Ctrl Pts',(-43.6528057791958,4.12999005714525,0.510372995931821));
#25774=CARTESIAN_POINT('Ctrl Pts',(-43.6666147684555,4.11984170736092,-0.567086304521003));
#25775=CARTESIAN_POINT('Ctrl Pts',(-43.6732645340858,4.01344136503595,-1.08948541134691));
#25776=CARTESIAN_POINT('Ctrl Pts',(-43.6857251858634,3.60524496755625,-2.07567416616227));
#25777=CARTESIAN_POINT('Ctrl Pts',(-43.6916675575682,3.30343334572731,-2.52854662486236));
#25778=CARTESIAN_POINT('Ctrl Pts',(-43.7049785336112,2.55166504379906,-3.28355142682418));
#25779=CARTESIAN_POINT('Ctrl Pts',(-43.7117878594451,2.11226815661032,-3.58204221900527));
#25780=CARTESIAN_POINT('Ctrl Pts',(-43.724947801425,1.15867261640002,-3.9918383467642));
#25781=CARTESIAN_POINT('Ctrl Pts',(-43.7311919121336,0.655195493564536,
-4.10463443942983));
#25782=CARTESIAN_POINT('Ctrl Pts',(-43.7368750008672,0.143960423897816,
-4.12248716145376));
#25783=CARTESIAN_POINT('',(-43.8559375004336,0.143960423897816,-4.12248716145376));
#25784=CARTESIAN_POINT('Origin',(-43.975,0.,0.));
#25785=CARTESIAN_POINT('Ctrl Pts',(-43.6591154631359,-5.88152861126802E-14,
-4.12499999999999));
#25786=CARTESIAN_POINT('Ctrl Pts',(-43.6589893495955,0.0111341806831491,
-4.12499999999999));
#25787=CARTESIAN_POINT('Ctrl Pts',(-43.6588634832089,0.0222705103512012,
-4.12495492002788));
#25788=CARTESIAN_POINT('Ctrl Pts',(-43.6528491033062,0.555558413132617,
-4.12063563480334));
#25789=CARTESIAN_POINT('Ctrl Pts',(-43.6466866748295,1.07219509882857,-4.01729972547807));
#25790=CARTESIAN_POINT('Ctrl Pts',(-43.6332360135605,2.05777766494,-3.61592783690613));
#25791=CARTESIAN_POINT('Ctrl Pts',(-43.6262179313814,2.51456795578323,-3.31456360783142));
#25792=CARTESIAN_POINT('Ctrl Pts',(-43.6126724826772,3.2842264042745,-2.5536973745261));
#25793=CARTESIAN_POINT('Ctrl Pts',(-43.6066817918365,3.59009962015523,-2.10206847694175));
#25794=CARTESIAN_POINT('Ctrl Pts',(-43.5942516665281,4.00554134652347,-1.118007782556));
#25795=CARTESIAN_POINT('Ctrl Pts',(-43.5876182065664,4.11560219486197,-0.596752694620666));
#25796=CARTESIAN_POINT('Ctrl Pts',(-43.5738241914443,4.13359553106555,0.479812571999722));
#25797=CARTESIAN_POINT('Ctrl Pts',(-43.5667907652833,4.03316101536502,1.02491447200937));
#25798=CARTESIAN_POINT('Ctrl Pts',(-43.5538235392921,3.63344749912529,2.02240331718184));
#25799=CARTESIAN_POINT('Ctrl Pts',(-43.5482445740158,3.34636672711171,2.46857976389889));
#25800=CARTESIAN_POINT('Ctrl Pts',(-43.5353393944105,2.61450760049208,3.23497562268258));
#25801=CARTESIAN_POINT('Ctrl Pts',(-43.5284804597234,2.17426530363052,3.5458826013205));
#25802=CARTESIAN_POINT('Ctrl Pts',(-43.5146565723004,1.18866196397726,3.98760057133189));
#25803=CARTESIAN_POINT('Ctrl Pts',(-43.5078293194862,0.650866351281966,
4.10977587436382));
#25804=CARTESIAN_POINT('Ctrl Pts',(-43.4955762826235,-0.416478607119255,
4.13693051141778));
#25805=CARTESIAN_POINT('Ctrl Pts',(-43.4896521368969,-0.935687040047014,
4.051190919213));
#25806=CARTESIAN_POINT('Ctrl Pts',(-43.4763198279506,-1.93199439036745,
3.68439226432171));
#25807=CARTESIAN_POINT('Ctrl Pts',(-43.4693247754649,-2.39730049356399,
3.40004392262083));
#25808=CARTESIAN_POINT('Ctrl Pts',(-43.4556306941763,-3.19624375915856,
2.66417888234778));
#25809=CARTESIAN_POINT('Ctrl Pts',(-43.4493885733127,-3.52047080129217,
2.21812931962595));
#25810=CARTESIAN_POINT('Ctrl Pts',(-43.4370960977028,-3.96810446840913,
1.24368117175732));
#25811=CARTESIAN_POINT('Ctrl Pts',(-43.4305386941905,-4.09425198481728,
0.727796748705689));
#25812=CARTESIAN_POINT('Ctrl Pts',(-43.416819479703,-4.14684849979684,-0.34414241772645));
#25813=CARTESIAN_POINT('Ctrl Pts',(-43.4097799656186,-4.06473266900419,
-0.890358879991509));
#25814=CARTESIAN_POINT('Ctrl Pts',(-43.3966496446118,-3.69845197366426,
-1.9017366805059));
#25815=CARTESIAN_POINT('Ctrl Pts',(-43.3910360105349,-3.42452061952142,
-2.3596201642345));
#25816=CARTESIAN_POINT('Ctrl Pts',(-43.3782569044449,-2.71636030568324,
-3.14965330502464));
#25817=CARTESIAN_POINT('Ctrl Pts',(-43.3714513328493,-2.28771552358482,
-3.47351143594485));
#25818=CARTESIAN_POINT('Ctrl Pts',(-43.3576250115465,-1.31855718802831,
-3.94656209058349));
#25819=CARTESIAN_POINT('Ctrl Pts',(-43.3507398923813,-0.784984740112883,
-4.08628834955838));
#25820=CARTESIAN_POINT('Ctrl Pts',(-43.3434394408746,-0.159800277789472,
-4.12268075233252));
#25821=CARTESIAN_POINT('Ctrl Pts',(-43.3425200419099,-0.0798625070550304,
-4.12499999999999));
#25822=CARTESIAN_POINT('Ctrl Pts',(-43.3416154631359,-1.12029116405105E-15,
-4.12499999999999));
#25823=CARTESIAN_POINT('Origin',(-44.,0.,0.));
#25824=CARTESIAN_POINT('',(-43.0241154623315,3.55101082989618E-8,-4.12499999999999));
#25825=CARTESIAN_POINT('',(-43.1034904640031,1.43537882654006E-14,-4.12499999999999));
#25826=CARTESIAN_POINT('',(-44.,-5.05166804648282E-16,-4.12499999999999));
#25827=CARTESIAN_POINT('Ctrl Pts',(-43.1034904640031,2.66800470605233E-14,
-4.12499999999999));
#25828=CARTESIAN_POINT('Ctrl Pts',(-43.1052759746021,-0.157637296951777,
-4.12499999999999));
#25829=CARTESIAN_POINT('Ctrl Pts',(-43.1071177918741,-0.315441248402036,
-4.11596406793883));
#25830=CARTESIAN_POINT('Ctrl Pts',(-43.1155801821711,-1.01938953197842,
-4.03477234996318));
#25831=CARTESIAN_POINT('Ctrl Pts',(-43.1226029500698,-1.54803169098638,
-3.86291787270377));
#25832=CARTESIAN_POINT('Ctrl Pts',(-43.1364480328831,-2.48824646386089,
-3.33231706468981));
#25833=CARTESIAN_POINT('Ctrl Pts',(-43.1431392580727,-2.89481536520694,
-2.98592673132087));
#25834=CARTESIAN_POINT('Ctrl Pts',(-43.1556794793951,-3.55911665894801,
-2.15307206131927));
#25835=CARTESIAN_POINT('Ctrl Pts',(-43.1615091733841,-3.80851942528891,
-1.67278633352888));
#25836=CARTESIAN_POINT('Ctrl Pts',(-43.1749294953952,-4.11166775494155,
-0.63658374513006));
#25837=CARTESIAN_POINT('Ctrl Pts',(-43.181960207216,-4.15968428344299,-0.0898630879483996));
#25838=CARTESIAN_POINT('Ctrl Pts',(-43.1955032704882,-4.04319752992879,
0.970567332147449));
#25839=CARTESIAN_POINT('Ctrl Pts',(-43.2019012030249,-3.88760292525187,
1.47511599045853));
#25840=CARTESIAN_POINT('Ctrl Pts',(-43.2137810015111,-3.38549162281178,
2.4191248825152));
#25841=CARTESIAN_POINT('Ctrl Pts',(-43.2204822457843,-3.03593416215933,
2.84548968059295));
#25842=CARTESIAN_POINT('Ctrl Pts',(-43.2342625605633,-2.19802302773201,
3.53167830687168));
#25843=CARTESIAN_POINT('Ctrl Pts',(-43.2412020406226,-1.72003210358548,
3.78755181652603));
#25844=CARTESIAN_POINT('Ctrl Pts',(-43.2543303665285,-0.706898517967219,
4.09741633258318));
#25845=CARTESIAN_POINT('Ctrl Pts',(-43.2599952700414,-0.182841721369498,
4.15392485974037));
#25846=CARTESIAN_POINT('Ctrl Pts',(-43.27258568614,0.882197411269908,4.06641392686791));
#25847=CARTESIAN_POINT('Ctrl Pts',(-43.2795082293,1.41232328103033,3.9139915817091));
#25848=CARTESIAN_POINT('Ctrl Pts',(-43.293326935015,2.36887210151711,3.41849039809921));
#25849=CARTESIAN_POINT('Ctrl Pts',(-43.3000894237945,2.78883430396983,3.08545633642643));
#25850=CARTESIAN_POINT('Ctrl Pts',(-43.3127744739824,3.47957156632881,2.27827258369358));
#25851=CARTESIAN_POINT('Ctrl Pts',(-43.3184504853474,3.74379956401648,1.81160442420162));
#25852=CARTESIAN_POINT('Ctrl Pts',(-43.3316979749886,4.08519911444116,0.790218569659973));
#25853=CARTESIAN_POINT('Ctrl Pts',(-43.3387371374263,4.1537902969791,0.243557244814858));
#25854=CARTESIAN_POINT('Ctrl Pts',(-43.352392196471,4.07577218433711,-0.824265521417086));
#25855=CARTESIAN_POINT('Ctrl Pts',(-43.3588893768645,3.93786891142691,-1.33586304490966));
#25856=CARTESIAN_POINT('Ctrl Pts',(-43.3710773892195,3.46630909135439,-2.30299855020026));
#25857=CARTESIAN_POINT('Ctrl Pts',(-43.3775451400705,3.12810928621691,-2.74482226760805));
#25858=CARTESIAN_POINT('Ctrl Pts',(-43.3913460634929,2.30735339026894,-3.46149660931171));
#25859=CARTESIAN_POINT('Ctrl Pts',(-43.398318482974,1.83605538028894,-3.73292651099064));
#25860=CARTESIAN_POINT('Ctrl Pts',(-43.4106822940254,0.898449640878296,
-4.05119835744849));
#25861=CARTESIAN_POINT('Ctrl Pts',(-43.4158878772981,0.450491851513638,
-4.12499999999999));
#25862=CARTESIAN_POINT('Ctrl Pts',(-43.4209904640031,2.15305958091061E-15,
-4.12499999999999));
#25863=CARTESIAN_POINT('Ctrl Pts',(-43.3416154631359,-1.12029116405105E-15,
-4.12499999999999));
#25864=CARTESIAN_POINT('Ctrl Pts',(-43.3366238909621,0.440690716415442,
-4.12499999999999));
#25865=CARTESIAN_POINT('Ctrl Pts',(-43.3315395690574,0.879083534272734,
-4.05437460853012));
#25866=CARTESIAN_POINT('Ctrl Pts',(-43.3193225167226,1.8093221609183,-3.74590157636243));
#25867=CARTESIAN_POINT('Ctrl Pts',(-43.312357155907,2.28221507838271,-3.47806241162083));
#25868=CARTESIAN_POINT('Ctrl Pts',(-43.2986058700743,3.10428455213175,-2.77079207616584));
#25869=CARTESIAN_POINT('Ctrl Pts',(-43.2921143504653,3.44344052223974,-2.33593029491167));
#25870=CARTESIAN_POINT('Ctrl Pts',(-43.2800569829449,3.92299988165074,-1.3787057721374));
#25871=CARTESIAN_POINT('Ctrl Pts',(-43.2735890934869,4.06635403816314,-0.869202600509911));
#25872=CARTESIAN_POINT('Ctrl Pts',(-43.2599665762459,4.1561992094172,0.196494906175366));
#25873=CARTESIAN_POINT('Ctrl Pts',(-43.2529289889307,4.09391972913349,0.743253780537866));
#25874=CARTESIAN_POINT('Ctrl Pts',(-43.2396277769611,3.76419938548784,1.76923783817601));
#25875=CARTESIAN_POINT('Ctrl Pts',(-43.2339121132508,3.50450765055868,2.24004991540411));
#25876=CARTESIAN_POINT('Ctrl Pts',(-43.2212712597041,2.82188654574836,3.05515937030567));
#25877=CARTESIAN_POINT('Ctrl Pts',(-43.2145299107476,2.40600978151607,3.39236689111578));
#25878=CARTESIAN_POINT('Ctrl Pts',(-43.2006455938717,1.45053478435525,3.90078195707088));
#25879=CARTESIAN_POINT('Ctrl Pts',(-43.1936374133849,0.916266102859524,
4.05963233795626));
#25880=CARTESIAN_POINT('Ctrl Pts',(-43.1809398703271,-0.153985615878453,
4.15512756988326));
#25881=CARTESIAN_POINT('Ctrl Pts',(-43.1752949016246,-0.678687930182376,
4.10221674084147));
#25882=CARTESIAN_POINT('Ctrl Pts',(-43.1621921889391,-1.69380827193884,
3.79929948284872));
#25883=CARTESIAN_POINT('Ctrl Pts',(-43.1552609706994,-2.17323075061218,
3.54693227843849));
#25884=CARTESIAN_POINT('Ctrl Pts',(-43.1414729074834,-3.01571167852317,
2.8669170315091));
#25885=CARTESIAN_POINT('Ctrl Pts',(-43.1347555624722,-3.36829176801628,
2.44302098258961));
#25886=CARTESIAN_POINT('Ctrl Pts',(-43.1228311727003,-3.87691226534231,
1.5028694643996));
#25887=CARTESIAN_POINT('Ctrl Pts',(-43.1164997074165,-4.03602609781071,
0.99979001300251));
#25888=CARTESIAN_POINT('Ctrl Pts',(-43.1029809855698,-4.16018275602907,
-0.0590096082767586));
#25889=CARTESIAN_POINT('Ctrl Pts',(-43.0959531158827,-4.11628346110768,
-0.605652355224156));
#25890=CARTESIAN_POINT('Ctrl Pts',(-43.0824990114904,-3.82085591578393,
-1.64475959424927));
#25891=CARTESIAN_POINT('Ctrl Pts',(-43.0766301501403,-3.57443671439989,
-2.12780920288455));
#25892=CARTESIAN_POINT('Ctrl Pts',(-43.0641191842593,-2.91542104739757,
-2.96574701170689));
#25893=CARTESIAN_POINT('Ctrl Pts',(-43.0574430227019,-2.51155811526016,
-3.31472531301843));
#25894=CARTESIAN_POINT('Ctrl Pts',(-43.0436107066202,-1.57581142100035,
-3.85160952045626));
#25895=CARTESIAN_POINT('Ctrl Pts',(-43.0365845808552,-1.04883828179103,
-4.02716051968696));
#25896=CARTESIAN_POINT('Ctrl Pts',(-43.0279803506855,-0.335775072933513,
-4.11476116179616));
#25897=CARTESIAN_POINT('Ctrl Pts',(-43.0260161096807,-0.167802299982725,
-4.12500000144471));
#25898=CARTESIAN_POINT('Ctrl Pts',(-43.0241154627337,3.55147232455888E-8,
-4.12499999999999));
#25899=CARTESIAN_POINT('Origin',(-44.,0.,0.));
#25900=CARTESIAN_POINT('',(-42.7066154631359,-2.40364051253538E-15,-4.12499999999999));
#25901=CARTESIAN_POINT('',(-42.7859904640031,-1.53620248780821E-14,-4.12499999999999));
#25902=CARTESIAN_POINT('',(-44.,-5.05166804648282E-16,-4.12499999999999));
#25903=CARTESIAN_POINT('Ctrl Pts',(-42.7859904640031,-3.47638584585752E-14,
-4.12499999999999));
#25904=CARTESIAN_POINT('Ctrl Pts',(-42.7888245165898,-0.250209878029857,
-4.12499999999999));
#25905=CARTESIAN_POINT('Ctrl Pts',(-42.7917962670083,-0.500472261515978,
-4.10223490248918));
#25906=CARTESIAN_POINT('Ctrl Pts',(-42.8015560655256,-1.28523165018734,
-3.95760041622189));
#25907=CARTESIAN_POINT('Ctrl Pts',(-42.8085958753329,-1.79778204456973,
-3.75265203123737));
#25908=CARTESIAN_POINT('Ctrl Pts',(-42.8222999930062,-2.69584454212555,
-3.16618068502911));
#25909=CARTESIAN_POINT('Ctrl Pts',(-42.8288428847336,-3.07719487032833,
-2.79699093818034));
#25910=CARTESIAN_POINT('Ctrl Pts',(-42.8411098637959,-3.69279084440484,
-1.9179050173747));
#25911=CARTESIAN_POINT('Ctrl Pts',(-42.8474043707732,-3.9143712156974,-1.41165644113701));
#25912=CARTESIAN_POINT('Ctrl Pts',(-42.8611250097368,-4.14545751488401,
-0.349512587343389));
#25913=CARTESIAN_POINT('Ctrl Pts',(-42.8681149403688,-4.15557646971381,
0.195350538477975));
#25914=CARTESIAN_POINT('Ctrl Pts',(-42.881425017066,-3.96860979414112,1.24006915556839));
#25915=CARTESIAN_POINT('Ctrl Pts',(-42.8873118844221,-3.78019612553688,
1.73139937857128));
#25916=CARTESIAN_POINT('Ctrl Pts',(-42.8996027432266,-3.21734484665115,
2.63867222791108));
#25917=CARTESIAN_POINT('Ctrl Pts',(-42.9064416027748,-2.84011387612309,
3.04099378338463));
#25918=CARTESIAN_POINT('Ctrl Pts',(-42.9202671056224,-1.96109074647784,
3.66803676823795));
#25919=CARTESIAN_POINT('Ctrl Pts',(-42.9271163877112,-1.47064201769888,
3.89070522371206));
#25920=CARTESIAN_POINT('Ctrl Pts',(-42.9399978038948,-0.439333279023981,
4.1351622341229));
#25921=CARTESIAN_POINT('Ctrl Pts',(-42.9455788864246,0.0912667879587264,
4.15743317289483));
#25922=CARTESIAN_POINT('Ctrl Pts',(-42.9585773827393,1.15412200234955,3.99805577246191));
#25923=CARTESIAN_POINT('Ctrl Pts',(-42.9656125412644,1.6748987435772,3.80935121142002));
#25924=CARTESIAN_POINT('Ctrl Pts',(-42.9793934583387,2.59426481170688,3.250194003948));
#25925=CARTESIAN_POINT('Ctrl Pts',(-42.9860130016714,2.98827660915105,2.89208950765888));
#25926=CARTESIAN_POINT('Ctrl Pts',(-42.9984173813874,3.62818198206529,2.03590841524423));
#25927=CARTESIAN_POINT('Ctrl Pts',(-43.0044509665188,3.86374723920393,1.54275460734297));
#25928=CARTESIAN_POINT('Ctrl Pts',(-43.0180248816437,4.13105728843214,0.493320214040006));
#25929=CARTESIAN_POINT('Ctrl Pts',(-43.0250392589146,4.16007352615153,-0.0527898485888066));
#25930=CARTESIAN_POINT('Ctrl Pts',(-43.0384680104133,4.00822866347273,-1.10553865169403));
#25931=CARTESIAN_POINT('Ctrl Pts',(-43.0445811221813,3.83631078108773,-1.60337691310156));
#25932=CARTESIAN_POINT('Ctrl Pts',(-43.056666822505,3.30398722598507,-2.52932488849252));
#25933=CARTESIAN_POINT('Ctrl Pts',(-43.0634400914866,2.94051137861696,-2.94401066815298));
#25934=CARTESIAN_POINT('Ctrl Pts',(-43.0772505199682,2.08171497497243,-3.6012056953707));
#25935=CARTESIAN_POINT('Ctrl Pts',(-43.0841488103069,1.59727264490132,-3.84069566259819));
#25936=CARTESIAN_POINT('Ctrl Pts',(-43.0952134104074,0.727707799486982,
-4.07673776869245));
#25937=CARTESIAN_POINT('Ctrl Pts',(-43.0993641378131,0.364300781693087,
-4.12499999999999));
#25938=CARTESIAN_POINT('Ctrl Pts',(-43.1034904640031,2.68869879372251E-14,
-4.12499999999999));
#25939=CARTESIAN_POINT('Ctrl Pts',(-43.0241154627337,3.55147231723032E-8,
-4.12499999999999));
#25940=CARTESIAN_POINT('Ctrl Pts',(-43.0201000493006,0.354508669064718,
-4.1249999969478));
#25941=CARTESIAN_POINT('Ctrl Pts',(-43.0160674581826,0.708253156444587,
-4.07929759244896));
#25942=CARTESIAN_POINT('Ctrl Pts',(-43.005151345896,1.56964374183415,-3.85201695055881));
#25943=CARTESIAN_POINT('Ctrl Pts',(-42.9982631939178,2.05545173993792,-3.61620389309265));
#25944=CARTESIAN_POINT('Ctrl Pts',(-42.9844481153621,2.91877349526748,-2.96556690220725));
#25945=CARTESIAN_POINT('Ctrl Pts',(-42.9776597934361,3.28530187692224,-2.55355186408069));
#25946=CARTESIAN_POINT('Ctrl Pts',(-42.9655287220031,3.82433839284296,-1.63167264176363));
#25947=CARTESIAN_POINT('Ctrl Pts',(-42.9594706776355,3.99988166706038,-1.13528834876725));
#25948=CARTESIAN_POINT('Ctrl Pts',(-42.9460677647307,4.1595007036321,-0.0842834828703053));
#25949=CARTESIAN_POINT('Ctrl Pts',(-42.9390580901803,4.13466688486896,0.461605819570947));
#25950=CARTESIAN_POINT('Ctrl Pts',(-42.9254511705147,3.87532109108673,1.51389269394917));
#25951=CARTESIAN_POINT('Ctrl Pts',(-42.9193648073432,3.64282907543009,2.00991867577158));
#25952=CARTESIAN_POINT('Ctrl Pts',(-42.9069906288836,3.00829785461101,2.87119235244729));
#25953=CARTESIAN_POINT('Ctrl Pts',(-42.9003875970296,2.61707371796781,3.23179805054191));
#25954=CARTESIAN_POINT('Ctrl Pts',(-42.8866225796335,1.70237454360611,3.79709236858559));
#25955=CARTESIAN_POINT('Ctrl Pts',(-42.8795857432846,1.1833843510517,3.9894355309398));
#25956=CARTESIAN_POINT('Ctrl Pts',(-42.8665510177599,0.121543390730149,
4.15673609487457));
#25957=CARTESIAN_POINT('Ctrl Pts',(-42.8609648298656,-0.409834881232685,
4.13826813090633));
#25958=CARTESIAN_POINT('Ctrl Pts',(-42.8481111837364,-1.44306283468347,
3.90096756669595));
#25959=CARTESIAN_POINT('Ctrl Pts',(-42.8412734251041,-1.93473515675691,
3.68195240576325));
#25960=CARTESIAN_POINT('Ctrl Pts',(-42.8274467266498,-2.81799138172734,
3.06150791209393));
#25961=CARTESIAN_POINT('Ctrl Pts',(-42.8205947213512,-3.19813918176695,
2.66192047922009));
#25962=CARTESIAN_POINT('Ctrl Pts',(-42.8082601062542,-3.76756140231514,
1.75872664932032));
#25963=CARTESIAN_POINT('Ctrl Pts',(-42.8024138241952,-3.95953098506463,
1.26876331708425));
#25964=CARTESIAN_POINT('Ctrl Pts',(-42.7891296672012,-4.15398136719704,
0.22580510709411));
#25965=CARTESIAN_POINT('Ctrl Pts',(-42.7821460098025,-4.14788774154854,
-0.318709272419962));
#25966=CARTESIAN_POINT('Ctrl Pts',(-42.7683949303322,-3.92460064974471,
-1.38349984832726));
#25967=CARTESIAN_POINT('Ctrl Pts',(-42.7620374185745,-3.70603558555749,
-1.89257731912303));
#25968=CARTESIAN_POINT('Ctrl Pts',(-42.7498000358233,-3.09562961199559,
-2.77650993271348));
#25969=CARTESIAN_POINT('Ctrl Pts',(-42.7432741437303,-2.71699806369652,
-3.14799028012294));
#25970=CARTESIAN_POINT('Ctrl Pts',(-42.7295880116923,-1.823544844846,-3.74014401885518));
#25971=CARTESIAN_POINT('Ctrl Pts',(-42.7225481710413,-1.31279735592544,
-3.94848829724771));
#25972=CARTESIAN_POINT('Ctrl Pts',(-42.7126518238129,-0.519869054439207,
-4.10043233476657));
#25973=CARTESIAN_POINT('Ctrl Pts',(-42.7095595751266,-0.259926687862678,
-4.12499999999999));
#25974=CARTESIAN_POINT('Ctrl Pts',(-42.7066154631359,-2.77555756156289E-16,
-4.12499999999999));
#25975=CARTESIAN_POINT('Origin',(-44.,0.,0.));
#25976=CARTESIAN_POINT('',(-42.3891154631359,-2.19547369541817E-15,-4.12499999999999));
#25977=CARTESIAN_POINT('',(-42.4684904640031,1.15782307038377E-14,-4.12499999999999));
#25978=CARTESIAN_POINT('',(-44.,-5.05166804648282E-16,-4.12499999999999));
#25979=CARTESIAN_POINT('Ctrl Pts',(-42.4684904640031,2.16493489801906E-14,
-4.12499999999999));
#25980=CARTESIAN_POINT('Ctrl Pts',(-42.4724362677784,-0.348363007083697,
-4.12499999999999));
#25981=CARTESIAN_POINT('Ctrl Pts',(-42.4766406552945,-0.696090583128804,
-4.08086874866564));
#25982=CARTESIAN_POINT('Ctrl Pts',(-42.4877762594709,-1.56016154950479,
-3.85695389900486));
#25983=CARTESIAN_POINT('Ctrl Pts',(-42.4948011956894,-2.05355245920538,
-3.61844142857051));
#25984=CARTESIAN_POINT('Ctrl Pts',(-42.5082974697846,-2.90361541835705,
-2.97620717943818));
#25985=CARTESIAN_POINT('Ctrl Pts',(-42.5145704841859,-3.25697037235858,
-2.58474681575524));
#25986=CARTESIAN_POINT('Ctrl Pts',(-42.5265356262334,-3.81079775100409,
-1.67080256498323));
#25987=CARTESIAN_POINT('Ctrl Pts',(-42.5332674465324,-3.99825409380244,
-1.15226487328355));
#25988=CARTESIAN_POINT('Ctrl Pts',(-42.5470620051222,-4.15891699238856,
-0.0818960292318208));
#25989=CARTESIAN_POINT('Ctrl Pts',(-42.5539853576718,-4.13432363969937,
0.458986168573618));
#25990=CARTESIAN_POINT('Ctrl Pts',(-42.5670644201357,-3.8826671044889,1.48794463240853));
#25991=CARTESIAN_POINT('Ctrl Pts',(-42.5726933681788,-3.66296944596519,
1.9676726110332));
#25992=CARTESIAN_POINT('Ctrl Pts',(-42.5854241355369,-3.03953589276337,
2.84270545807145));
#25993=CARTESIAN_POINT('Ctrl Pts',(-42.5924363794386,-2.63269427749126,
3.22314544875958));
#25994=CARTESIAN_POINT('Ctrl Pts',(-42.6063116669039,-1.71170506016576,
3.79035212504384));
#25995=CARTESIAN_POINT('Ctrl Pts',(-42.6130408464765,-1.21088314117952,
3.97875255600666));
#25996=CARTESIAN_POINT('Ctrl Pts',(-42.6256567611582,-0.162105593265999,
4.15619753914953));
#25997=CARTESIAN_POINT('Ctrl Pts',(-42.6313976429439,0.376227252487634,
4.1423075269595));
#25998=CARTESIAN_POINT('Ctrl Pts',(-42.6447287902611,1.42854328412835,3.90787423126925));
#25999=CARTESIAN_POINT('Ctrl Pts',(-42.6517650968985,1.93143647261353,3.68534496256726));
#26000=CARTESIAN_POINT('Ctrl Pts',(-42.6653685882037,2.80503073811873,3.06956393080499));
#26001=CARTESIAN_POINT('Ctrl Pts',(-42.671819676093,3.17202630260548,2.68862024117154));
#26002=CARTESIAN_POINT('Ctrl Pts',(-42.683833022173,3.75560589010962,1.79143439236175));
#26003=CARTESIAN_POINT('Ctrl Pts',(-42.6903743154332,3.95951954397787,1.27907690494286));
#26004=CARTESIAN_POINT('Ctrl Pts',(-42.7041335991802,4.15449872894309,0.212657859332945));
#26005=CARTESIAN_POINT('Ctrl Pts',(-42.7110928844457,4.14679344901288,-0.330437355567603));
#26006=CARTESIAN_POINT('Ctrl Pts',(-42.7242864692273,3.92666265703818,-1.36722768807397));
#26007=CARTESIAN_POINT('Ctrl Pts',(-42.730014556812,3.72237025880694,-1.85255123012292));
#26008=CARTESIAN_POINT('Ctrl Pts',(-42.7424993207356,3.13022561702276,-2.7414689395802));
#26009=CARTESIAN_POINT('Ctrl Pts',(-42.7493940681355,2.7401188756063,-3.13140622944548));
#26010=CARTESIAN_POINT('Ctrl Pts',(-42.7632192418648,1.84256598940375,-3.7287469907487));
#26011=CARTESIAN_POINT('Ctrl Pts',(-42.7700144866968,1.34685573561633,-3.93504619916284));
#26012=CARTESIAN_POINT('Ctrl Pts',(-42.7797493595055,0.553324077123309,
-4.09715985949721));
#26013=CARTESIAN_POINT('Ctrl Pts',(-42.7828564229322,0.276694948344091,
-4.12499999999999));
#26014=CARTESIAN_POINT('Ctrl Pts',(-42.7859904640031,-3.44139441956932E-14,
-4.12499999999999));
#26015=CARTESIAN_POINT('Ctrl Pts',(-42.7066154631359,-1.12029116405105E-15,
-4.12499999999999));
#26016=CARTESIAN_POINT('Ctrl Pts',(-42.7035833111296,0.267699472910892,
-4.12499999999999));
#26017=CARTESIAN_POINT('Ctrl Pts',(-42.7005816690409,0.535380873838965,
-4.09894073043939));
#26018=CARTESIAN_POINT('Ctrl Pts',(-42.6909831651212,1.32075710604345,-3.94383594341831));
#26019=CARTESIAN_POINT('Ctrl Pts',(-42.6842000643013,1.81750192394942,-3.74097880526701));
#26020=CARTESIAN_POINT('Ctrl Pts',(-42.670376808526,2.71880892727669,-3.14992802416122));
#26021=CARTESIAN_POINT('Ctrl Pts',(-42.6634712901854,3.11156008564056,-2.76263824749651));
#26022=CARTESIAN_POINT('Ctrl Pts',(-42.6509464481592,3.70981792363214,-1.87760808468546));
#26023=CARTESIAN_POINT('Ctrl Pts',(-42.6452442989327,3.91743447999407,-1.39351081816239));
#26024=CARTESIAN_POINT('Ctrl Pts',(-42.6320753195121,4.14442330981951,-0.358400222540147));
#26025=CARTESIAN_POINT('Ctrl Pts',(-42.6251232878707,4.15580827963938,0.184257705315122));
#26026=CARTESIAN_POINT('Ctrl Pts',(-42.6113554379963,3.96828355277432,1.25160522660637));
#26027=CARTESIAN_POINT('Ctrl Pts',(-42.604754990877,3.76794253452459,1.76532634455065));
#26028=CARTESIAN_POINT('Ctrl Pts',(-42.5927925942258,3.1908272637106,2.66620997745897));
#26029=CARTESIAN_POINT('Ctrl Pts',(-42.5863610425975,2.82679081582617,3.04947508457934));
#26030=CARTESIAN_POINT('Ctrl Pts',(-42.5727799861511,1.95827987055198,3.67109128614302));
#26031=CARTESIAN_POINT('Ctrl Pts',(-42.565745495969,1.45741866387244,3.89714054600239));
#26032=CARTESIAN_POINT('Ctrl Pts',(-42.5523803067902,0.406356146781749,
4.13958379346201));
#26033=CARTESIAN_POINT('Ctrl Pts',(-42.5466079711067,-0.132845589110581,
4.15735835990101));
#26034=CARTESIAN_POINT('Ctrl Pts',(-42.5340206983149,-1.18339757627937,
3.98696638339271));
#26035=CARTESIAN_POINT('Ctrl Pts',(-42.5273057032173,-1.68517010770252,
3.80217383029169));
#26036=CARTESIAN_POINT('Ctrl Pts',(-42.5134413562945,-2.60948276667548,
3.2418951599226));
#26037=CARTESIAN_POINT('Ctrl Pts',(-42.5064248136894,-3.01874389665988,
2.86469484965848));
#26038=CARTESIAN_POINT('Ctrl Pts',(-42.4936563305807,-3.64856784200123,
1.99434066474303));
#26039=CARTESIAN_POINT('Ctrl Pts',(-42.4880429459267,-3.87188615970388,
1.51589628663844));
#26040=CARTESIAN_POINT('Ctrl Pts',(-42.4749909574358,-4.13085568628257,
0.488794224764731));
#26041=CARTESIAN_POINT('Ctrl Pts',(-42.4680768830096,-4.15935489999998,
-0.0515006725587147));
#26042=CARTESIAN_POINT('Ctrl Pts',(-42.4542756513481,-4.00666787072579,
-1.12266854151268));
#26043=CARTESIAN_POINT('Ctrl Pts',(-42.4475277137696,-3.82304289047505,
-1.64259717952674));
#26044=CARTESIAN_POINT('Ctrl Pts',(-42.4355164062618,-3.27611316122999,
-2.56038321995924));
#26045=CARTESIAN_POINT('Ctrl Pts',(-42.4293069356349,-2.9258902950147,-2.95426188547286));
#26046=CARTESIAN_POINT('Ctrl Pts',(-42.4158363220833,-2.08128414995036,
-3.60249813982044));
#26047=CARTESIAN_POINT('Ctrl Pts',(-42.408815096909,-1.59014509167932,-3.84462953161962));
#26048=CARTESIAN_POINT('Ctrl Pts',(-42.3975278013324,-0.717744544535816,
-4.07806610689559));
#26049=CARTESIAN_POINT('Ctrl Pts',(-42.3931846180739,-0.359253305846238,
-4.12499999999999));
#26050=CARTESIAN_POINT('Ctrl Pts',(-42.3891154631359,-1.2490009027033E-14,
-4.12499999999999));
#26051=CARTESIAN_POINT('Origin',(-44.,0.,0.));
#26052=CARTESIAN_POINT('',(-42.0716154631359,2.62705756779736E-15,-4.12499999999999));
#26053=CARTESIAN_POINT('',(-42.1509904640031,1.22027311551893E-14,-4.12499999999999));
#26054=CARTESIAN_POINT('',(-44.,-5.05166804648282E-16,-4.12499999999999));
#26055=CARTESIAN_POINT('Ctrl Pts',(-42.1509904640031,3.17801340798951E-14,
-4.12499999999999));
#26056=CARTESIAN_POINT('Ctrl Pts',(-42.1560338924339,-0.445268947525859,
-4.12499999999999));
#26057=CARTESIAN_POINT('Ctrl Pts',(-42.1614864674767,-0.888322840384305,
-4.05289790512554));
#26058=CARTESIAN_POINT('Ctrl Pts',(-42.1739587071193,-1.82280109361283,
-3.73946011707928));
#26059=CARTESIAN_POINT('Ctrl Pts',(-42.1809364412098,-2.29532167022266,
-3.46953387089725));
#26060=CARTESIAN_POINT('Ctrl Pts',(-42.1941972499297,-3.09660567355616,
-2.77465727096019));
#26061=CARTESIAN_POINT('Ctrl Pts',(-42.2000095838757,-3.42229302213132,
-2.36126943593959));
#26062=CARTESIAN_POINT('Ctrl Pts',(-42.2123833088279,-3.91364098116501,
-1.41327377823633));
#26063=CARTESIAN_POINT('Ctrl Pts',(-42.2192468040062,-4.06617713874996,
-0.883245970453483));
#26064=CARTESIAN_POINT('Ctrl Pts',(-42.2330739520629,-4.15483875880001,
0.192179200922925));
#26065=CARTESIAN_POINT('Ctrl Pts',(-42.2399010836908,-4.09529222310576,
0.726776732738759));
#26066=CARTESIAN_POINT('Ctrl Pts',(-42.2527296541061,-3.77776018814276,
1.73849717190354));
#26067=CARTESIAN_POINT('Ctrl Pts',(-42.2583228562987,-3.52474092831486,
2.2068180825215));
#26068=CARTESIAN_POINT('Ctrl Pts',(-42.2713900111586,-2.84321758139603,
3.03837146446667));
#26069=CARTESIAN_POINT('Ctrl Pts',(-42.2784280439159,-2.41513573679348,
3.38861360283517));
#26070=CARTESIAN_POINT('Ctrl Pts',(-42.2921781579391,-1.46558462246781,
3.89169829027523));
#26071=CARTESIAN_POINT('Ctrl Pts',(-42.298766051037,-0.957005192665014,
4.04690043324374));
#26072=CARTESIAN_POINT('Ctrl Pts',(-42.3111128479386,0.10769051217861,4.15928298587356));
#26073=CARTESIAN_POINT('Ctrl Pts',(-42.3172493225262,0.654372363406386,
4.10889740066407));
#26074=CARTESIAN_POINT('Ctrl Pts',(-42.3308858004633,1.69395759783205,3.79982275752029));
#26075=CARTESIAN_POINT('Ctrl Pts',(-42.3378908816764,2.17704339310721,3.5452259825536));
#26076=CARTESIAN_POINT('Ctrl Pts',(-42.3512702445266,3.00254148378252,2.87620430103972));
#26077=CARTESIAN_POINT('Ctrl Pts',(-42.3572809620275,3.34187630402635,2.47379412796274));
#26078=CARTESIAN_POINT('Ctrl Pts',(-42.3694530362566,3.86447672600527,1.54261864147942));
#26079=CARTESIAN_POINT('Ctrl Pts',(-42.3762546983053,4.03453426683527,1.01802569478419));
#26080=CARTESIAN_POINT('Ctrl Pts',(-42.3900733439701,4.15913036951586,-0.055481427931184));
#26081=CARTESIAN_POINT('Ctrl Pts',(-42.3969519954047,4.1169424906266,-0.593491341014654));
#26082=CARTESIAN_POINT('Ctrl Pts',(-42.4099073092143,3.83225847614284,-1.61395072119891));
#26083=CARTESIAN_POINT('Ctrl Pts',(-42.4154887279345,3.59605813030624,-2.08791930193469));
#26084=CARTESIAN_POINT('Ctrl Pts',(-42.4283891662422,2.943644797198,-2.94153392581003));
#26085=CARTESIAN_POINT('Ctrl Pts',(-42.4354180316776,2.52599193930369,-3.30711739042688));
#26086=CARTESIAN_POINT('Ctrl Pts',(-42.4492381287215,1.59028508813065,-3.84265224811036));
#26087=CARTESIAN_POINT('Ctrl Pts',(-42.4559002985671,1.08534260792206,-4.01460106544558));
#26088=CARTESIAN_POINT('Ctrl Pts',(-42.4642898645937,0.375169285999567,
-4.1122171789071));
#26089=CARTESIAN_POINT('Ctrl Pts',(-42.4663667894089,0.187492766960302,
-4.12499999999999));
#26090=CARTESIAN_POINT('Ctrl Pts',(-42.4684904640031,2.09704502270805E-14,
-4.12499999999999));
#26091=CARTESIAN_POINT('Ctrl Pts',(-42.3891154631359,-1.1763057222536E-14,
-4.12499999999999));
#26092=CARTESIAN_POINT('Ctrl Pts',(-42.3871013770239,0.177817533376489,
-4.12499999999999));
#26093=CARTESIAN_POINT('Ctrl Pts',(-42.385134084848,0.355821541514001,-4.11350241751702));
#26094=CARTESIAN_POINT('Ctrl Pts',(-42.3768891234525,1.05664824774418,-4.02220037883837));
#26095=CARTESIAN_POINT('Ctrl Pts',(-42.3702430602757,1.56245378510728,-3.85400208227205));
#26096=CARTESIAN_POINT('Ctrl Pts',(-42.3564374347192,2.50136014959374,-3.32571631658645));
#26097=CARTESIAN_POINT('Ctrl Pts',(-42.3494058416175,2.92139877157236,-2.96354962449462));
#26098=CARTESIAN_POINT('Ctrl Pts',(-42.336467544458,3.58036382231714,-2.11485078686789));
#26099=CARTESIAN_POINT('Ctrl Pts',(-42.330888673688,3.8203268224177,-1.6421639770986));
#26100=CARTESIAN_POINT('Ctrl Pts',(-42.3179616762174,4.11243104906792,-0.623654159522199));
#26101=CARTESIAN_POINT('Ctrl Pts',(-42.311094051705,4.15855387560653,-0.086366937965185));
#26102=CARTESIAN_POINT('Ctrl Pts',(-42.2972721364892,4.04207283103092,0.987678594684015));
#26103=CARTESIAN_POINT('Ctrl Pts',(-42.2904558347728,3.87595592604241,1.51355104947175));
#26104=CARTESIAN_POINT('Ctrl Pts',(-42.2782378352712,3.36039808868393,2.44855465216588));
#26105=CARTESIAN_POINT('Ctrl Pts',(-42.2722773522877,3.0241706380018,2.8534361254441));
#26106=CARTESIAN_POINT('Ctrl Pts',(-42.2589245903854,2.2041621677276,3.52836536376145));
#26107=CARTESIAN_POINT('Ctrl Pts',(-42.2519250414944,1.72343714359835,3.78648349673181));
#26108=CARTESIAN_POINT('Ctrl Pts',(-42.2382557634832,0.685447014643934,
4.10400433986152));
#26109=CARTESIAN_POINT('Ctrl Pts',(-42.2320604506867,0.137790688399652,
4.15856861996258));
#26110=CARTESIAN_POINT('Ctrl Pts',(-42.2197444246986,-0.928622284584786,
4.05346076698241));
#26111=CARTESIAN_POINT('Ctrl Pts',(-42.2131737298568,-1.43792916326425,
3.90195270202446));
#26112=CARTESIAN_POINT('Ctrl Pts',(-42.1994409049684,-2.39038155574977,
3.40605431517219));
#26113=CARTESIAN_POINT('Ctrl Pts',(-42.1924018892718,-2.82068666982909,
3.05922555831872));
#26114=CARTESIAN_POINT('Ctrl Pts',(-42.1792987632596,-3.50858330700064,
2.23258010552681));
#26115=CARTESIAN_POINT('Ctrl Pts',(-42.1736950335671,-3.76532151402767,
1.76548129801672));
#26116=CARTESIAN_POINT('Ctrl Pts',(-42.1608945290857,-4.09000552243583,
0.755700256903659));
#26117=CARTESIAN_POINT('Ctrl Pts',(-42.1540795347079,-4.15330895456272,
0.221918240168212));
#26118=CARTESIAN_POINT('Ctrl Pts',(-42.1402525799222,-4.07247098359919,
-0.853765063861801));
#26119=CARTESIAN_POINT('Ctrl Pts',(-42.1333766474844,-3.92377409583911,
-1.38489705152091));
#26120=CARTESIAN_POINT('Ctrl Pts',(-42.120959597757,-3.43925693052631,-2.33651059002945));
#26121=CARTESIAN_POINT('Ctrl Pts',(-42.1151822829565,-3.11650566204604,
-2.75230237631966));
#26122=CARTESIAN_POINT('Ctrl Pts',(-42.1019475386014,-2.32046290297941,
-3.45270850167069));
#26123=CARTESIAN_POINT('Ctrl Pts',(-42.0949767153039,-1.85027981688563,
-3.72588343508057));
#26124=CARTESIAN_POINT('Ctrl Pts',(-42.0823642419539,-0.908829747591119,
-4.04949405600422));
#26125=CARTESIAN_POINT('Ctrl Pts',(-42.0767765678079,-0.455658224733047,
-4.12499999999999));
#26126=CARTESIAN_POINT('Ctrl Pts',(-42.0716154631359,1.06858966120171E-14,
-4.12499999999999));
#26127=CARTESIAN_POINT('Origin',(-44.,0.,0.));
#26128=CARTESIAN_POINT('',(-41.7541154631073,1.26320085361692E-9,-4.12499999999999));
#26129=CARTESIAN_POINT('',(-41.8334904640031,-3.97348897155563E-14,-4.12499999999999));
#26130=CARTESIAN_POINT('',(-44.,-5.05166804648282E-16,-4.12499999999999));
#26131=CARTESIAN_POINT('Ctrl Pts',(-41.8334904640031,-7.8687056870308E-14,
-4.12499999999999));
#26132=CARTESIAN_POINT('Ctrl Pts',(-41.8395591778476,-0.535788276456958,
-4.12499999999998));
#26133=CARTESIAN_POINT('Ctrl Pts',(-41.8461999805038,-1.06657900485524,
-4.02060928412677));
#26134=CARTESIAN_POINT('Ctrl Pts',(-41.859877854739,-2.0583164902902,-3.61467252212009));
#26135=CARTESIAN_POINT('Ctrl Pts',(-41.866783485758,-2.50979563480639,-3.31714535243961));
#26136=CARTESIAN_POINT('Ctrl Pts',(-41.8798115324135,-3.26517178664293,
-2.57457729607812));
#26137=CARTESIAN_POINT('Ctrl Pts',(-41.8854135929961,-3.56528624481668,
-2.13974936930175));
#26138=CARTESIAN_POINT('Ctrl Pts',(-41.8982151485474,-3.9977239376065,-1.15632561685152));
#26139=CARTESIAN_POINT('Ctrl Pts',(-41.9052351811761,-4.11621596943027,
-0.612898998358878));
#26140=CARTESIAN_POINT('Ctrl Pts',(-41.9190893201413,-4.13252385019637,
0.467158119454977));
#26141=CARTESIAN_POINT('Ctrl Pts',(-41.9257915479999,-4.03850430093581,
0.993216947518014));
#26142=CARTESIAN_POINT('Ctrl Pts',(-41.9383534078591,-3.65461681773415,
1.98645107418684));
#26143=CARTESIAN_POINT('Ctrl Pts',(-41.9441558529599,-3.36625086906328,
2.44347504257847));
#26144=CARTESIAN_POINT('Ctrl Pts',(-41.9575509421477,-2.62518032277939,
3.22797313494093));
#26145=CARTESIAN_POINT('Ctrl Pts',(-41.964583513613,-2.17720829183821,3.54558094845617));
#26146=CARTESIAN_POINT('Ctrl Pts',(-41.978144146734,-1.2024384117774,3.9804339500067));
#26147=CARTESIAN_POINT('Ctrl Pts',(-41.9845581524079,-0.688055081347689,
4.10076853475202));
#26148=CARTESIAN_POINT('Ctrl Pts',(-41.9964750015311,0.380622650465051,
4.14353186971007));
#26149=CARTESIAN_POINT('Ctrl Pts',(-42.0031297052446,0.925132281569847,
4.05683177438524));
#26150=CARTESIAN_POINT('Ctrl Pts',(-42.0169046083988,1.94061878465416,3.67944938583939));
#26151=CARTESIAN_POINT('Ctrl Pts',(-42.0238499588673,2.40290186475778,3.3956463027297));
#26152=CARTESIAN_POINT('Ctrl Pts',(-42.0369970178963,3.18150757612987,2.67700544892334));
#26153=CARTESIAN_POINT('Ctrl Pts',(-42.0426782231437,3.49452654137339,2.25313763786531));
#26154=CARTESIAN_POINT('Ctrl Pts',(-42.0552385214842,3.95614015023096,1.28955085881659));
#26155=CARTESIAN_POINT('Ctrl Pts',(-42.0621533383092,4.09194949567983,0.754935835501052));
#26156=CARTESIAN_POINT('Ctrl Pts',(-42.0759743533171,4.14665431899328,-0.321196753876167));
#26157=CARTESIAN_POINT('Ctrl Pts',(-42.0827464244384,4.07085950337766,-0.852066953666844));
#26158=CARTESIAN_POINT('Ctrl Pts',(-42.0954519040899,3.72226707730659,-1.85527093258268));
#26159=CARTESIAN_POINT('Ctrl Pts',(-42.1011117951717,3.45294113962082,-2.31829704960152));
#26160=CARTESIAN_POINT('Ctrl Pts',(-42.1143341632307,2.74365561441163,-3.12825399866998));
#26161=CARTESIAN_POINT('Ctrl Pts',(-42.1213737511663,2.30605190529893,-3.46348674000982));
#26162=CARTESIAN_POINT('Ctrl Pts',(-42.135043338992,1.34421224947164,-3.93505999849845));
#26163=CARTESIAN_POINT('Ctrl Pts',(-42.1415538466163,0.832648315696499,
-4.07410229519049));
#26164=CARTESIAN_POINT('Ctrl Pts',(-42.1486923346059,0.205876506656136,
-4.12115129696902));
#26165=CARTESIAN_POINT('Ctrl Pts',(-42.1498251835423,0.102879065588091,
-4.12499999999999));
#26166=CARTESIAN_POINT('Ctrl Pts',(-42.1509904640031,3.22433800653442E-14,
-4.12499999999999));
#26167=CARTESIAN_POINT('Ctrl Pts',(-42.0716154631359,1.00826204764594E-14,
-4.12499999999999));
#26168=CARTESIAN_POINT('Ctrl Pts',(-42.0706071354656,0.0890221813736162,
-4.12499999999999));
#26169=CARTESIAN_POINT('Ctrl Pts',(-42.0696256589146,0.17813940412384,-4.12211823705744));
#26170=CARTESIAN_POINT('Ctrl Pts',(-42.0626886542998,0.7909332714484,-4.08233867750673));
#26171=CARTESIAN_POINT('Ctrl Pts',(-42.0562052748367,1.30338169855081,-3.94870250210379));
#26172=CARTESIAN_POINT('Ctrl Pts',(-42.0425654464095,2.26910007257139,-3.48771418943761));
#26173=CARTESIAN_POINT('Ctrl Pts',(-42.0355269191161,2.7097718068153,-3.15754733837929));
#26174=CARTESIAN_POINT('Ctrl Pts',(-42.022253867818,3.42827956248434,-2.35489338257773));
#26175=CARTESIAN_POINT('Ctrl Pts',(-42.0165598775598,3.70308685011076,-1.89361285033071));
#26176=CARTESIAN_POINT('Ctrl Pts',(-42.003895768798,4.06194662621669,-0.89327726827948));
#26177=CARTESIAN_POINT('Ctrl Pts',(-41.9971432275796,4.14307116392663,-0.363744288221829));
#26178=CARTESIAN_POINT('Ctrl Pts',(-41.9833272568024,4.09957329739581,0.712386205342942));
#26179=CARTESIAN_POINT('Ctrl Pts',(-41.9763970206415,3.96932046878808,1.24839797888657));
#26180=CARTESIAN_POINT('Ctrl Pts',(-41.9637759771424,3.51757530187574,2.21706751039052));
#26181=CARTESIAN_POINT('Ctrl Pts',(-41.9581262385893,3.20869952870754,2.64442330263496));
#26182=CARTESIAN_POINT('Ctrl Pts',(-41.9450170702117,2.43754139377463,3.37077950978567));
#26183=CARTESIAN_POINT('Ctrl Pts',(-41.938083744251,1.97868840678086,3.65903706703988));
#26184=CARTESIAN_POINT('Ctrl Pts',(-41.9242975634932,0.967763055249048,
4.04687030811766));
#26185=CARTESIAN_POINT('Ctrl Pts',(-41.9175842347531,0.424208048029082,
4.13929740023204));
#26186=CARTESIAN_POINT('Ctrl Pts',(-41.9056710388727,-0.644320389458257,
4.10779781125427));
#26187=CARTESIAN_POINT('Ctrl Pts',(-41.8993231337814,-1.15943347937385,
3.99310500027776));
#26188=CARTESIAN_POINT('Ctrl Pts',(-41.8857982796435,-2.13785287067713,
3.56935563619536));
#26189=CARTESIAN_POINT('Ctrl Pts',(-41.8787696603756,-2.58881238302563,
3.25711017274507));
#26190=CARTESIAN_POINT('Ctrl Pts',(-41.8653240099461,-3.33939203076905,
2.48039210939859));
#26191=CARTESIAN_POINT('Ctrl Pts',(-41.8594652417615,-3.63353898381416,
2.02516037260728));
#26192=CARTESIAN_POINT('Ctrl Pts',(-41.8469469235392,-4.02793962295403,
1.03495537794674));
#26193=CARTESIAN_POINT('Ctrl Pts',(-41.8402669562126,-4.12733191964218,
0.510445256955648));
#26194=CARTESIAN_POINT('Ctrl Pts',(-41.826431375729,-4.12249034620183,-0.56856470653867));
#26195=CARTESIAN_POINT('Ctrl Pts',(-41.8194060573837,-4.01002352305216,
-1.11261401728585));
#26196=CARTESIAN_POINT('Ctrl Pts',(-41.8065486818142,-3.58848388940988,
-2.10077231492132));
#26197=CARTESIAN_POINT('Ctrl Pts',(-41.8009607349585,-3.29273067922381,
-2.53936740460541));
#26198=CARTESIAN_POINT('Ctrl Pts',(-41.7879735316739,-2.54522144101839,
-3.28994919264909));
#26199=CARTESIAN_POINT('Ctrl Pts',(-41.7810828091145,-2.0974692024319,-3.59201019840101));
#26200=CARTESIAN_POINT('Ctrl Pts',(-41.7672688239022,-1.10147983510762,
-4.01255069242754));
#26201=CARTESIAN_POINT('Ctrl Pts',(-41.7604842356396,-0.561200380517341,
-4.12297039185286));
#26202=CARTESIAN_POINT('Ctrl Pts',(-41.7542297015537,-0.0100808504658389,
-4.12499076228453));
#26203=CARTESIAN_POINT('Ctrl Pts',(-41.7541725520838,-0.00504020946799272,
-4.12500000000308));
#26204=CARTESIAN_POINT('Ctrl Pts',(-41.7541154631073,2.52640221240065E-9,
-4.12499999999999));
#26205=CARTESIAN_POINT('Origin',(-44.,0.,0.));
#26206=CARTESIAN_POINT('',(-41.4366154631359,1.78571668194861E-15,-4.12499999999999));
#26207=CARTESIAN_POINT('',(-41.5159904640031,-7.9070507400718E-15,-4.12499999999999));
#26208=CARTESIAN_POINT('',(-44.,-5.05166804648282E-16,-4.12499999999999));
#26209=CARTESIAN_POINT('Ctrl Pts',(-41.5159904640031,-1.18330754202892E-14,
-4.12499999999999));
#26210=CARTESIAN_POINT('Ctrl Pts',(-41.5169064666755,-0.0808710882830204,
-4.12499999999999));
#26211=CARTESIAN_POINT('Ctrl Pts',(-41.5178376612464,-0.161818913602757,
-4.12262180362065));
#26212=CARTESIAN_POINT('Ctrl Pts',(-41.525152401119,-0.787988831146203,
-4.08571028062563));
#26213=CARTESIAN_POINT('Ctrl Pts',(-41.5320387340023,-1.32145965265631,
-3.94559136003377));
#26214=CARTESIAN_POINT('Ctrl Pts',(-41.5458649386386,-2.29023705263989,
-3.47184364151419));
#26215=CARTESIAN_POINT('Ctrl Pts',(-41.5526692345746,-2.71861702121608,
-3.14769928392844));
#26216=CARTESIAN_POINT('Ctrl Pts',(-41.5654454686437,-3.42624217444751,
-2.35713653314498));
#26217=CARTESIAN_POINT('Ctrl Pts',(-41.5710605547243,-3.69987605959061,
-1.89898547979264));
#26218=CARTESIAN_POINT('Ctrl Pts',(-41.5841945105728,-4.06539635765999,
-0.887297606981464));
#26219=CARTESIAN_POINT('Ctrl Pts',(-41.5912340750953,-4.14709738387759,
-0.341062725244499));
#26220=CARTESIAN_POINT('Ctrl Pts',(-41.6049514347675,-4.0937195899075,0.730759047958374));
#26221=CARTESIAN_POINT('Ctrl Pts',(-41.6115070426618,-3.96720999099781,
1.24651605651722));
#26222=CARTESIAN_POINT('Ctrl Pts',(-41.6237963514478,-3.51884470746436,
2.22074273986629));
#26223=CARTESIAN_POINT('Ctrl Pts',(-41.6300448827958,-3.19419463151977,
2.66666423168129));
#26224=CARTESIAN_POINT('Ctrl Pts',(-41.6437422794425,-2.39458481918784,
3.40195027359171));
#26225=CARTESIAN_POINT('Ctrl Pts',(-41.6507367100721,-1.92909112707186,
3.6859069333138));
#26226=CARTESIAN_POINT('Ctrl Pts',(-41.6640662626243,-0.932543250535931,
4.05191519173872));
#26227=CARTESIAN_POINT('Ctrl Pts',(-41.6699856615776,-0.413272813762911,
4.13725146996676));
#26228=CARTESIAN_POINT('Ctrl Pts',(-41.6822434024603,0.654048294593352,
4.109270905025));
#26229=CARTESIAN_POINT('Ctrl Pts',(-41.6890721110328,1.19175078806432,3.98667875081201));
#26230=CARTESIAN_POINT('Ctrl Pts',(-41.702896228521,2.17697664219642,3.54421263294516));
#26231=CARTESIAN_POINT('Ctrl Pts',(-41.7097539781292,2.61694886463819,3.23299449297784));
#26232=CARTESIAN_POINT('Ctrl Pts',(-41.7226562142323,3.34824990507222,2.46603777649558));
#26233=CARTESIAN_POINT('Ctrl Pts',(-41.7282353282386,3.63502138046449,2.01958879815716));
#26234=CARTESIAN_POINT('Ctrl Pts',(-41.7412064410462,4.03395292401031,1.02176947315805));
#26235=CARTESIAN_POINT('Ctrl Pts',(-41.7482400967005,4.13395732363673,0.47663465262452));
#26236=CARTESIAN_POINT('Ctrl Pts',(-41.7620325149337,4.11514927403033,-0.599834506646873));
#26237=CARTESIAN_POINT('Ctrl Pts',(-41.7686642617806,4.00470855990209,-1.12096923636333));
#26238=CARTESIAN_POINT('Ctrl Pts',(-41.7810912029171,3.58851334733966,-2.10480787679789));
#26239=CARTESIAN_POINT('Ctrl Pts',(-41.7870870932464,3.28221629689906,-2.55630723943552));
#26240=CARTESIAN_POINT('Ctrl Pts',(-41.8006360790771,2.51187359056085,-3.31659875348705));
#26241=CARTESIAN_POINT('Ctrl Pts',(-41.8076537182903,2.05487827683795,-3.61756971572469));
#26242=CARTESIAN_POINT('Ctrl Pts',(-41.8211016757378,1.06904147596912,-4.01813700315628));
#26243=CARTESIAN_POINT('Ctrl Pts',(-41.8272578864661,0.552347994909614,
-4.12106421930381));
#26244=CARTESIAN_POINT('Ctrl Pts',(-41.8332625189997,0.0201441818758197,
-4.12496311665681));
#26245=CARTESIAN_POINT('Ctrl Pts',(-41.8333763904363,0.0100712080537732,
-4.12499999999999));
#26246=CARTESIAN_POINT('Ctrl Pts',(-41.8334904640031,-7.85254087802035E-14,
-4.12499999999999));
#26247=CARTESIAN_POINT('Ctrl Pts',(-41.7541154631073,2.52640221240065E-9,
-4.12499999999999));
#26248=CARTESIAN_POINT('Ctrl Pts',(-41.7482626432124,0.516727659373442,
-4.12499999968352));
#26249=CARTESIAN_POINT('Ctrl Pts',(-41.7422293800106,1.02893702726848,-4.02790594356507));
#26250=CARTESIAN_POINT('Ctrl Pts',(-41.7288835687061,2.01365979063146,-3.64058183567956));
#26251=CARTESIAN_POINT('Ctrl Pts',(-41.7218726813988,2.47352462425983,-3.3451962913757));
#26252=CARTESIAN_POINT('Ctrl Pts',(-41.7082739814623,3.25354692617725,-2.59308227027601));
#26253=CARTESIAN_POINT('Ctrl Pts',(-41.7022010727125,3.56586474073121,-2.1434188269279));
#26254=CARTESIAN_POINT('Ctrl Pts',(-41.6898193365417,3.99271145407791,-1.16273422749369));
#26255=CARTESIAN_POINT('Ctrl Pts',(-41.6832121542179,4.10850532121644,-0.64332860102408));
#26256=CARTESIAN_POINT('Ctrl Pts',(-41.6694431045306,4.13880671511246,0.431719161751283));
#26257=CARTESIAN_POINT('Ctrl Pts',(-41.6624066525318,4.044876135757,0.977284200391839));
#26258=CARTESIAN_POINT('Ctrl Pts',(-41.6493809475519,3.65700162885682,1.97974784987871));
#26259=CARTESIAN_POINT('Ctrl Pts',(-41.6437962991127,3.37459401737114,2.43005714560394));
#26260=CARTESIAN_POINT('Ctrl Pts',(-41.6309357144839,2.6511648782504,3.20490279380071));
#26261=CARTESIAN_POINT('Ctrl Pts',(-41.6240950523528,2.21501810087195,3.52047828305974));
#26262=CARTESIAN_POINT('Ctrl Pts',(-41.6102685834166,1.23516775348485,3.97344470167659));
#26263=CARTESIAN_POINT('Ctrl Pts',(-41.6034198208226,0.69881157589226,4.10189875001512));
#26264=CARTESIAN_POINT('Ctrl Pts',(-41.5910960941911,-0.368151649154125,
4.14150890791189));
#26265=CARTESIAN_POINT('Ctrl Pts',(-41.5852399688694,-0.888308013753419,
4.06184052114298));
#26266=CARTESIAN_POINT('Ctrl Pts',(-41.5719493419555,-1.88821115154311,
3.70692788444243));
#26267=CARTESIAN_POINT('Ctrl Pts',(-41.5649640886082,-2.35630439073406,
3.42848137615101));
#26268=CARTESIAN_POINT('Ctrl Pts',(-41.5512205553717,-3.16525635115029,
2.70135906194979));
#26269=CARTESIAN_POINT('Ctrl Pts',(-41.5448789620358,-3.49586139456939,
2.25723915262381));
#26270=CARTESIAN_POINT('Ctrl Pts',(-41.5326342043063,-3.9544771530286,1.28612950930069));
#26271=CARTESIAN_POINT('Ctrl Pts',(-41.5261040609182,-4.08604265353204,
0.772182183164868));
#26272=CARTESIAN_POINT('Ctrl Pts',(-41.5124134013752,-4.15034109753943,
-0.297938330209873));
#26273=CARTESIAN_POINT('Ctrl Pts',(-41.5053735373433,-4.07444377836835,
-0.844399243679091));
#26274=CARTESIAN_POINT('Ctrl Pts',(-41.4921889978187,-3.71957997578257,
-1.86040478998788));
#26275=CARTESIAN_POINT('Ctrl Pts',(-41.4865505274689,-3.45010848821036,
-2.32231169383177));
#26276=CARTESIAN_POINT('Ctrl Pts',(-41.4738145603255,-2.74996538392358,
-3.1202600661284));
#26277=CARTESIAN_POINT('Ctrl Pts',(-41.4670284180359,-2.32530046045201,
-3.44837711027349));
#26278=CARTESIAN_POINT('Ctrl Pts',(-41.4532046264246,-1.36189166545342,
-3.93182103888445));
#26279=CARTESIAN_POINT('Ctrl Pts',(-41.4463017518192,-0.829869995784418,
-4.07741206503004));
#26280=CARTESIAN_POINT('Ctrl Pts',(-41.4387871633191,-0.189989831523175,
-4.12172195295433));
#26281=CARTESIAN_POINT('Ctrl Pts',(-41.4376908908779,-0.0949462424977904,
-4.12499999999999));
#26282=CARTESIAN_POINT('Ctrl Pts',(-41.4366154631359,1.00826204764594E-14,
-4.12499999999999));
#26283=CARTESIAN_POINT('Origin',(-44.,0.,0.));
#26284=CARTESIAN_POINT('',(-41.1191154638315,-3.0705135232325E-8,-4.12499999999999));
#26285=CARTESIAN_POINT('',(-41.1984904632914,3.14162372061423E-8,-4.12499999999999));
#26286=CARTESIAN_POINT('',(-44.,-5.05166804648282E-16,-4.12499999999999));
#26287=CARTESIAN_POINT('Ctrl Pts',(-41.1984904636472,3.14203072240837E-8,
-4.12499999999999));
#26288=CARTESIAN_POINT('Ctrl Pts',(-41.2004042872906,-0.168965634416243,
-4.12500000128701));
#26289=CARTESIAN_POINT('Ctrl Pts',(-41.2023825656739,-0.338101978249229,
-4.114618703125));
#26290=CARTESIAN_POINT('Ctrl Pts',(-41.2110030427661,-1.05220486136019,
-4.02627570612251));
#26291=CARTESIAN_POINT('Ctrl Pts',(-41.2180295293847,-1.5789854227773,-3.85030260331271));
#26292=CARTESIAN_POINT('Ctrl Pts',(-41.2318603414182,-2.51421818099586,
-3.31270156035402));
#26293=CARTESIAN_POINT('Ctrl Pts',(-41.2385347595153,-2.91777039863962,
-2.96342838054045));
#26294=CARTESIAN_POINT('Ctrl Pts',(-41.2510423657805,-3.57618020949202,
-2.12490896476215));
#26295=CARTESIAN_POINT('Ctrl Pts',(-41.2569158946691,-3.82225694858102,
-1.6415416877236));
#26296=CARTESIAN_POINT('Ctrl Pts',(-41.27037385398,-4.11679795812124,-0.602102805487428));
#26297=CARTESIAN_POINT('Ctrl Pts',(-41.2774013732852,-4.16022530825056,
-0.0554709077489143));
#26298=CARTESIAN_POINT('Ctrl Pts',(-41.2909172897172,-4.0351898209026,1.00314057981436));
#26299=CARTESIAN_POINT('Ctrl Pts',(-41.2972413020317,-3.87567202277939,
1.50605216667389));
#26300=CARTESIAN_POINT('Ctrl Pts',(-41.3091708039741,-3.36630412025233,
2.44575960254218));
#26301=CARTESIAN_POINT('Ctrl Pts',(-41.3158899774543,-3.01337777792877,
2.86937050451361));
#26302=CARTESIAN_POINT('Ctrl Pts',(-41.3296788863341,-2.17037455234931,
3.54867430021675));
#26303=CARTESIAN_POINT('Ctrl Pts',(-41.3366091344405,-1.69078914481731,
3.80063805434704));
#26304=CARTESIAN_POINT('Ctrl Pts',(-41.3497088930555,-0.675441298380965,
4.10275667587154));
#26305=CARTESIAN_POINT('Ctrl Pts',(-41.3553517360618,-0.150664019239523,
4.15525340870424));
#26306=CARTESIAN_POINT('Ctrl Pts',(-41.3680534433334,0.919496695149706,
4.05889558137054));
#26307=CARTESIAN_POINT('Ctrl Pts',(-41.3750621471651,1.45359422294924,3.89963640912485));
#26308=CARTESIAN_POINT('Ctrl Pts',(-41.3889453632281,2.4086002008445,3.39052202916359));
#26309=CARTESIAN_POINT('Ctrl Pts',(-41.3956852034788,2.824189305568,3.05302401047762));
#26310=CARTESIAN_POINT('Ctrl Pts',(-41.408322946054,3.50624077004482,2.23735977487124));
#26311=CARTESIAN_POINT('Ctrl Pts',(-41.4140416444253,3.76561366420139,1.76625562075626));
#26312=CARTESIAN_POINT('Ctrl Pts',(-41.4273466055861,4.09451215588275,0.739950425480524));
#26313=CARTESIAN_POINT('Ctrl Pts',(-41.4343840485107,4.15634843276931,0.193187336624593));
#26314=CARTESIAN_POINT('Ctrl Pts',(-41.4480042183726,4.06567365410874,-0.872356044391565));
#26315=CARTESIAN_POINT('Ctrl Pts',(-41.4544700226359,3.92193758677376,-1.38170990687377));
#26316=CARTESIAN_POINT('Ctrl Pts',(-41.4665219163392,3.44167337160256,-2.33853208454178));
#26317=CARTESIAN_POINT('Ctrl Pts',(-41.4730195565733,3.10219191222297,-2.7731339278448));
#26318=CARTESIAN_POINT('Ctrl Pts',(-41.4867718677304,2.27962297532667,-3.47975578357437));
#26319=CARTESIAN_POINT('Ctrl Pts',(-41.4937364829231,1.80656753398599,-3.74722517231711));
#26320=CARTESIAN_POINT('Ctrl Pts',(-41.5059384302564,0.877091854307792,
-4.05469718261492));
#26321=CARTESIAN_POINT('Ctrl Pts',(-41.5110103044948,0.439683126898675,
-4.12499999999999));
#26322=CARTESIAN_POINT('Ctrl Pts',(-41.5159904640031,-1.18330754202892E-14,
-4.12499999999999));
#26323=CARTESIAN_POINT('Ctrl Pts',(-41.4366154631359,1.00826204764594E-14,
-4.12499999999999));
#26324=CARTESIAN_POINT('Ctrl Pts',(-41.4317940371804,0.425669024604756,
-4.12499999999999));
#26325=CARTESIAN_POINT('Ctrl Pts',(-41.4268949318863,0.849375791545828,
-4.05910724870507));
#26326=CARTESIAN_POINT('Ctrl Pts',(-41.4149033936746,1.76813330683894,-3.76543441969213));
#26327=CARTESIAN_POINT('Ctrl Pts',(-41.4079495348907,2.24342129297016,-3.50312015033128));
#26328=CARTESIAN_POINT('Ctrl Pts',(-41.3941837491158,3.07288942831861,-2.80555716233585));
#26329=CARTESIAN_POINT('Ctrl Pts',(-41.3875981767775,3.41688030312777,-2.37459638194406));
#26330=CARTESIAN_POINT('Ctrl Pts',(-41.375623100298,3.90691815915836,-1.42342466553835));
#26331=CARTESIAN_POINT('Ctrl Pts',(-41.3691866776663,4.05595320297728,-0.916177533959273));
#26332=CARTESIAN_POINT('Ctrl Pts',(-41.3555999968818,4.15815176059325,0.14715610915311));
#26333=CARTESIAN_POINT('Ctrl Pts',(-41.3485650216949,4.10247827203129,0.693941923109606));
#26334=CARTESIAN_POINT('Ctrl Pts',(-41.3352082450052,3.785032576777,1.72468868416642));
#26335=CARTESIAN_POINT('Ctrl Pts',(-41.3294439600945,3.53009840798865,2.19986935707565));
#26336=CARTESIAN_POINT('Ctrl Pts',(-41.3168495808063,2.85596491216151,3.02322492890188));
#26337=CARTESIAN_POINT('Ctrl Pts',(-41.3101310458571,2.44438625515306,3.36472789343333));
#26338=CARTESIAN_POINT('Ctrl Pts',(-41.2962639281764,1.49593664801328,3.88349997977635));
#26339=CARTESIAN_POINT('Ctrl Pts',(-41.2892484157969,0.964243672942856,
4.04841197387696));
#26340=CARTESIAN_POINT('Ctrl Pts',(-41.2764892467617,-0.104631011406712,
4.15672963094904));
#26341=CARTESIAN_POINT('Ctrl Pts',(-41.2708722798639,-0.630461211216935,
4.1099719745518));
#26342=CARTESIAN_POINT('Ctrl Pts',(-41.2578135827526,-1.64893728802458,
3.81889984176855));
#26343=CARTESIAN_POINT('Ctrl Pts',(-41.2508971823998,-2.13074152766268,
3.57252400847945));
#26344=CARTESIAN_POINT('Ctrl Pts',(-41.2370975291885,-2.98090443188783,
2.90309756948463));
#26345=CARTESIAN_POINT('Ctrl Pts',(-41.230353540608,-3.33859389179644,2.48345887136472));
#26346=CARTESIAN_POINT('Ctrl Pts',(-41.2183536245615,-3.85828119023053,
1.54990778949892));
#26347=CARTESIAN_POINT('Ctrl Pts',(-41.2121287394241,-4.02337456439361,
1.0492964816937));
#26348=CARTESIAN_POINT('Ctrl Pts',(-41.1986517713558,-4.1605053726292,-0.00669940082423867));
#26349=CARTESIAN_POINT('Ctrl Pts',(-41.1916295921606,-4.12357675364772,
-0.553141709230854));
#26350=CARTESIAN_POINT('Ctrl Pts',(-41.1781189185054,-3.84127647443778,
-1.59711978036542));
#26351=CARTESIAN_POINT('Ctrl Pts',(-41.1721774070469,-3.59992621745098,
-2.08487947020022));
#26352=CARTESIAN_POINT('Ctrl Pts',(-41.1597161953658,-2.94985948018453,
-2.93138640074789));
#26353=CARTESIAN_POINT('Ctrl Pts',(-41.1530661326808,-2.55059699927362,
-3.28468334129481));
#26354=CARTESIAN_POINT('Ctrl Pts',(-41.1392568744909,-1.62247801565102,
-3.83208457025847));
#26355=CARTESIAN_POINT('Ctrl Pts',(-41.13222591755,-1.09837547570754,-4.01383656740647));
#26356=CARTESIAN_POINT('Ctrl Pts',(-41.1233819784795,-0.370064243632087,
-4.11256198139676));
#26357=CARTESIAN_POINT('Ctrl Pts',(-41.1212103068118,-0.184947372187953,
-4.12499999862313));
#26358=CARTESIAN_POINT('Ctrl Pts',(-41.1191154634838,-3.07091125445469E-8,
-4.12499999999999));
#26359=CARTESIAN_POINT('Origin',(-44.,0.,0.));
#26360=CARTESIAN_POINT('',(-40.8016154631359,1.23927878701591E-15,-4.12499999999999));
#26361=CARTESIAN_POINT('',(-40.8809904640031,1.31047873626973E-14,-4.12499999999999));
#26362=CARTESIAN_POINT('',(-44.,-5.05166804648282E-16,-4.12499999999999));
#26363=CARTESIAN_POINT('Ctrl Pts',(-40.8809904640031,3.10168557504653E-14,
-4.12499999999999));
#26364=CARTESIAN_POINT('Ctrl Pts',(-40.8839470138832,-0.26102479127236,
-4.12499999999999));
#26365=CARTESIAN_POINT('Ctrl Pts',(-40.8870529019846,-0.522060729148633,
-4.10022430546627));
#26366=CARTESIAN_POINT('Ctrl Pts',(-40.8969646800572,-1.31590810541924,
-3.94744660305077));
#26367=CARTESIAN_POINT('Ctrl Pts',(-40.9040045032918,-1.82645051981365,
-3.73871952743978));
#26368=CARTESIAN_POINT('Ctrl Pts',(-40.9176885650803,-2.71938071075019,
-3.1459258679918));
#26369=CARTESIAN_POINT('Ctrl Pts',(-40.9242125192711,-3.09770419502207,
-2.77418791269944));
#26370=CARTESIAN_POINT('Ctrl Pts',(-40.9364465459559,-3.70752266479565,
-1.88970761857416));
#26371=CARTESIAN_POINT('Ctrl Pts',(-40.9428113492738,-3.92574569379075,
-1.38030921310186));
#26372=CARTESIAN_POINT('Ctrl Pts',(-40.9565658541248,-4.14814848331695,
-0.315220576048532));
#26373=CARTESIAN_POINT('Ctrl Pts',(-40.963548778103,-4.15378670615725,0.229252499479745));
#26374=CARTESIAN_POINT('Ctrl Pts',(-40.9768299884806,-3.9584895041917,1.27201044419376));
#26375=CARTESIAN_POINT('Ctrl Pts',(-40.9826718505753,-3.76611658540577,
1.76181953416122));
#26376=CARTESIAN_POINT('Ctrl Pts',(-40.9950114172715,-3.19594937715089,
2.66454953000424));
#26377=CARTESIAN_POINT('Ctrl Pts',(-41.001864890921,-2.8154718999071,3.06382536801303));
#26378=CARTESIAN_POINT('Ctrl Pts',(-41.0156916787708,-1.93173850362775,
3.68351937831143));
#26379=CARTESIAN_POINT('Ctrl Pts',(-41.0225281091007,-1.43992902586759,
3.90211964688776));
#26380=CARTESIAN_POINT('Ctrl Pts',(-41.0353785939384,-0.406484012832493,
4.13860780742009));
#26381=CARTESIAN_POINT('Ctrl Pts',(-41.0409655408276,0.124983314558916,
4.15664324157981));
#26382=CARTESIAN_POINT('Ctrl Pts',(-41.0540043698413,1.18670756229525,3.98844181504285));
#26383=CARTESIAN_POINT('Ctrl Pts',(-41.0610413736391,1.70549307778222,3.79568590729839));
#26384=CARTESIAN_POINT('Ctrl Pts',(-41.0748045405807,2.61965908259185,3.22969609932009));
#26385=CARTESIAN_POINT('Ctrl Pts',(-41.0814056757731,3.01056525603536,2.86880732798728));
#26386=CARTESIAN_POINT('Ctrl Pts',(-41.0937764079445,3.64448434837413,2.00695463922163));
#26387=CARTESIAN_POINT('Ctrl Pts',(-41.099868960675,3.87662568440571,1.51060067487246));
#26388=CARTESIAN_POINT('Ctrl Pts',(-41.1134796197322,4.13506274571464,0.457990393297178));
#26389=CARTESIAN_POINT('Ctrl Pts',(-41.1204887333393,4.15942031041744,-0.0878717865673329));
#26390=CARTESIAN_POINT('Ctrl Pts',(-41.1338886885907,3.99891612317659,-1.13867686484691));
#26391=CARTESIAN_POINT('Ctrl Pts',(-41.13994064032,3.82295917353972,-1.63489610003659));
#26392=CARTESIAN_POINT('Ctrl Pts',(-41.1520768794015,3.28315673221665,-2.55630976250079));
#26393=CARTESIAN_POINT('Ctrl Pts',(-41.1588668964708,2.91628103728796,-2.96801834399691));
#26394=CARTESIAN_POINT('Ctrl Pts',(-41.1726824579823,2.05244569098672,-3.61790446180448));
#26395=CARTESIAN_POINT('Ctrl Pts',(-41.1795694303592,1.56648346783269,-3.85329718460974));
#26396=CARTESIAN_POINT('Ctrl Pts',(-41.190468584663,0.706031521498386,-4.07958539149015));
#26397=CARTESIAN_POINT('Ctrl Pts',(-41.1944877121763,0.353390778668214,
-4.1249999973082));
#26398=CARTESIAN_POINT('Ctrl Pts',(-41.1984904636472,3.1420303382781E-8,
-4.12499999999999));
#26399=CARTESIAN_POINT('Ctrl Pts',(-41.1191154634838,-3.07091139260437E-8,
-4.12499999999999));
#26400=CARTESIAN_POINT('Ctrl Pts',(-41.1152860126284,0.338090529834655,
-4.12500000251695));
#26401=CARTESIAN_POINT('Ctrl Pts',(-41.1114506786048,0.675611576268281,
-4.08343304902581));
#26402=CARTESIAN_POINT('Ctrl Pts',(-41.1007837261389,1.52310611262671,-3.87056625707979));
#26403=CARTESIAN_POINT('Ctrl Pts',(-41.0939133549729,2.01114439427458,-3.64093801160786));
#26404=CARTESIAN_POINT('Ctrl Pts',(-41.0800921712788,2.88194622251291,-3.00137355503281));
#26405=CARTESIAN_POINT('Ctrl Pts',(-41.0732794357799,3.25355108826573,-2.5938912779187));
#26406=CARTESIAN_POINT('Ctrl Pts',(-41.0610727172601,3.80382762960107,-1.67887193692206));
#26407=CARTESIAN_POINT('Ctrl Pts',(-41.0551001677632,3.98544290848857,-1.18489296223169));
#26408=CARTESIAN_POINT('Ctrl Pts',(-41.0417408498085,4.15801392901122,-0.13683622103637));
#26409=CARTESIAN_POINT('Ctrl Pts',(-41.0347399039998,4.14014941659439,0.408615610718514));
#26410=CARTESIAN_POINT('Ctrl Pts',(-41.0210786526762,3.89414024647464,1.46560609433591));
#26411=CARTESIAN_POINT('Ctrl Pts',(-41.0148980575338,3.66679578896948,1.96645071832313));
#26412=CARTESIAN_POINT('Ctrl Pts',(-41.0025744628787,3.04122646956046,2.83618016236111));
#26413=CARTESIAN_POINT('Ctrl Pts',(-40.9959995199361,2.65466604187339,3.20089303689757));
#26414=CARTESIAN_POINT('Ctrl Pts',(-40.9822623901042,1.74780447029673,3.77629718990782));
#26415=CARTESIAN_POINT('Ctrl Pts',(-40.9752235810873,1.23183458420386,3.97464827148568));
#26416=CARTESIAN_POINT('Ctrl Pts',(-40.9621292566798,0.171727153597128,
4.15510514463831));
#26417=CARTESIAN_POINT('Ctrl Pts',(-40.9565283722576,-0.360963948783399,
4.14295711179001));
#26418=CARTESIAN_POINT('Ctrl Pts',(-40.9437209756471,-1.39733836990323,
3.91749539509072));
#26419=CARTESIAN_POINT('Ctrl Pts',(-40.9369029772592,-1.89097413188998,
3.7045291876586));
#26420=CARTESIAN_POINT('Ctrl Pts',(-40.9230759075655,-2.78111561604286,
3.09504880154495));
#26421=CARTESIAN_POINT('Ctrl Pts',(-40.9162029883302,-3.1660382402763,2.70002618019827));
#26422=CARTESIAN_POINT('Ctrl Pts',(-40.9037965342527,-3.74629750031841,
1.80360750350104));
#26423=CARTESIAN_POINT('Ctrl Pts',(-40.8980109075797,-3.94413844250431,
1.31587350265686));
#26424=CARTESIAN_POINT('Ctrl Pts',(-40.8847697694036,-4.15087445447382,
0.27584174848787));
#26425=CARTESIAN_POINT('Ctrl Pts',(-40.8777972220417,-4.15138561118553,
-0.268036689214984));
#26426=CARTESIAN_POINT('Ctrl Pts',(-40.8639968365375,-3.94096336839514,
-1.3371223995839));
#26427=CARTESIAN_POINT('Ctrl Pts',(-40.857530323586,-3.7273776994595,-1.8508722670883));
#26428=CARTESIAN_POINT('Ctrl Pts',(-40.8453417721317,-3.12549978411905,
-2.74273570037126));
#26429=CARTESIAN_POINT('Ctrl Pts',(-40.8388442759054,-2.75134560113339,
-3.11792179483804));
#26430=CARTESIAN_POINT('Ctrl Pts',(-40.8251888704923,-1.86550885922186,
-3.71929808341301));
#26431=CARTESIAN_POINT('Ctrl Pts',(-40.8181496958091,-1.35775745373826,
-3.93316659552598));
#26432=CARTESIAN_POINT('Ctrl Pts',(-40.808029911448,-0.551601820026865,
-4.09733394871241));
#26433=CARTESIAN_POINT('Ctrl Pts',(-40.8047397042343,-0.275829738591203,
-4.12499999999999));
#26434=CARTESIAN_POINT('Ctrl Pts',(-40.8016154631359,-9.0205620750794E-15,
-4.12499999999999));
#26435=CARTESIAN_POINT('Origin',(-44.,0.,0.));
#26436=CARTESIAN_POINT('',(-40.4841154631359,8.00470034332546E-15,-4.12499999999999));
#26437=CARTESIAN_POINT('',(-40.5634904640031,-9.48131229452075E-15,-4.12499999999999));
#26438=CARTESIAN_POINT('',(-44.,-5.05166804648282E-16,-4.12499999999999));
#26439=CARTESIAN_POINT('Ctrl Pts',(-40.5634904640031,-1.4363510381088E-14,
-4.12499999999999));
#26440=CARTESIAN_POINT('Ctrl Pts',(-40.5675734140323,-0.360471232468091,
-4.12499999999999));
#26441=CARTESIAN_POINT('Ctrl Pts',(-40.571932143759,-0.720165512036405,
-4.07774730593135));
#26442=CARTESIAN_POINT('Ctrl Pts',(-40.5832363854935,-1.59349134286567,
-3.84323713483626));
#26443=CARTESIAN_POINT('Ctrl Pts',(-40.5902571703085,-2.08437704877094,
-3.60070237538558));
#26444=CARTESIAN_POINT('Ctrl Pts',(-40.6037249008704,-2.92837251785335,
-2.95179630856995));
#26445=CARTESIAN_POINT('Ctrl Pts',(-40.6099274472567,-3.27824553450907,
-2.5576465443238));
#26446=CARTESIAN_POINT('Ctrl Pts',(-40.6219439142245,-3.82440199459883,
-1.63943106145909));
#26447=CARTESIAN_POINT('Ctrl Pts',(-40.6286936343242,-4.007596999902,-1.11934837125817));
#26448=CARTESIAN_POINT('Ctrl Pts',(-40.6424955661354,-4.1593901361805,-0.048094675003366));
#26449=CARTESIAN_POINT('Ctrl Pts',(-40.6494085791874,-4.13045370680168,
0.492132702753004));
#26450=CARTESIAN_POINT('Ctrl Pts',(-40.6624575231156,-3.87066496912996,
1.51902589539787));
#26451=CARTESIAN_POINT('Ctrl Pts',(-40.6680693413401,-3.64693990695748,
1.99732679628217));
#26452=CARTESIAN_POINT('Ctrl Pts',(-40.680842044632,-3.0163991495834,2.86715464410791));
#26453=CARTESIAN_POINT('Ctrl Pts',(-40.6878590472127,-2.60686785534687,
3.24399026501724));
#26454=CARTESIAN_POINT('Ctrl Pts',(-40.7017221237258,-1.68218512502133,
3.80348981623548));
#26455=CARTESIAN_POINT('Ctrl Pts',(-40.7084355068985,-1.18030743090806,
3.98787695473004));
#26456=CARTESIAN_POINT('Ctrl Pts',(-40.7210195525044,-0.129556763979266,
4.15747624818416));
#26457=CARTESIAN_POINT('Ctrl Pts',(-40.7267955976369,0.409743228067629,
4.13926407299677));
#26458=CARTESIAN_POINT('Ctrl Pts',(-40.7401645996931,1.46066303086723,3.89591931502526));
#26459=CARTESIAN_POINT('Ctrl Pts',(-40.7471988621716,1.96129409504847,3.66947502882011));
#26460=CARTESIAN_POINT('Ctrl Pts',(-40.7607773519379,2.82923062666211,3.047204693113));
#26461=CARTESIAN_POINT('Ctrl Pts',(-40.7672066864071,3.19293317205768,2.66367975186589));
#26462=CARTESIAN_POINT('Ctrl Pts',(-40.7791633166215,3.7693195703258,1.76238278909522));
#26463=CARTESIAN_POINT('Ctrl Pts',(-40.7857705616497,3.96925798059591,1.24850966615598));
#26464=CARTESIAN_POINT('Ctrl Pts',(-40.799539335584,4.15594352225663,0.18106076295438));
#26465=CARTESIAN_POINT('Ctrl Pts',(-40.8064905315325,4.14414474838805,-0.361546430985013));
#26466=CARTESIAN_POINT('Ctrl Pts',(-40.8196567319039,3.91638435717499,-1.39646720353316));
#26467=CARTESIAN_POINT('Ctrl Pts',(-40.8253561135646,3.70839290177736,-1.88042683332904));
#26468=CARTESIAN_POINT('Ctrl Pts',(-40.8378854635978,3.10944612457397,-2.76501760465572));
#26469=CARTESIAN_POINT('Ctrl Pts',(-40.8447921762378,2.71639790136549,-3.15200766330559));
#26470=CARTESIAN_POINT('Ctrl Pts',(-40.8586151755949,1.81467031067166,-3.74234764402162));
#26471=CARTESIAN_POINT('Ctrl Pts',(-40.8653968890452,1.31781029025714,-3.94481633328329));
#26472=CARTESIAN_POINT('Ctrl Pts',(-40.8749800234564,0.533357374710669,
-4.09913783379567));
#26473=CARTESIAN_POINT('Ctrl Pts',(-40.877969800176,0.266685216526378,-4.12499999999999));
#26474=CARTESIAN_POINT('Ctrl Pts',(-40.8809904640031,3.17182435821952E-14,
-4.12499999999999));
#26475=CARTESIAN_POINT('Ctrl Pts',(-40.8016154631359,-1.28833483865871E-14,
-4.12499999999999));
#26476=CARTESIAN_POINT('Ctrl Pts',(-40.7987491667761,0.253056582631218,
-4.12499999999999));
#26477=CARTESIAN_POINT('Ctrl Pts',(-40.7959184081503,0.506160509587679,
-4.10171373271893));
#26478=CARTESIAN_POINT('Ctrl Pts',(-40.7865416494958,1.27813394217847,-3.95777939416467));
#26479=CARTESIAN_POINT('Ctrl Pts',(-40.7797789333525,1.77651344586574,-3.76053694882057));
#26480=CARTESIAN_POINT('Ctrl Pts',(-40.7659601690815,2.68383921778971,-3.17977892504124));
#26481=CARTESIAN_POINT('Ctrl Pts',(-40.7590378055941,3.08085732675141,-2.79683972378313));
#26482=CARTESIAN_POINT('Ctrl Pts',(-40.7464480969967,3.68905485419697,-1.91817431678888));
#26483=CARTESIAN_POINT('Ctrl Pts',(-40.7407828262988,3.90208612855456,-1.43605207520613));
#26484=CARTESIAN_POINT('Ctrl Pts',(-40.7276540591317,4.14018118830279,-0.403690208174394));
#26485=CARTESIAN_POINT('Ctrl Pts',(-40.7207144391096,4.15751878480496,0.138207480308497));
#26486=CARTESIAN_POINT('Ctrl Pts',(-40.7069342644054,3.98208570997053,1.20693859145346));
#26487=CARTESIAN_POINT('Ctrl Pts',(-40.7002333014212,3.78755871206735,1.72282249150634));
#26488=CARTESIAN_POINT('Ctrl Pts',(-40.6883542753676,3.22096473485822,2.62960385192518));
#26489=CARTESIAN_POINT('Ctrl Pts',(-40.6819551684805,2.86175752493203,3.01658708980989));
#26490=CARTESIAN_POINT('Ctrl Pts',(-40.668411685601,2.00155042900569,3.64758170969355));
#26491=CARTESIAN_POINT('Ctrl Pts',(-40.6613809279315,1.50403158161056,3.87929727322067));
#26492=CARTESIAN_POINT('Ctrl Pts',(-40.6479611935944,0.455056611180836,
4.13472350026447));
#26493=CARTESIAN_POINT('Ctrl Pts',(-40.6421321536017,-0.0855688602521068,
4.15880863776603));
#26494=CARTESIAN_POINT('Ctrl Pts',(-40.6295914262721,-1.1389622030828,3.99981076167824));
#26495=CARTESIAN_POINT('Ctrl Pts',(-40.6228999424275,-1.64221384336218,
3.82084385528187));
#26496=CARTESIAN_POINT('Ctrl Pts',(-40.609054644058,-2.57177890670439,3.27177288984792));
#26497=CARTESIAN_POINT('Ctrl Pts',(-40.6020319376635,-2.98488904384758,
2.89982556624254));
#26498=CARTESIAN_POINT('Ctrl Pts',(-40.5892031578238,-3.62498922247056,
2.03704695742646));
#26499=CARTESIAN_POINT('Ctrl Pts',(-40.5836087707956,-3.85415098979506,
1.56065010585271));
#26500=CARTESIAN_POINT('Ctrl Pts',(-40.5706005753391,-4.12484416838145,
0.536554513603813));
#26501=CARTESIAN_POINT('Ctrl Pts',(-40.5637021117861,-4.15959364278306,
-0.00274099528344514));
#26502=CARTESIAN_POINT('Ctrl Pts',(-40.5498917708271,-4.01970620139322,
-1.07506636337484));
#26503=CARTESIAN_POINT('Ctrl Pts',(-40.5431187668493,-3.84224905068353,
-1.59716557269067));
#26504=CARTESIAN_POINT('Ctrl Pts',(-40.5310338571766,-3.30639681266052,
-2.5210794364958));
#26505=CARTESIAN_POINT('Ctrl Pts',(-40.5249197608055,-2.96116162576673,
-2.91884190336009));
#26506=CARTESIAN_POINT('Ctrl Pts',(-40.5114905610946,-2.1252829111401,-3.57661556325932));
#26507=CARTESIAN_POINT('Ctrl Pts',(-40.5044761054092,-1.63779006275009,
-3.82448044806031));
#26508=CARTESIAN_POINT('Ctrl Pts',(-40.4929472200596,-0.752298941107392,
-4.07341167294306));
#26509=CARTESIAN_POINT('Ctrl Pts',(-40.4883815963868,-0.376643921628896,
-4.12499999999999));
#26510=CARTESIAN_POINT('Ctrl Pts',(-40.4841154631359,3.19883008970123E-14,
-4.12499999999999));
#26511=CARTESIAN_POINT('Origin',(-44.,0.,0.));
#26512=CARTESIAN_POINT('',(-40.1666154631359,-6.3588100377625E-15,-4.12499999999999));
#26513=CARTESIAN_POINT('',(-40.2459904640031,-1.4997732948127E-14,-4.12499999999999));
#26514=CARTESIAN_POINT('',(-44.,-5.05166804648282E-16,-4.12499999999999));
#26515=CARTESIAN_POINT('Ctrl Pts',(-40.2459904640031,-1.08246744900953E-14,
-4.12499999999999));
#26516=CARTESIAN_POINT('Ctrl Pts',(-40.2511645331132,-0.456802815521309,
-4.12499999999999));
#26517=CARTESIAN_POINT('Ctrl Pts',(-40.2567671388541,-0.911090653036704,
-4.04911424251985));
#26518=CARTESIAN_POINT('Ctrl Pts',(-40.2693950955372,-1.85330635565894,
-3.7243726598499));
#26519=CARTESIAN_POINT('Ctrl Pts',(-40.2763651340528,-2.32323014163459,
-3.45084036187277));
#26520=CARTESIAN_POINT('Ctrl Pts',(-40.2895969905501,-3.1186938864387,-2.7498247794128));
#26521=CARTESIAN_POINT('Ctrl Pts',(-40.295370610222,-3.44112113451425,-2.33376677506535));
#26522=CARTESIAN_POINT('Ctrl Pts',(-40.3077924387886,-3.92488219124724,
-1.38175408190277));
#26523=CARTESIAN_POINT('Ctrl Pts',(-40.3146697241653,-4.07315395093914,
-0.850501718841946));
#26524=CARTESIAN_POINT('Ctrl Pts',(-40.3284966127207,-4.15312669191325,
0.225206633704283));
#26525=CARTESIAN_POINT('Ctrl Pts',(-40.3353102446371,-4.08940826849617,
0.758896869890493));
#26526=CARTESIAN_POINT('Ctrl Pts',(-40.3481076346137,-3.76393320782021,
1.76846260293689));
#26527=CARTESIAN_POINT('Ctrl Pts',(-40.3537127053316,-3.5067823671733,2.23542637049589));
#26528=CARTESIAN_POINT('Ctrl Pts',(-40.3668198019382,-2.81818007320255,
3.0615266230001));
#26529=CARTESIAN_POINT('Ctrl Pts',(-40.3738589036421,-2.38763015013398,
3.40797625552582));
#26530=CARTESIAN_POINT('Ctrl Pts',(-40.3875897705407,-1.43485943880383,
3.90307719940798));
#26531=CARTESIAN_POINT('Ctrl Pts',(-40.3941585404323,-0.925473555718519,
4.05417566477752));
#26532=CARTESIAN_POINT('Ctrl Pts',(-40.4064711435521,0.141129194611049,
4.15847629606445));
#26533=CARTESIAN_POINT('Ctrl Pts',(-40.4126731645028,0.688894074985228,
4.10344704284241));
#26534=CARTESIAN_POINT('Ctrl Pts',(-40.4263460636897,1.72670495377073,3.78498780607248));
#26535=CARTESIAN_POINT('Ctrl Pts',(-40.4333449731268,2.20716624280072,3.52647983676792));
#26536=CARTESIAN_POINT('Ctrl Pts',(-40.446694767345,3.02656439153977,2.85089551558366));
#26537=CARTESIAN_POINT('Ctrl Pts',(-40.452649855385,3.3624468926465,2.4457386866896));
#26538=CARTESIAN_POINT('Ctrl Pts',(-40.4648729533427,3.87722024233396,1.51031000812043));
#26539=CARTESIAN_POINT('Ctrl Pts',(-40.4716908604004,4.04289787582651,0.984296996577499));
#26540=CARTESIAN_POINT('Ctrl Pts',(-40.4855130908483,4.15847552344624,-0.0898046715788642));
#26541=CARTESIAN_POINT('Ctrl Pts',(-40.4923794658442,4.11191518262026,-0.627009708846587));
#26542=CARTESIAN_POINT('Ctrl Pts',(-40.5053033001154,3.81898505439463,-1.64530163712721));
#26543=CARTESIAN_POINT('Ctrl Pts',(-40.5108820741256,3.57860195755648,-2.11784602213624));
#26544=CARTESIAN_POINT('Ctrl Pts',(-40.523824578453,2.91890677962931,-2.96599529937724));
#26545=CARTESIAN_POINT('Ctrl Pts',(-40.5308564517633,2.49860365386708,-3.32777991648706));
#26546=CARTESIAN_POINT('Ctrl Pts',(-40.544660418758,1.55934370916937,-3.85525585600394));
#26547=CARTESIAN_POINT('Ctrl Pts',(-40.5513046650687,1.05344357974458,-4.02303550703667));
#26548=CARTESIAN_POINT('Ctrl Pts',(-40.5595335155396,0.353662903039793,
-4.11364157625598));
#26549=CARTESIAN_POINT('Ctrl Pts',(-40.5614886034933,0.176738172163106,
-4.12499999999999));
#26550=CARTESIAN_POINT('Ctrl Pts',(-40.5634904640031,-1.23582119034381E-14,
-4.12499999999999));
#26551=CARTESIAN_POINT('Ctrl Pts',(-40.4841154631359,3.13681525934293E-14,
-4.12499999999999));
#26552=CARTESIAN_POINT('Ctrl Pts',(-40.4822753706969,0.162456161504383,
-4.12499999999999));
#26553=CARTESIAN_POINT('Ctrl Pts',(-40.4804812668311,0.325096198638992,
-4.11540312943268));
#26554=CARTESIAN_POINT('Ctrl Pts',(-40.4724651726939,1.01097481237393,-4.03384622077745));
#26555=CARTESIAN_POINT('Ctrl Pts',(-40.4658453438792,1.51809459276297,-3.87161030816205));
#26556=CARTESIAN_POINT('Ctrl Pts',(-40.4520641552773,2.46196947749767,-3.35487058828514));
#26557=CARTESIAN_POINT('Ctrl Pts',(-40.4450290293083,2.88574115794718,-2.99815834290086));
#26558=CARTESIAN_POINT('Ctrl Pts',(-40.4320311675825,3.55508263011756,-2.15730311961309));
#26559=CARTESIAN_POINT('Ctrl Pts',(-40.4264501489989,3.80103124624296,-1.68663302019211));
#26560=CARTESIAN_POINT('Ctrl Pts',(-40.41356824869,4.10485447069414,-0.671231557054981));
#26561=CARTESIAN_POINT('Ctrl Pts',(-40.4067187680204,4.15717619845452,-0.135143089765433));
#26562=CARTESIAN_POINT('Ctrl Pts',(-40.3928932925976,4.05351566546605,0.939627842130299));
#26563=CARTESIAN_POINT('Ctrl Pts',(-40.3860546662005,3.8936436306417,1.46745970374505));
#26564=CARTESIAN_POINT('Ctrl Pts',(-40.3737645744268,3.38922878719453,2.40847564516003));
#26565=CARTESIAN_POINT('Ctrl Pts',(-40.3678769712427,3.05787925922361,2.81726992195831));
#26566=CARTESIAN_POINT('Ctrl Pts',(-40.3545664420887,2.24651754008161,3.50144885572143));
#26567=CARTESIAN_POINT('Ctrl Pts',(-40.3475764048178,1.76955239567787,3.76505895019985));
#26568=CARTESIAN_POINT('Ctrl Pts',(-40.3338563021928,0.734137805202703,
4.09586277936751));
#26569=CARTESIAN_POINT('Ctrl Pts',(-40.3275628767339,0.184939966494483,
4.15702242121256));
#26570=CARTESIAN_POINT('Ctrl Pts',(-40.3152953798184,-0.884140561094941,
4.06332232400762));
#26571=CARTESIAN_POINT('Ctrl Pts',(-40.3087521921069,-1.39453225494303,
3.91759670981335));
#26572=CARTESIAN_POINT('Ctrl Pts',(-40.2950477641159,-2.35141623776284,
3.43296762105789));
#26573=CARTESIAN_POINT('Ctrl Pts',(-40.2880079578197,-2.78514593313154,
3.09150304024689));
#26574=CARTESIAN_POINT('Ctrl Pts',(-40.2748491081645,-3.48298625464293,
2.27257368934654));
#26575=CARTESIAN_POINT('Ctrl Pts',(-40.2692232582875,-3.74555545626104,
1.80737321559898));
#26576=CARTESIAN_POINT('Ctrl Pts',(-40.2564667705712,-4.0813718577666,0.800636742382464));
#26577=CARTESIAN_POINT('Ctrl Pts',(-40.2496713147319,-4.15050504243521,
0.26817515751442));
#26578=CARTESIAN_POINT('Ctrl Pts',(-40.2358461129982,-4.08184039453985,
-0.807796509791499));
#26579=CARTESIAN_POINT('Ctrl Pts',(-40.2289515579117,-3.93913465550836,
-1.3405902846371));
#26580=CARTESIAN_POINT('Ctrl Pts',(-40.2164675004409,-3.46526878917106,
-2.29780239688099));
#26581=CARTESIAN_POINT('Ctrl Pts',(-40.2107389342126,-3.14706448761942,
-2.71734678090657));
#26582=CARTESIAN_POINT('Ctrl Pts',(-40.1975449173483,-2.35915715275628,
-3.42629087401622));
#26583=CARTESIAN_POINT('Ctrl Pts',(-40.1905855070596,-1.8926366192759,-3.70445900981677));
#26584=CARTESIAN_POINT('Ctrl Pts',(-40.1777562548584,-0.940557438244165,
-4.0440739233157));
#26585=CARTESIAN_POINT('Ctrl Pts',(-40.1719586032874,-0.471729583234032,
-4.12499999999999));
#26586=CARTESIAN_POINT('Ctrl Pts',(-40.1666154631359,-1.2490009027033E-14,
-4.12499999999999));
#26587=CARTESIAN_POINT('Origin',(-44.,0.,0.));
#26588=CARTESIAN_POINT('',(-39.8491154631359,1.54314928943905E-14,-4.12499999999999));
#26589=CARTESIAN_POINT('',(-39.9284904639595,1.92328552709179E-9,-4.12499999999999));
#26590=CARTESIAN_POINT('',(-44.,-5.05166804648282E-16,-4.12499999999999));
#26591=CARTESIAN_POINT('Ctrl Pts',(-39.9284904639595,3.84657155935038E-9,
-4.12499999999999));
#26592=CARTESIAN_POINT('Ctrl Pts',(-39.9285613255899,-0.00625615385321784,
-4.12500000000582));
#26593=CARTESIAN_POINT('Ctrl Pts',(-39.9286322803852,-0.0125129692164882,
-4.12498576746479));
#26594=CARTESIAN_POINT('Ctrl Pts',(-39.9349035628237,-0.564849025000654,
-4.1224723921527));
#26595=CARTESIAN_POINT('Ctrl Pts',(-39.941689948868,-1.10503267883579,-4.01157400752992));
#26596=CARTESIAN_POINT('Ctrl Pts',(-39.9555044655837,-2.10060887504081,
-3.59016819890216));
#26597=CARTESIAN_POINT('Ctrl Pts',(-39.9623939550971,-2.54805930694276,
-3.28774431673863));
#26598=CARTESIAN_POINT('Ctrl Pts',(-39.9753778551158,-3.29493450649213,
-2.53651856164694));
#26599=CARTESIAN_POINT('Ctrl Pts',(-39.9809649441868,-3.59033631924146,
-2.09761859456588));
#26600=CARTESIAN_POINT('Ctrl Pts',(-39.9938268014861,-4.01099550328834,
-1.1090799748115));
#26601=CARTESIAN_POINT('Ctrl Pts',(-40.0008525107595,-4.12297601485987,
-0.564983189194966));
#26602=CARTESIAN_POINT('Ctrl Pts',(-40.0146865276618,-4.12689303188455,
0.5139371007478));
#26603=CARTESIAN_POINT('Ctrl Pts',(-40.0213646683409,-4.02706797150972,
1.03831985518209));
#26604=CARTESIAN_POINT('Ctrl Pts',(-40.0338794544559,-3.63181818055359,
2.0282789975544));
#26605=CARTESIAN_POINT('Ctrl Pts',(-40.0397430506145,-3.33720204469592,
2.48336578946497));
#26606=CARTESIAN_POINT('Ctrl Pts',(-40.0531927654037,-2.58585361099515,
3.25945141792043));
#26607=CARTESIAN_POINT('Ctrl Pts',(-40.0602210275196,-2.13465491468969,
3.57126156886965));
#26608=CARTESIAN_POINT('Ctrl Pts',(-40.073742936908,-1.15594403833876,3.99411127763624));
#26609=CARTESIAN_POINT('Ctrl Pts',(-40.0800829220566,-0.640771741663391,
4.10834777384782));
#26610=CARTESIAN_POINT('Ctrl Pts',(-40.0920014966045,0.427745727565198,
4.13893364113017));
#26611=CARTESIAN_POINT('Ctrl Pts',(-40.098716757312,0.971223994379406,4.04604143043629));
#26612=CARTESIAN_POINT('Ctrl Pts',(-40.1125038478542,1.9817777368465,3.65735823047392));
#26613=CARTESIAN_POINT('Ctrl Pts',(-40.1194361638857,2.44034969934498,3.36873983532249));
#26614=CARTESIAN_POINT('Ctrl Pts',(-40.132542232477,3.21090076698186,2.64175660037354));
#26615=CARTESIAN_POINT('Ctrl Pts',(-40.1381896593882,3.51943910808138,2.21411543790356));
#26616=CARTESIAN_POINT('Ctrl Pts',(-40.1508156422579,3.97037755423067,1.24503246284474));
#26617=CARTESIAN_POINT('Ctrl Pts',(-40.1577471034709,4.10017612521246,0.70890927187637));
#26618=CARTESIAN_POINT('Ctrl Pts',(-40.1715625963995,4.14275938969906,-0.367215887972643));
#26619=CARTESIAN_POINT('Ctrl Pts',(-40.1783135140328,4.06120060776941,-0.896637392098473));
#26620=CARTESIAN_POINT('Ctrl Pts',(-40.1909742296231,3.70150240323432,-1.89673758441462));
#26621=CARTESIAN_POINT('Ctrl Pts',(-40.1966712706875,3.42624545922335,-2.35787560203382));
#26622=CARTESIAN_POINT('Ctrl Pts',(-40.2099484456965,2.7069837021752,-3.15992951396612));
#26623=CARTESIAN_POINT('Ctrl Pts',(-40.21698685119,2.26606326514222,-3.4896804402072));
#26624=CARTESIAN_POINT('Ctrl Pts',(-40.2306241797491,1.30003232585709,-3.94980080559581));
#26625=CARTESIAN_POINT('Ctrl Pts',(-40.2371053097944,0.787513969953535,
-4.08299417523486));
#26626=CARTESIAN_POINT('Ctrl Pts',(-40.2440258670844,0.175867960167723,
-4.12219123871433));
#26627=CARTESIAN_POINT('Ctrl Pts',(-40.2449949899983,0.0878873703636625,
-4.12499999999999));
#26628=CARTESIAN_POINT('Ctrl Pts',(-40.2459904640031,-1.23582119034381E-14,
-4.12499999999999));
#26629=CARTESIAN_POINT('Ctrl Pts',(-40.1666154631359,-1.28833483865871E-14,
-4.12499999999999));
#26630=CARTESIAN_POINT('Ctrl Pts',(-40.1657875078361,0.0730976537079367,
-4.12499999999999));
#26631=CARTESIAN_POINT('Ctrl Pts',(-40.1649788014734,0.146265079272092,
-4.1230570124755));
#26632=CARTESIAN_POINT('Ctrl Pts',(-40.1582718697332,0.742907530787551,
-4.09127421296842));
#26633=CARTESIAN_POINT('Ctrl Pts',(-40.1518204403058,1.25630263379554,-3.96385298436616));
#26634=CARTESIAN_POINT('Ctrl Pts',(-40.1382165597341,2.22633704610043,-3.51505981705709));
#26635=CARTESIAN_POINT('Ctrl Pts',(-40.1311802244293,2.67046358955764,-3.19074426475465));
#26636=CARTESIAN_POINT('Ctrl Pts',(-40.1178496794716,3.39953551237553,-2.39653901600989));
#26637=CARTESIAN_POINT('Ctrl Pts',(-40.1121093274993,3.68066420103062,-1.93725311097702));
#26638=CARTESIAN_POINT('Ctrl Pts',(-40.0994929087377,4.05125765893966,-0.940227612697416));
#26639=CARTESIAN_POINT('Ctrl Pts',(-40.0927634815047,4.13844542904659,-0.412285797036978));
#26640=CARTESIAN_POINT('Ctrl Pts',(-40.0788880069208,4.10758931019005,0.668927469168811));
#26641=CARTESIAN_POINT('Ctrl Pts',(-40.0718758421793,3.98146853579977,1.21147398876256));
#26642=CARTESIAN_POINT('Ctrl Pts',(-40.0591457428114,3.5352567600302,2.18884313792248));
#26643=CARTESIAN_POINT('Ctrl Pts',(-40.053516493891,3.22959731636452,2.61892692349575));
#26644=CARTESIAN_POINT('Ctrl Pts',(-40.0404369540956,2.46422838844342,3.35125140856129));
#26645=CARTESIAN_POINT('Ctrl Pts',(-40.0335134405718,2.00806398201211,3.64293615791774));
#26646=CARTESIAN_POINT('Ctrl Pts',(-40.0197190068943,1.00070809848204,4.03885293655703));
#26647=CARTESIAN_POINT('Ctrl Pts',(-40.012987475074,0.457900809079785,4.13570878662521));
#26648=CARTESIAN_POINT('Ctrl Pts',(-40.0010231515811,-0.610513816318687,
4.11291266072887));
#26649=CARTESIAN_POINT('Ctrl Pts',(-39.9947489848203,-1.12619666349221,
4.00255897520987));
#26650=CARTESIAN_POINT('Ctrl Pts',(-39.9813041330625,-2.10360415532423,
3.58895883078212));
#26651=CARTESIAN_POINT('Ctrl Pts',(-39.9743327543442,-2.55378770749458,
3.28389183220121));
#26652=CARTESIAN_POINT('Ctrl Pts',(-39.9610959576698,-3.29947441517994,
2.53006645859444));
#26653=CARTESIAN_POINT('Ctrl Pts',(-39.9553159945307,-3.5926783721241,2.09294620363441));
#26654=CARTESIAN_POINT('Ctrl Pts',(-39.9429023435717,-4.01018999587605,
1.11009823057164));
#26655=CARTESIAN_POINT('Ctrl Pts',(-39.9360273756597,-4.1217821755761,0.569951981661034));
#26656=CARTESIAN_POINT('Ctrl Pts',(-39.9222003792236,-4.12800221666922,
-0.508774703888089));
#26657=CARTESIAN_POINT('Ctrl Pts',(-39.9153844187221,-4.02790805533635,
-1.03692610883357));
#26658=CARTESIAN_POINT('Ctrl Pts',(-39.9025817014483,-3.63412649732825,
-2.02179037792622));
#26659=CARTESIAN_POINT('Ctrl Pts',(-39.8969789036376,-3.34571628854063,
-2.46995843314048));
#26660=CARTESIAN_POINT('Ctrl Pts',(-39.8838786012199,-2.6023047713686,-3.24702630260162));
#26661=CARTESIAN_POINT('Ctrl Pts',(-39.8768396494237,-2.14900926008281,
-3.56327444715444));
#26662=CARTESIAN_POINT('Ctrl Pts',(-39.8631054381929,-1.16447139702274,
-3.99210612797126));
#26663=CARTESIAN_POINT('Ctrl Pts',(-39.8565333777027,-0.645872395426181,
-4.10801194929109));
#26664=CARTESIAN_POINT('Ctrl Pts',(-39.8500212029461,-0.0796584766999726,
-4.12442349205516));
#26665=CARTESIAN_POINT('Ctrl Pts',(-39.8495664599918,-0.0398171398878583,
-4.12499999999999));
#26666=CARTESIAN_POINT('Ctrl Pts',(-39.8491154631359,3.13681525934293E-14,
-4.12499999999999));
#26667=CARTESIAN_POINT('Origin',(-44.,0.,0.));
#26668=CARTESIAN_POINT('',(-39.5316154631359,1.25662602177568E-15,-4.12499999999999));
#26669=CARTESIAN_POINT('',(-39.6109904640031,-5.93380278614818E-15,-4.12499999999999));
#26670=CARTESIAN_POINT('',(-44.,-5.05166804648282E-16,-4.12499999999999));
#26671=CARTESIAN_POINT('Ctrl Pts',(-39.6109904640031,-1.23582119034381E-14,
-4.12499999999999));
#26672=CARTESIAN_POINT('Ctrl Pts',(-39.6120784864535,-0.0960581909754306,
-4.12499999999999));
#26673=CARTESIAN_POINT('Ctrl Pts',(-39.613187837006,-0.19221534304798,-4.12164472355536));
#26674=CARTESIAN_POINT('Ctrl Pts',(-39.620718248277,-0.833175183420811,
-4.07673814098845));
#26675=CARTESIAN_POINT('Ctrl Pts',(-39.6276223981309,-1.36507991359612,
-3.93071543675476));
#26676=CARTESIAN_POINT('Ctrl Pts',(-39.6414459366988,-2.32806042343033,
-3.44650803714958));
#26677=CARTESIAN_POINT('Ctrl Pts',(-39.6482306169486,-2.75243031666917,
-3.1180788842059));
#26678=CARTESIAN_POINT('Ctrl Pts',(-39.6609633880996,-3.45198123824481,
-2.31954745235684));
#26679=CARTESIAN_POINT('Ctrl Pts',(-39.6666039547501,-3.72112298136687,
-1.85734208907042));
#26680=CARTESIAN_POINT('Ctrl Pts',(-39.6797924788468,-4.0751413196876,-0.840996220796809));
#26681=CARTESIAN_POINT('Ctrl Pts',(-39.6868323341888,-4.15057896526983,
-0.294519932982031));
#26682=CARTESIAN_POINT('Ctrl Pts',(-39.7005208192468,-4.08541641084468,
0.77546114537168));
#26683=CARTESIAN_POINT('Ctrl Pts',(-39.7070489185251,-3.95345127565009,
1.28926298594501));
#26684=CARTESIAN_POINT('Ctrl Pts',(-39.7192901280476,-3.4940224803795,2.26012426002136));
#26685=CARTESIAN_POINT('Ctrl Pts',(-39.725639361951,-3.16294286667469,2.70410066801925));
#26686=CARTESIAN_POINT('Ctrl Pts',(-39.7393865290349,-2.35324967764201,
3.43057131862578));
#26687=CARTESIAN_POINT('Ctrl Pts',(-39.746371017253,-1.8849525637005,3.70857900625545));
#26688=CARTESIAN_POINT('Ctrl Pts',(-39.7596585323065,-0.884784462692935,
4.06260984891072));
#26689=CARTESIAN_POINT('Ctrl Pts',(-39.7655098995271,-0.364556442023356,
4.14182727479458));
#26690=CARTESIAN_POINT('Ctrl Pts',(-39.7778388660033,0.702376467574034,
4.10129005906997));
#26691=CARTESIAN_POINT('Ctrl Pts',(-39.784689191451,1.2386225047964,3.97236936493211));
#26692=CARTESIAN_POINT('Ctrl Pts',(-39.7985157764843,2.21803952075457,3.51856869125415));
#26693=CARTESIAN_POINT('Ctrl Pts',(-39.8053550443527,2.65387954852039,3.20264779831331));
#26694=CARTESIAN_POINT('Ctrl Pts',(-39.818212292288,3.37668007672995,2.42717394157867));
#26695=CARTESIAN_POINT('Ctrl Pts',(-39.8237976592278,3.65873908869338,1.97655506891192));
#26696=CARTESIAN_POINT('Ctrl Pts',(-39.8368277047136,4.0457284357555,0.973721948313611));
#26697=CARTESIAN_POINT('Ctrl Pts',(-39.8438643444358,4.13917345088107,0.428125310920622));
#26698=CARTESIAN_POINT('Ctrl Pts',(-39.857631459975,4.10795416376912,-0.646803641311481));
#26699=CARTESIAN_POINT('Ctrl Pts',(-39.864236648442,3.99173323773183,-1.16606865962808));
#26700=CARTESIAN_POINT('Ctrl Pts',(-39.8766147511517,3.56403405226136,-2.14649961709799));
#26701=CARTESIAN_POINT('Ctrl Pts',(-39.8826941077983,3.25123200088449,-2.59601571084602));
#26702=CARTESIAN_POINT('Ctrl Pts',(-39.8962967627661,2.47043449902232,-3.34747094998367));
#26703=CARTESIAN_POINT('Ctrl Pts',(-39.9033070700102,2.01034235308391,-3.64240738946468));
#26704=CARTESIAN_POINT('Ctrl Pts',(-39.9166344383974,1.02646869575269,-4.02837734110635));
#26705=CARTESIAN_POINT('Ctrl Pts',(-39.9226518744084,0.51547130702924,-4.12499999951931));
#26706=CARTESIAN_POINT('Ctrl Pts',(-39.9284904639595,3.84657155935038E-9,
-4.12499999999999));
#26707=CARTESIAN_POINT('Ctrl Pts',(-39.8491154631359,3.13681525934293E-14,
-4.12499999999999));
#26708=CARTESIAN_POINT('Ctrl Pts',(-39.843402485096,0.504381444880162,-4.12499999999999));
#26709=CARTESIAN_POINT('Ctrl Pts',(-39.8375223233553,1.00487152049101,-4.03248595035866));
#26710=CARTESIAN_POINT('Ctrl Pts',(-39.8243576494017,1.98112817703027,-3.65825910161386));
#26711=CARTESIAN_POINT('Ctrl Pts',(-39.8173576492924,2.44288280604376,-3.36749940249));
#26712=CARTESIAN_POINT('Ctrl Pts',(-39.8040027808205,3.21427799065912,-2.63744746711315));
#26713=CARTESIAN_POINT('Ctrl Pts',(-39.7980384429505,3.52170140820749,-2.21027615043971));
#26714=CARTESIAN_POINT('Ctrl Pts',(-39.7858240655497,3.97135752656289,-1.24184905854371));
#26715=CARTESIAN_POINT('Ctrl Pts',(-39.7790089067465,4.10070484310535,-0.705747913315952));
#26716=CARTESIAN_POINT('Ctrl Pts',(-39.7651872213033,4.1426232649795,0.373811128262174));
#26717=CARTESIAN_POINT('Ctrl Pts',(-39.7583187121852,4.05943945848419,0.906651862177761));
#26718=CARTESIAN_POINT('Ctrl Pts',(-39.7453894698742,3.69757339961626,1.90249963232007));
#26719=CARTESIAN_POINT('Ctrl Pts',(-39.7398105076248,3.42551234676977,2.35741774652478));
#26720=CARTESIAN_POINT('Ctrl Pts',(-39.7268751988628,2.70944016452086,3.15850728351391));
#26721=CARTESIAN_POINT('Ctrl Pts',(-39.7198438075971,2.26532985103266,3.49077489483737));
#26722=CARTESIAN_POINT('Ctrl Pts',(-39.7060370101051,1.29206995435841,3.95286983078476));
#26723=CARTESIAN_POINT('Ctrl Pts',(-39.6993896596857,0.775810073068537,
4.08567630966704));
#26724=CARTESIAN_POINT('Ctrl Pts',(-39.6869335551,-0.28970140984737,4.14999731159824));
#26725=CARTESIAN_POINT('Ctrl Pts',(-39.68098416215,-0.829144441797188,4.07663213774457));
#26726=CARTESIAN_POINT('Ctrl Pts',(-39.6674677452171,-1.85215882006829,
3.72549080996463));
#26727=CARTESIAN_POINT('Ctrl Pts',(-39.66044621068,-2.3254103729873,3.44996225448759));
#26728=CARTESIAN_POINT('Ctrl Pts',(-39.6469735531507,-3.12320577978043,
2.74483237311875));
#26729=CARTESIAN_POINT('Ctrl Pts',(-39.6407591472535,-3.44536102340515,
2.32765735044714));
#26730=CARTESIAN_POINT('Ctrl Pts',(-39.6287515009935,-3.9275052950731,1.37422083235662));
#26731=CARTESIAN_POINT('Ctrl Pts',(-39.6220048306236,-4.07472638121562,
0.8428376377412));
#26732=CARTESIAN_POINT('Ctrl Pts',(-39.6082041013904,-4.15295732985394,
-0.236354875145553));
#26733=CARTESIAN_POINT('Ctrl Pts',(-39.6012892767861,-4.08714456180461,
-0.773414839596819));
#26734=CARTESIAN_POINT('Ctrl Pts',(-39.5882351301151,-3.7577282036435,-1.78013835225203));
#26735=CARTESIAN_POINT('Ctrl Pts',(-39.5826206126713,-3.50185985590037,
-2.24196104421186));
#26736=CARTESIAN_POINT('Ctrl Pts',(-39.5698551236704,-2.81333837034102,
-3.06666841839316));
#26737=CARTESIAN_POINT('Ctrl Pts',(-39.5628389099864,-2.37893526329097,
-3.41467248922035));
#26738=CARTESIAN_POINT('Ctrl Pts',(-39.548973667415,-1.41801473088533,-3.90967882644601));
#26739=CARTESIAN_POINT('Ctrl Pts',(-39.5422575317382,-0.904628541834916,
-4.05931128723266));
#26740=CARTESIAN_POINT('Ctrl Pts',(-39.5344981490777,-0.2514509148248,-4.11925879260599));
#26741=CARTESIAN_POINT('Ctrl Pts',(-39.5330386994699,-0.125653204598835,
-4.12499999999999));
#26742=CARTESIAN_POINT('Ctrl Pts',(-39.5316154631359,-1.16920362280837E-14,
-4.12499999999999));
#26743=CARTESIAN_POINT('Origin',(-44.,0.,0.));
#26744=CARTESIAN_POINT('',(-39.2141154631359,7.39754712673358E-15,-4.12499999999999));
#26745=CARTESIAN_POINT('',(-39.2934904648176,-3.59547304179607E-8,-4.12499999999999));
#26746=CARTESIAN_POINT('',(-44.,-5.05166804648282E-16,-4.12499999999999));
#26747=CARTESIAN_POINT('Ctrl Pts',(-39.2934904644104,-3.5959404204311E-8,
-4.12499999999999));
#26748=CARTESIAN_POINT('Ctrl Pts',(-39.295599384249,-0.186190149588254,
-4.12499999837689));
#26749=CARTESIAN_POINT('Ctrl Pts',(-39.2977861373005,-0.372549332322611,
-4.11239426138431));
#26750=CARTESIAN_POINT('Ctrl Pts',(-39.3066474723105,-1.10195949492571,
-4.01284715042124));
#26751=CARTESIAN_POINT('Ctrl Pts',(-39.3136787388404,-1.62585126307851,
-3.83064734391326));
#26752=CARTESIAN_POINT('Ctrl Pts',(-39.3274862514165,-2.55341291536397,
-3.28248777516562));
#26753=CARTESIAN_POINT('Ctrl Pts',(-39.3341343886972,-2.95234017512007,
-2.92888007643203));
#26754=CARTESIAN_POINT('Ctrl Pts',(-39.3465919737327,-3.60175656712804,
-2.0817522056745));
#26755=CARTESIAN_POINT('Ctrl Pts',(-39.3525390739346,-3.84273753841753,
-1.59364873374324));
#26756=CARTESIAN_POINT('Ctrl Pts',(-39.3660538272193,-4.12408110394775,
-0.549319041224531));
#26757=CARTESIAN_POINT('Ctrl Pts',(-39.3730755497843,-4.16050319778585,
-0.00289466185195243));
#26758=CARTESIAN_POINT('Ctrl Pts',(-39.3865494573202,-4.02243009077466,
1.05289540411226));
#26759=CARTESIAN_POINT('Ctrl Pts',(-39.3927668921141,-3.85690107642523,
1.55332829300766));
#26760=CARTESIAN_POINT('Ctrl Pts',(-39.4047722979627,-3.33640726107213,
2.48639624480013));
#26761=CARTESIAN_POINT('Ctrl Pts',(-39.4115181919553,-2.97834694191541,
2.90572173604516));
#26762=CARTESIAN_POINT('Ctrl Pts',(-39.4253186114539,-2.12762856695797,
3.5743719592753));
#26763=CARTESIAN_POINT('Ctrl Pts',(-39.4322338938875,-1.6456533410096,3.82030970791316));
#26764=CARTESIAN_POINT('Ctrl Pts',(-39.4452893602645,-0.626933783143563,
4.11051693858186));
#26765=CARTESIAN_POINT('Ctrl Pts',(-39.4509045795661,-0.10101988185248,
4.15682431718069));
#26766=CARTESIAN_POINT('Ctrl Pts',(-39.4636682366469,0.967751936535434,
4.04756798604883));
#26767=CARTESIAN_POINT('Ctrl Pts',(-39.4706842480285,1.49925370884556,3.88221353574909));
#26768=CARTESIAN_POINT('Ctrl Pts',(-39.4845500362765,2.44718453842596,3.362686514528));
#26769=CARTESIAN_POINT('Ctrl Pts',(-39.4912668685653,2.85844670521885,3.02087103436019));
#26770=CARTESIAN_POINT('Ctrl Pts',(-39.5038578262864,3.53195717667501,2.19691185348038));
#26771=CARTESIAN_POINT('Ctrl Pts',(-39.5096259671741,3.78654151503228,1.72140910431719));
#26772=CARTESIAN_POINT('Ctrl Pts',(-39.5229867970177,4.10308374097648,0.690314646312808));
#26773=CARTESIAN_POINT('Ctrl Pts',(-39.5300215415094,4.15827215547997,0.143529887484189));
#26774=CARTESIAN_POINT('Ctrl Pts',(-39.5436055190979,4.05516751064371,-0.919624546867021));
#26775=CARTESIAN_POINT('Ctrl Pts',(-39.5500395984354,3.90571629799609,-1.42670343379841));
#26776=CARTESIAN_POINT('Ctrl Pts',(-39.5620085730998,3.41491132232603,-2.37742599538191));
#26777=CARTESIAN_POINT('Ctrl Pts',(-39.568601290936,3.07056680412132,-2.80809809184484));
#26778=CARTESIAN_POINT('Ctrl Pts',(-39.5823680755418,2.24055924177556,-3.50494474729392));
#26779=CARTESIAN_POINT('Ctrl Pts',(-39.5893210568637,1.76509769813185,-3.76685218921186));
#26780=CARTESIAN_POINT('Ctrl Pts',(-39.6012960044861,0.847192453867817,
-4.05944841020172));
#26781=CARTESIAN_POINT('Ctrl Pts',(-39.60618153575,0.424565640489271,-4.12499999999999));
#26782=CARTESIAN_POINT('Ctrl Pts',(-39.6109904640031,-1.23582119034381E-14,
-4.12499999999999));
#26783=CARTESIAN_POINT('Ctrl Pts',(-39.5316154631359,-1.28833483865871E-14,
-4.12499999999999));
#26784=CARTESIAN_POINT('Ctrl Pts',(-39.5270062407276,0.406934219222845,
-4.12499999999999));
#26785=CARTESIAN_POINT('Ctrl Pts',(-39.5223363198912,0.812347824891932,
-4.06477965010671));
#26786=CARTESIAN_POINT('Ctrl Pts',(-39.5105357603151,1.72348496276242,-3.78700521349252));
#26787=CARTESIAN_POINT('Ctrl Pts',(-39.5035011115944,2.20753977941869,-3.52683635719434));
#26788=CARTESIAN_POINT('Ctrl Pts',(-39.4899182410904,3.03101153407769,-2.84658455385363));
#26789=CARTESIAN_POINT('Ctrl Pts',(-39.4834851202791,3.3676748191655,-2.43902654846832));
#26790=CARTESIAN_POINT('Ctrl Pts',(-39.4715186405353,3.88107743642454,-1.50033645743129));
#26791=CARTESIAN_POINT('Ctrl Pts',(-39.4649229943107,4.04538718282125,-0.97397940572874));
#26792=CARTESIAN_POINT('Ctrl Pts',(-39.4511558042648,4.15859905583844,0.103818602234392));
#26793=CARTESIAN_POINT('Ctrl Pts',(-39.4442031826834,4.10967803484536,0.644416613965508));
#26794=CARTESIAN_POINT('Ctrl Pts',(-39.4310322347819,3.8115726491491,1.66134405757424));
#26795=CARTESIAN_POINT('Ctrl Pts',(-39.4253281053926,3.57095108017744,2.12989537645652));
#26796=CARTESIAN_POINT('Ctrl Pts',(-39.4128064587927,2.91287926763723,2.97138178254049));
#26797=CARTESIAN_POINT('Ctrl Pts',(-39.4059017891302,2.49426416236043,3.33055759347151));
#26798=CARTESIAN_POINT('Ctrl Pts',(-39.3920783566002,1.5541855677181,3.85781962416697));
#26799=CARTESIAN_POINT('Ctrl Pts',(-39.3852942749978,1.04456260395922,4.02581166954861));
#26800=CARTESIAN_POINT('Ctrl Pts',(-39.3725628105428,-0.00869603853111918,
4.15889866115016));
#26801=CARTESIAN_POINT('Ctrl Pts',(-39.3669213767033,-0.542409605992354,
4.12338532663788));
#26802=CARTESIAN_POINT('Ctrl Pts',(-39.3537312247787,-1.58288504110619,
3.84818211866607));
#26803=CARTESIAN_POINT('Ctrl Pts',(-39.346691374359,-2.07801866231148,3.60497786987691));
#26804=CARTESIAN_POINT('Ctrl Pts',(-39.3330037806798,-2.92838982685494,
2.95236901937931));
#26805=CARTESIAN_POINT('Ctrl Pts',(-39.3264765181129,-3.2804161839462,2.55554852638602));
#26806=CARTESIAN_POINT('Ctrl Pts',(-39.3142367598118,-3.82811724441854,
1.63154730083484));
#26807=CARTESIAN_POINT('Ctrl Pts',(-39.3078843912774,-4.01089579172321,
1.10867329980487));
#26808=CARTESIAN_POINT('Ctrl Pts',(-39.2941357396797,-4.16000209505153,
0.0310678347067559));
#26809=CARTESIAN_POINT('Ctrl Pts',(-39.2871515658459,-4.12841714503876,
-0.512596650218839));
#26810=CARTESIAN_POINT('Ctrl Pts',(-39.2738653240342,-3.86227563484386,
-1.5396332532564));
#26811=CARTESIAN_POINT('Ctrl Pts',(-39.2680158909314,-3.636872729621,-2.01514085728428));
#26812=CARTESIAN_POINT('Ctrl Pts',(-39.2556847820188,-3.00633714628252,
-2.87677781179184));
#26813=CARTESIAN_POINT('Ctrl Pts',(-39.2488338188269,-2.59945910740675,
-3.24911021753748));
#26814=CARTESIAN_POINT('Ctrl Pts',(-39.2350071893406,-1.67537468047583,
-3.80698373692771));
#26815=CARTESIAN_POINT('Ctrl Pts',(-39.2281684931446,-1.16969888523996,
-3.99146773122192));
#26816=CARTESIAN_POINT('Ctrl Pts',(-39.2190847694358,-0.429801702513547,
-4.1082178495998));
#26817=CARTESIAN_POINT('Ctrl Pts',(-39.21654878163,-0.214830284541508,-4.12499999999999));
#26818=CARTESIAN_POINT('Ctrl Pts',(-39.2141154631359,3.40005801291454E-14,
-4.12499999999999));
#26819=CARTESIAN_POINT('Origin',(-44.,0.,0.));
#26820=CARTESIAN_POINT('',(-38.8966154631359,-7.81597775758302E-15,-4.12499999999999));
#26821=CARTESIAN_POINT('',(-38.9759904640031,-5.04042019602013E-15,-4.12499999999999));
#26822=CARTESIAN_POINT('',(-44.,-5.05166804648282E-16,-4.12499999999999));
#26823=CARTESIAN_POINT('Ctrl Pts',(-38.9759904640031,-2.15105711021124E-14,
-4.12499999999999));
#26824=CARTESIAN_POINT('Ctrl Pts',(-38.9790474996013,-0.269896369513169,
-4.12499999999999));
#26825=CARTESIAN_POINT('Ctrl Pts',(-38.9822635574637,-0.539748106423213,
-4.09851142651325));
#26826=CARTESIAN_POINT('Ctrl Pts',(-38.992171577137,-1.33074276654309,-3.94099260355166));
#26827=CARTESIAN_POINT('Ctrl Pts',(-38.9990717182805,-1.83050192552105,
-3.73517849360003));
#26828=CARTESIAN_POINT('Ctrl Pts',(-39.0128811969529,-2.73228840497834,
-3.1382164174264));
#26829=CARTESIAN_POINT('Ctrl Pts',(-39.019651620186,-3.12327088774582,-2.74936196462474));
#26830=CARTESIAN_POINT('Ctrl Pts',(-39.0317288442979,-3.71769260733261,
-1.86196066114348));
#26831=CARTESIAN_POINT('Ctrl Pts',(-39.0378525559747,-3.92326379015565,
-1.37700840925209));
#26832=CARTESIAN_POINT('Ctrl Pts',(-39.0512861088709,-4.14674799464015,
-0.336991875673695));
#26833=CARTESIAN_POINT('Ctrl Pts',(-39.0583013204775,-4.15512014108993,
0.209904172918947));
#26834=CARTESIAN_POINT('Ctrl Pts',(-39.0718690354137,-3.96014727794907,
1.27499822485171));
#26835=CARTESIAN_POINT('Ctrl Pts',(-39.077893072742,-3.75894753442914,1.78288911644535));
#26836=CARTESIAN_POINT('Ctrl Pts',(-39.0903030835144,-3.17925708982892,
2.68074128890209));
#26837=CARTESIAN_POINT('Ctrl Pts',(-39.0969256833317,-2.81063365599906,
3.06502531008103));
#26838=CARTESIAN_POINT('Ctrl Pts',(-39.1107095013912,-1.93156464744709,
3.68586291261577));
#26839=CARTESIAN_POINT('Ctrl Pts',(-39.117744304952,-1.42484137660058,3.90977743641053));
#26840=CARTESIAN_POINT('Ctrl Pts',(-39.1307359923122,-0.375402464839822,
4.14144133452341));
#26841=CARTESIAN_POINT('Ctrl Pts',(-39.1363164342365,0.155364053080466,
4.15551749008611));
#26842=CARTESIAN_POINT('Ctrl Pts',(-39.1492030408596,1.20094621231838,3.98223276667685));
#26843=CARTESIAN_POINT('Ctrl Pts',(-39.1560544478221,1.70554863977671,3.79361951957827));
#26844=CARTESIAN_POINT('Ctrl Pts',(-39.1698796448005,2.62545931848446,3.22813418022329));
#26845=CARTESIAN_POINT('Ctrl Pts',(-39.1767159975248,3.02932345921329,2.85255943133749));
#26846=CARTESIAN_POINT('Ctrl Pts',(-39.1889986252139,3.65291444704421,1.98591158993573));
#26847=CARTESIAN_POINT('Ctrl Pts',(-39.1948934325522,3.87449493902384,1.50861745452681));
#26848=CARTESIAN_POINT('Ctrl Pts',(-39.2082083611995,4.13250053218192,0.479059158036542));
#26849=CARTESIAN_POINT('Ctrl Pts',(-39.215199430204,4.15966272975775,-0.065297597988825));
#26850=CARTESIAN_POINT('Ctrl Pts',(-39.2289143087603,4.00173529390893,-1.14057679742806));
#26851=CARTESIAN_POINT('Ctrl Pts',(-39.2351972511196,3.81540734251379,-1.66055888320928));
#26852=CARTESIAN_POINT('Ctrl Pts',(-39.2476992999592,3.25123845070424,-2.59678981543789));
#26853=CARTESIAN_POINT('Ctrl Pts',(-39.2545137578529,2.87926912340319,-3.0039422018544));
#26854=CARTESIAN_POINT('Ctrl Pts',(-39.2683353001993,2.00793250615844,-3.64270357598583));
#26855=CARTESIAN_POINT('Ctrl Pts',(-39.2752043497793,1.51973610071058,-3.87188436109807));
#26856=CARTESIAN_POINT('Ctrl Pts',(-39.2858533066883,0.673253899371989,
-4.08372402589253));
#26857=CARTESIAN_POINT('Ctrl Pts',(-39.2896744394388,0.336905193941784,
-4.12500000293694));
#26858=CARTESIAN_POINT('Ctrl Pts',(-39.2934904644104,-3.59594048395727E-8,
-4.12499999999999));
#26859=CARTESIAN_POINT('Ctrl Pts',(-39.2141154631359,3.13681525934293E-14,
-4.12499999999999));
#26860=CARTESIAN_POINT('Ctrl Pts',(-39.2106076395524,0.309695068855631,
-4.12499999999999));
#26861=CARTESIAN_POINT('Ctrl Pts',(-39.2071110024133,0.619094537650788,
-4.09012254664969));
#26862=CARTESIAN_POINT('Ctrl Pts',(-39.196695117648,1.45649361160747,-3.89803246967592));
#26863=CARTESIAN_POINT('Ctrl Pts',(-39.189658402646,1.96096703584027,-3.67023625977947));
#26864=CARTESIAN_POINT('Ctrl Pts',(-39.175892081298,2.83441544551272,-3.04297763892349));
#26865=CARTESIAN_POINT('Ctrl Pts',(-39.1692877099202,3.19977026976349,-2.65614420856511));
#26866=CARTESIAN_POINT('Ctrl Pts',(-39.1569110947223,3.77313686189122,-1.75308434849624));
#26867=CARTESIAN_POINT('Ctrl Pts',(-39.1508290874092,3.970725038286,-1.24226285192036));
#26868=CARTESIAN_POINT('Ctrl Pts',(-39.1372248150422,4.15669220016776,-0.174631796483549));
#26869=CARTESIAN_POINT('Ctrl Pts',(-39.1302147468664,4.14372093648504,0.371702458396875));
#26870=CARTESIAN_POINT('Ctrl Pts',(-39.1168097438426,3.91179105654006,1.40919716469096));
#26871=CARTESIAN_POINT('Ctrl Pts',(-39.1107473679707,3.70233301351323,1.89226394095644));
#26872=CARTESIAN_POINT('Ctrl Pts',(-39.0986199515878,3.10081981753944,2.77466222329187));
#26873=CARTESIAN_POINT('Ctrl Pts',(-39.0918328310287,2.70667356357166,3.16033897225272));
#26874=CARTESIAN_POINT('Ctrl Pts',(-39.0780180998527,1.80039426427184,3.74972342793978));
#26875=CARTESIAN_POINT('Ctrl Pts',(-39.0711291166307,1.29940843771414,3.95137781008399));
#26876=CARTESIAN_POINT('Ctrl Pts',(-39.0581465698181,0.258893382924898,
4.15012262690843));
#26877=CARTESIAN_POINT('Ctrl Pts',(-39.052559819976,-0.270180862102667,
4.14940293972721));
#26878=CARTESIAN_POINT('Ctrl Pts',(-39.039696128115,-1.32487355405879,3.94497537962508));
#26879=CARTESIAN_POINT('Ctrl Pts',(-39.0326702602678,-1.83847358117235,
3.73338043732847));
#26880=CARTESIAN_POINT('Ctrl Pts',(-39.018836886592,-2.73488704715773,3.13300998511365));
#26881=CARTESIAN_POINT('Ctrl Pts',(-39.0121594953428,-3.11365616207528,
2.75690245931389));
#26882=CARTESIAN_POINT('Ctrl Pts',(-38.9996461566451,-3.71307058463043,
1.87541539377217));
#26883=CARTESIAN_POINT('Ctrl Pts',(-38.9937805709011,-3.92545063473447,
1.3765600433662));
#26884=CARTESIAN_POINT('Ctrl Pts',(-38.9803291922002,-4.14831505802596,
0.319566254637141));
#26885=CARTESIAN_POINT('Ctrl Pts',(-38.9733010780177,-4.15430764739794,
-0.228837826006839));
#26886=CARTESIAN_POINT('Ctrl Pts',(-38.9597803760164,-3.95720546520464,
-1.27657329396925));
#26887=CARTESIAN_POINT('Ctrl Pts',(-38.9534436245317,-3.76366253628105,
-1.76746632844331));
#26888=CARTESIAN_POINT('Ctrl Pts',(-38.9415228464317,-3.19120408915522,
-2.67019767817732));
#26889=CARTESIAN_POINT('Ctrl Pts',(-38.9348067953756,-2.81014340061275,
-3.06868415908844));
#26890=CARTESIAN_POINT('Ctrl Pts',(-38.9210193349198,-1.92261251543051,
-3.6888011243803));
#26891=CARTESIAN_POINT('Ctrl Pts',(-38.9140874341518,-1.426848744064,-3.90740294846574));
#26892=CARTESIAN_POINT('Ctrl Pts',(-38.9036813911272,-0.606059342712801,
-4.09157961116413));
#26893=CARTESIAN_POINT('Ctrl Pts',(-38.9000492507543,-0.303158658804201,
-4.12499999999999));
#26894=CARTESIAN_POINT('Ctrl Pts',(-38.8966154631359,-1.16573417585641E-14,
-4.12499999999999));
#26895=CARTESIAN_POINT('Origin',(-44.,0.,0.));
#26896=CARTESIAN_POINT('',(-38.5791154631359,-1.5969178094674E-14,-4.12499999999999));
#26897=CARTESIAN_POINT('',(-38.6584904640031,5.29853172080164E-15,-4.12499999999999));
#26898=CARTESIAN_POINT('',(-44.,-5.05166804648282E-16,-4.12499999999999));
#26899=CARTESIAN_POINT('Ctrl Pts',(-38.6584904640031,-1.74860126378462E-14,
-4.12499999999999));
#26900=CARTESIAN_POINT('Ctrl Pts',(-38.6625193640772,-0.35569932642004,
-4.12499999999999));
#26901=CARTESIAN_POINT('Ctrl Pts',(-38.666816404744,-0.710608137653691,
-4.07899022355685));
#26902=CARTESIAN_POINT('Ctrl Pts',(-38.6780065172728,-1.57663101836591,
-3.8496956268941));
#26903=CARTESIAN_POINT('Ctrl Pts',(-38.6849802916811,-2.06544662779795,
-3.61107336014592));
#26904=CARTESIAN_POINT('Ctrl Pts',(-38.6987754840373,-2.93308426250075,
-2.95225879949218));
#26905=CARTESIAN_POINT('Ctrl Pts',(-38.7052301010454,-3.30053012312115,
-2.53481766159836));
#26906=CARTESIAN_POINT('Ctrl Pts',(-38.717423849814,-3.83713355243541,-1.60244055093468));
#26907=CARTESIAN_POINT('Ctrl Pts',(-38.7239243883266,-4.00977089429739,
-1.10142541046586));
#26908=CARTESIAN_POINT('Ctrl Pts',(-38.7375831250835,-4.16072925823174,
-0.0413118164422865));
#26909=CARTESIAN_POINT('Ctrl Pts',(-38.7446224123957,-4.12970481913612,
0.50883790280608));
#26910=CARTESIAN_POINT('Ctrl Pts',(-38.7578636131338,-3.85899534969774,
1.55110853918749));
#26911=CARTESIAN_POINT('Ctrl Pts',(-38.7635354456736,-3.62740470376424,
2.0346293191332));
#26912=CARTESIAN_POINT('Ctrl Pts',(-38.7762256240908,-2.99364950257224,
2.88717331827899));
#26913=CARTESIAN_POINT('Ctrl Pts',(-38.782990529657,-2.59743470686741,3.24823554430925));
#26914=CARTESIAN_POINT('Ctrl Pts',(-38.7968098485576,-1.67700368856532,
3.80810237752584));
#26915=CARTESIAN_POINT('Ctrl Pts',(-38.8037304728962,-1.15856033930691,
3.99646473989038));
#26916=CARTESIAN_POINT('Ctrl Pts',(-38.816313351069,-0.102058589372211,
4.15668864362566));
#26917=CARTESIAN_POINT('Ctrl Pts',(-38.8219822057465,0.424592352730211,
4.13620612943619));
#26918=CARTESIAN_POINT('Ctrl Pts',(-38.8351152300092,1.45659591667997,3.89646770657547));
#26919=CARTESIAN_POINT('Ctrl Pts',(-38.8420561961729,1.95105063724238,3.67389866493515));
#26920=CARTESIAN_POINT('Ctrl Pts',(-38.8558353355033,2.8340425270065,3.04662676057572));
#26921=CARTESIAN_POINT('Ctrl Pts',(-38.8625255368819,3.21196550207653,2.64518131664316));
#26922=CARTESIAN_POINT('Ctrl Pts',(-38.8744131495901,3.77755565123565,1.73769514038321));
#26923=CARTESIAN_POINT('Ctrl Pts',(-38.8808158529087,3.96732924442539,1.2449095827013));
#26924=CARTESIAN_POINT('Ctrl Pts',(-38.8943631979186,4.15610184752558,0.194805077521741));
#26925=CARTESIAN_POINT('Ctrl Pts',(-38.9013943947845,4.14557826576012,-0.353997679006895));
#26926=CARTESIAN_POINT('Ctrl Pts',(-38.9148084184843,3.91398593596523,-1.4083825527151));
#26927=CARTESIAN_POINT('Ctrl Pts',(-38.9206311516536,3.69810657045983,-1.90442421215133));
#26928=CARTESIAN_POINT('Ctrl Pts',(-38.9331767909217,3.09247613130066,-2.78071508509055));
#26929=CARTESIAN_POINT('Ctrl Pts',(-38.939870782221,2.71052692038369,-3.15417531195753));
#26930=CARTESIAN_POINT('Ctrl Pts',(-38.9537181636733,1.80870958177029,-3.74795834727925));
#26931=CARTESIAN_POINT('Ctrl Pts',(-38.9607402669324,1.29298833288854,-3.95560484262641));
#26932=CARTESIAN_POINT('Ctrl Pts',(-38.9703269021749,0.50324821785069,-4.10198003830776));
#26933=CARTESIAN_POINT('Ctrl Pts',(-38.9731406059396,0.251605295474299,
-4.12499999999999));
#26934=CARTESIAN_POINT('Ctrl Pts',(-38.9759904640031,-1.23582119034381E-14,
-4.12499999999999));
#26935=CARTESIAN_POINT('Ctrl Pts',(-38.8966154631359,-1.28833483865871E-14,
-4.12499999999999));
#26936=CARTESIAN_POINT('Ctrl Pts',(-38.8941551257047,0.217215704275863,
-4.12499999999999));
#26937=CARTESIAN_POINT('Ctrl Pts',(-38.8917389813284,0.434563195301831,
-4.10784292032265));
#26938=CARTESIAN_POINT('Ctrl Pts',(-38.8827081392599,1.18941421738817,-3.98739239222705));
#26939=CARTESIAN_POINT('Ctrl Pts',(-38.8757761772874,1.7063965454856,-3.79502410638837));
#26940=CARTESIAN_POINT('Ctrl Pts',(-38.8619608831417,2.62214532974901,-3.22825618620668));
#26941=CARTESIAN_POINT('Ctrl Pts',(-38.8552106323992,3.01531105470513,-2.8644701966738));
#26942=CARTESIAN_POINT('Ctrl Pts',(-38.8425513085925,3.64301874167191,-2.00678695994037));
#26943=CARTESIAN_POINT('Ctrl Pts',(-38.8368530051158,3.87124617766612,-1.52060326836833));
#26944=CARTESIAN_POINT('Ctrl Pts',(-38.8235741401363,4.13359596934735,-0.475686737312476));
#26945=CARTESIAN_POINT('Ctrl Pts',(-38.8165357861214,4.16021387590477,0.0742363049878281));
#26946=CARTESIAN_POINT('Ctrl Pts',(-38.8028994855135,4.00110661022955,1.13231530738008));
#26947=CARTESIAN_POINT('Ctrl Pts',(-38.7964192791794,3.82476576207119,1.63161520311227));
#26948=CARTESIAN_POINT('Ctrl Pts',(-38.7843295174402,3.28362068269884,2.55572269933035));
#26949=CARTESIAN_POINT('Ctrl Pts',(-38.777873816786,2.9167823001544,2.96753795432328));
#26950=CARTESIAN_POINT('Ctrl Pts',(-38.7641287818026,2.05008100550226,3.61978520293195));
#26951=CARTESIAN_POINT('Ctrl Pts',(-38.7571590663949,1.56047246954954,3.85624222065994));
#26952=CARTESIAN_POINT('Ctrl Pts',(-38.7439283948578,0.534412161839448,
4.12337198936735));
#26953=CARTESIAN_POINT('Ctrl Pts',(-38.7381562807806,0.00916916585072175,
4.15784836567742));
#26954=CARTESIAN_POINT('Ctrl Pts',(-38.7257324925636,-1.05056311073634,
4.02619700780108));
#26955=CARTESIAN_POINT('Ctrl Pts',(-38.7188546534834,-1.57384711308623,
3.85187515299262));
#26956=CARTESIAN_POINT('Ctrl Pts',(-38.7050277946806,-2.51017981893487,
3.31634719660548));
#26957=CARTESIAN_POINT('Ctrl Pts',(-38.698214722834,-2.91687171763236,2.96496643205763));
#26958=CARTESIAN_POINT('Ctrl Pts',(-38.6854186111024,-3.57158157041546,
2.13037376857811));
#26959=CARTESIAN_POINT('Ctrl Pts',(-38.6798129800651,-3.8147745344501,1.65595381201699));
#26960=CARTESIAN_POINT('Ctrl Pts',(-38.6667042550831,-4.11423373550093,
0.62301235783989));
#26961=CARTESIAN_POINT('Ctrl Pts',(-38.6596651194103,-4.16050790034444,
0.0723419343465299));
#26962=CARTESIAN_POINT('Ctrl Pts',(-38.6459350583739,-4.03783829815713,
-0.994322838177824));
#26963=CARTESIAN_POINT('Ctrl Pts',(-38.6393670794612,-3.87810220559565,
-1.50104886972644));
#26964=CARTESIAN_POINT('Ctrl Pts',(-38.6270558816207,-3.36781647438429,
-2.44350607415521));
#26965=CARTESIAN_POINT('Ctrl Pts',(-38.6208510972024,-3.01570572680273,
-2.86678197462549));
#26966=CARTESIAN_POINT('Ctrl Pts',(-38.6071767129135,-2.1710764440728,-3.5488095434222));
#26967=CARTESIAN_POINT('Ctrl Pts',(-38.6001780673964,-1.68802106886808,
-3.80239492397942));
#26968=CARTESIAN_POINT('Ctrl Pts',(-38.5883995110342,-0.789429385568951,
-4.06814385357856));
#26969=CARTESIAN_POINT('Ctrl Pts',(-38.5835941021609,-0.39540540970529,
-4.12499999999999));
#26970=CARTESIAN_POINT('Ctrl Pts',(-38.5791154631359,-6.57113252700015E-14,
-4.12499999999999));
#26971=CARTESIAN_POINT('Origin',(-44.,0.,0.));
#26972=CARTESIAN_POINT('',(-38.261615463136,-6.99207366342899E-13,-4.12499999999999));
#26973=CARTESIAN_POINT('',(-38.3409904640031,-2.68119626869167E-15,-4.12499999999999));
#26974=CARTESIAN_POINT('',(-44.,-5.05166804648282E-16,-4.12499999999999));
#26975=CARTESIAN_POINT('Ctrl Pts',(-38.3409904640031,2.84494650060196E-14,
-4.12499999999999));
#26976=CARTESIAN_POINT('Ctrl Pts',(-38.3460731333721,-0.448733410539718,
-4.12499999999999));
#26977=CARTESIAN_POINT('Ctrl Pts',(-38.3515687489139,-0.894988901034538,
-4.05177263444848));
#26978=CARTESIAN_POINT('Ctrl Pts',(-38.3641290304286,-1.83494582066274,
-3.7340199284862));
#26979=CARTESIAN_POINT('Ctrl Pts',(-38.3711518773069,-2.30958973180772,
-3.46059640334447));
#26980=CARTESIAN_POINT('Ctrl Pts',(-38.3846564814364,-3.12306575806814,
-2.74816899221892));
#26981=CARTESIAN_POINT('Ctrl Pts',(-38.3905897661896,-3.45496107975674,
-2.31715585160993));
#26982=CARTESIAN_POINT('Ctrl Pts',(-38.4030563636754,-3.92957274116637,
-1.36133166666959));
#26983=CARTESIAN_POINT('Ctrl Pts',(-38.4097092800234,-4.071454835502,-0.847357016752972));
#26984=CARTESIAN_POINT('Ctrl Pts',(-38.4235211144765,-4.15521847085631,
0.22704473077945));
#26985=CARTESIAN_POINT('Ctrl Pts',(-38.4305516010864,-4.0880889406769,0.777768810425782));
#26986=CARTESIAN_POINT('Ctrl Pts',(-38.4434739145985,-3.749699355543,1.79752959830024));
#26987=CARTESIAN_POINT('Ctrl Pts',(-38.4490534938235,-3.49067077741897,
2.25977347387685));
#26988=CARTESIAN_POINT('Ctrl Pts',(-38.4619924785919,-2.80719285316213,
3.06934466299846));
#26989=CARTESIAN_POINT('Ctrl Pts',(-38.4688648061341,-2.38636786388807,
3.40682445000972));
#26990=CARTESIAN_POINT('Ctrl Pts',(-38.4826854358763,-1.42907319461139,
3.9078899385387));
#26991=CARTESIAN_POINT('Ctrl Pts',(-38.4894955993512,-0.899727126113582,
4.06255516959346));
#26992=CARTESIAN_POINT('Ctrl Pts',(-38.5016942198358,0.164047634942325,
4.15461433304697));
#26993=CARTESIAN_POINT('Ctrl Pts',(-38.5076755410745,0.687592626235074,
4.10060475917359));
#26994=CARTESIAN_POINT('Ctrl Pts',(-38.5210395565078,1.70490817498503,3.79488758815944));
#26995=CARTESIAN_POINT('Ctrl Pts',(-38.5280414898454,2.18704462559348,3.5390280401939));
#26996=CARTESIAN_POINT('Ctrl Pts',(-38.5416969670434,3.02814092354596,2.85349529517244));
#26997=CARTESIAN_POINT('Ctrl Pts',(-38.547867103372,3.37792837628264,2.42933391002391));
#26998=CARTESIAN_POINT('Ctrl Pts',(-38.5601961270754,3.88417209712161,1.48534513332595));
#26999=CARTESIAN_POINT('Ctrl Pts',(-38.5667741100694,4.04190583936277,0.977768857113072));
#27000=CARTESIAN_POINT('Ctrl Pts',(-38.580514306922,4.16019826172762,-0.0898393663118697));
#27001=CARTESIAN_POINT('Ctrl Pts',(-38.5875529536404,4.11157098037679,-0.640553823867985));
#27002=CARTESIAN_POINT('Ctrl Pts',(-38.6006409460874,3.80769852020947,-1.67203224909574));
#27003=CARTESIAN_POINT('Ctrl Pts',(-38.6062398918612,3.56271849964873,-2.14506326699018));
#27004=CARTESIAN_POINT('Ctrl Pts',(-38.6190522367407,2.90477027887625,-2.97686140441376));
#27005=CARTESIAN_POINT('Ctrl Pts',(-38.6258723825032,2.49647225022286,-3.32671241854949));
#27006=CARTESIAN_POINT('Ctrl Pts',(-38.6396995077155,1.55772831997847,-3.85842079894035));
#27007=CARTESIAN_POINT('Ctrl Pts',(-38.6465702471808,1.03372763497844,-4.03055134652997));
#27008=CARTESIAN_POINT('Ctrl Pts',(-38.6548230212139,0.328042356742512,
-4.11522730771825));
#27009=CARTESIAN_POINT('Ctrl Pts',(-38.6566335954254,0.163937275725416,
-4.12499999999999));
#27010=CARTESIAN_POINT('Ctrl Pts',(-38.6584904640031,-1.23582119034381E-14,
-4.12499999999999));
#27011=CARTESIAN_POINT('Ctrl Pts',(-38.5791154631359,-5.54544126205271E-14,
-4.12499999999999));
#27012=CARTESIAN_POINT('Ctrl Pts',(-38.5777052984279,0.124499150524016,
-4.12499999999999));
#27013=CARTESIAN_POINT('Ctrl Pts',(-38.5763345689061,0.249135344500066,
-4.11936371508453));
#27014=CARTESIAN_POINT('Ctrl Pts',(-38.5686514172062,0.917403659595085,
-4.05860129543216));
#27015=CARTESIAN_POINT('Ctrl Pts',(-38.5618328524111,1.44608084437713,-3.90162976661254));
#27016=CARTESIAN_POINT('Ctrl Pts',(-38.5480104953561,2.40099318624483,-3.39649766423788));
#27017=CARTESIAN_POINT('Ctrl Pts',(-38.5411446346849,2.82019163732253,-3.05736616861612));
#27018=CARTESIAN_POINT('Ctrl Pts',(-38.528222099859,3.50032561853965,-2.24486338919386));
#27019=CARTESIAN_POINT('Ctrl Pts',(-38.522643354713,3.75751718053833,-1.78122293458685));
#27020=CARTESIAN_POINT('Ctrl Pts',(-38.5096991233565,4.09141308629972,-0.759909471639569));
#27021=CARTESIAN_POINT('Ctrl Pts',(-38.5026671363584,4.15612476431192,-0.209152794560566));
#27022=CARTESIAN_POINT('Ctrl Pts',(-38.4888638531382,4.06783773883121,0.864423994213772));
#27023=CARTESIAN_POINT('Ctrl Pts',(-38.4822203542193,3.9238733786363,1.37759136778585));
#27024=CARTESIAN_POINT('Ctrl Pts',(-38.4697714822992,3.44514179888959,2.33188908306655));
#27025=CARTESIAN_POINT('Ctrl Pts',(-38.4638107939175,3.11094493722129,2.76201665332028));
#27026=CARTESIAN_POINT('Ctrl Pts',(-38.4502862636308,2.29387538428945,3.47099423492359));
#27027=CARTESIAN_POINT('Ctrl Pts',(-38.4432656612203,1.81822607978738,3.74215421063642));
#27028=CARTESIAN_POINT('Ctrl Pts',(-38.4297991159506,0.808214524886094,
4.07863262096241));
#27029=CARTESIAN_POINT('Ctrl Pts',(-38.4235994038568,0.285791044091418,
4.14810329170106));
#27030=CARTESIAN_POINT('Ctrl Pts',(-38.411580817241,-0.780819452979407,
4.08706579109104));
#27031=CARTESIAN_POINT('Ctrl Pts',(-38.4048303659324,-1.31438245457892,
3.9479329072716));
#27032=CARTESIAN_POINT('Ctrl Pts',(-38.3910281491536,-2.28719728908359,
3.47441347868357));
#27033=CARTESIAN_POINT('Ctrl Pts',(-38.3841155735743,-2.71876148407847,
3.14819940317982));
#27034=CARTESIAN_POINT('Ctrl Pts',(-38.3710678815349,-3.4245630366514,2.35836231288253));
#27035=CARTESIAN_POINT('Ctrl Pts',(-38.3654566966874,-3.69584460745119,
1.90531768684261));
#27036=CARTESIAN_POINT('Ctrl Pts',(-38.3526822593364,-4.06402646341166,
0.896050910667726));
#27037=CARTESIAN_POINT('Ctrl Pts',(-38.3456650689886,-4.14724396373961,
0.345802138784072));
#27038=CARTESIAN_POINT('Ctrl Pts',(-38.3318025171984,-4.09366352410783,
-0.733609595231798));
#27039=CARTESIAN_POINT('Ctrl Pts',(-38.3250897978148,-3.96571863384391,
-1.25273559605927));
#27040=CARTESIAN_POINT('Ctrl Pts',(-38.312507079564,-3.51843465170034,-2.21857153579474));
#27041=CARTESIAN_POINT('Ctrl Pts',(-38.3067294990485,-3.20159152013847,
-2.65542024677681));
#27042=CARTESIAN_POINT('Ctrl Pts',(-38.2933589300789,-2.41190819510755,
-3.39033953816649));
#27043=CARTESIAN_POINT('Ctrl Pts',(-38.2863247626057,-1.94414638530157,
-3.67858612594586));
#27044=CARTESIAN_POINT('Ctrl Pts',(-38.2731805804295,-0.974777894902451,
-4.03797668959702));
#27045=CARTESIAN_POINT('Ctrl Pts',(-38.2671563241853,-0.489185759583953,
-4.12499999999983));
#27046=CARTESIAN_POINT('Ctrl Pts',(-38.261615463136,-1.3759826611448E-12,
-4.12499999999999));
#27047=CARTESIAN_POINT('Origin',(-44.,0.,0.));
#27048=CARTESIAN_POINT('',(-37.9441154631359,-4.83767438976534E-15,-4.12499999999999));
#27049=CARTESIAN_POINT('',(-38.0234904636412,1.59756785521265E-8,-4.12499999999999));
#27050=CARTESIAN_POINT('',(-44.,-5.05166804648282E-16,-4.12499999999999));
#27051=CARTESIAN_POINT('Ctrl Pts',(-38.0234904638221,1.59777359460301E-8,
-4.12499999999999));
#27052=CARTESIAN_POINT('Ctrl Pts',(-38.0237043202452,-0.0188807168282395,
-4.12500000007312));
#27053=CARTESIAN_POINT('Ctrl Pts',(-38.0239190251932,-0.037767437987376,
-4.12487037046446));
#27054=CARTESIAN_POINT('Ctrl Pts',(-38.030132982982,-0.582400873088368,
-4.11738886468603));
#27055=CARTESIAN_POINT('Ctrl Pts',(-38.036666147453,-1.10194175114423,-4.00971289103375));
#27056=CARTESIAN_POINT('Ctrl Pts',(-38.0503600124608,-2.0915695050058,-3.59715313532195));
#27057=CARTESIAN_POINT('Ctrl Pts',(-38.0573998806197,-2.54913449809062,
-3.28878256199403));
#27058=CARTESIAN_POINT('Ctrl Pts',(-38.0705785109338,-3.30574968149235,
-2.52354132989884));
#27059=CARTESIAN_POINT('Ctrl Pts',(-38.0762139412877,-3.60216899750856,
-2.07860995930911));
#27060=CARTESIAN_POINT('Ctrl Pts',(-38.0889546415996,-4.01127620085621,
-1.09911821341874));
#27061=CARTESIAN_POINT('Ctrl Pts',(-38.0957429434606,-4.11941725962378,
-0.573405193795346));
#27062=CARTESIAN_POINT('Ctrl Pts',(-38.109567093331,-4.13030764530197,0.504501949583931));
#27063=CARTESIAN_POINT('Ctrl Pts',(-38.1164680692199,-4.02729010836241,
1.04637739463638));
#27064=CARTESIAN_POINT('Ctrl Pts',(-38.1289758842185,-3.62528197375484,
2.03602879459263));
#27065=CARTESIAN_POINT('Ctrl Pts',(-38.1346887608154,-3.33882262695728,
2.47797306655773));
#27066=CARTESIAN_POINT('Ctrl Pts',(-38.1478682160114,-2.6053850947198,3.24296611051257));
#27067=CARTESIAN_POINT('Ctrl Pts',(-38.1548233679752,-2.16083706612372,
3.55466482608879));
#27068=CARTESIAN_POINT('Ctrl Pts',(-38.1685876557074,-1.16965371430349,
3.99320900259259));
#27069=CARTESIAN_POINT('Ctrl Pts',(-38.1751626900788,-0.631358802437693,
4.11280596691297));
#27070=CARTESIAN_POINT('Ctrl Pts',(-38.1871468020538,0.438465805498592,
4.134968133176));
#27071=CARTESIAN_POINT('Ctrl Pts',(-38.1935866920777,0.95966217178111,4.04589330651222));
#27072=CARTESIAN_POINT('Ctrl Pts',(-38.207177364227,1.95982939445767,3.67028992410267));
#27073=CARTESIAN_POINT('Ctrl Pts',(-38.2142126717834,2.42655689980747,3.37990878902027));
#27074=CARTESIAN_POINT('Ctrl Pts',(-38.2275634299127,3.21277574063565,2.6417632140657));
#27075=CARTESIAN_POINT('Ctrl Pts',(-38.2333220673957,3.52745304345701,2.20406743014782));
#27076=CARTESIAN_POINT('Ctrl Pts',(-38.2459215193518,3.97074923950501,1.23678700030555));
#27077=CARTESIAN_POINT('Ctrl Pts',(-38.2526425728528,4.09664290430123,0.716939305680258));
#27078=CARTESIAN_POINT('Ctrl Pts',(-38.2665116457084,4.14579456083928,-0.363135729722965));
#27079=CARTESIAN_POINT('Ctrl Pts',(-38.2735264080823,4.06022308534345,-0.913277321608179));
#27080=CARTESIAN_POINT('Ctrl Pts',(-38.2862789110268,3.68769584072957,-1.92098495243211));
#27081=CARTESIAN_POINT('Ctrl Pts',(-38.2918985471915,3.4146152650931,-2.37269647451847));
#27082=CARTESIAN_POINT('Ctrl Pts',(-38.3049620365485,2.70553536602887,-3.15961094780644));
#27083=CARTESIAN_POINT('Ctrl Pts',(-38.3118800875951,2.27241232352458,-3.48413580392644));
#27084=CARTESIAN_POINT('Ctrl Pts',(-38.3256785830878,1.2973759659784,-3.95355263983835));
#27085=CARTESIAN_POINT('Ctrl Pts',(-38.3324197327732,0.763230661045134,
-4.09038534611251));
#27086=CARTESIAN_POINT('Ctrl Pts',(-38.339364533471,0.145294655553673,-4.12308259222839));
#27087=CARTESIAN_POINT('Ctrl Pts',(-38.3401679774318,0.0726148363152235,
-4.12499999999999));
#27088=CARTESIAN_POINT('Ctrl Pts',(-38.3409904640031,3.27860210979314E-14,
-4.12499999999999));
#27089=CARTESIAN_POINT('Ctrl Pts',(-38.261615463136,-1.38636031551329E-12,
-4.12499999999999));
#27090=CARTESIAN_POINT('Ctrl Pts',(-38.2612299027003,0.0340399574915664,
-4.125));
#27091=CARTESIAN_POINT('Ctrl Pts',(-38.260846682765,0.0680973155369406,
-4.12457864916165));
#27092=CARTESIAN_POINT('Ctrl Pts',(-38.2543646522353,0.648015297153039,
-4.11021134172938));
#27093=CARTESIAN_POINT('Ctrl Pts',(-38.2477546034083,1.18579871497768,-3.98844139822242));
#27094=CARTESIAN_POINT('Ctrl Pts',(-38.2339854518078,2.17498861886444,-3.54599154814852));
#27095=CARTESIAN_POINT('Ctrl Pts',(-38.2270346006617,2.61812006051472,-3.23265848310332));
#27096=CARTESIAN_POINT('Ctrl Pts',(-38.2138695437158,3.34850409647604,-2.46489685055937));
#27097=CARTESIAN_POINT('Ctrl Pts',(-38.2081712912561,3.63328432239769,-2.02174111422272));
#27098=CARTESIAN_POINT('Ctrl Pts',(-38.1956400875167,4.03140816708781,-1.03040102852718));
#27099=CARTESIAN_POINT('Ctrl Pts',(-38.1887328847935,4.13227712503136,-0.488114918740732));
#27100=CARTESIAN_POINT('Ctrl Pts',(-38.1749099932757,4.11711234980687,0.589544807818989));
#27101=CARTESIAN_POINT('Ctrl Pts',(-38.1681288515778,4.00696696566288,1.11462934019106));
#27102=CARTESIAN_POINT('Ctrl Pts',(-38.1554037880281,3.59402685237509,2.09276756622477));
#27103=CARTESIAN_POINT('Ctrl Pts',(-38.1497580216216,3.29558782142648,2.53688925902393));
#27104=CARTESIAN_POINT('Ctrl Pts',(-38.1365599064696,2.53566351202438,3.29914226321505));
#27105=CARTESIAN_POINT('Ctrl Pts',(-38.1295200916333,2.07704592276241,3.60552433718027));
#27106=CARTESIAN_POINT('Ctrl Pts',(-38.1158368839312,1.08617970980033,4.01398531250382));
#27107=CARTESIAN_POINT('Ctrl Pts',(-38.1093137281357,0.5664222643215,4.11959210542275));
#27108=CARTESIAN_POINT('Ctrl Pts',(-38.0970810830802,-0.507902906672018,
4.13023294250604));
#27109=CARTESIAN_POINT('Ctrl Pts',(-38.0907132693152,-1.05227289152958,
4.02610542998951));
#27110=CARTESIAN_POINT('Ctrl Pts',(-38.0769573558672,-2.05953550630973,
3.61452533619776));
#27111=CARTESIAN_POINT('Ctrl Pts',(-38.0699747351249,-2.51395801148782,
3.31458834453322));
#27112=CARTESIAN_POINT('Ctrl Pts',(-38.0566947382491,-3.26897144918954,
2.56933397632723));
#27113=CARTESIAN_POINT('Ctrl Pts',(-38.0508546849896,-3.5673225554335,2.13584965034781));
#27114=CARTESIAN_POINT('Ctrl Pts',(-38.0385130804182,-3.99655631436128,
1.15821196910055));
#27115=CARTESIAN_POINT('Ctrl Pts',(-38.0316590036003,-4.11462839855131,
0.619468947952946));
#27116=CARTESIAN_POINT('Ctrl Pts',(-38.0178321816844,-4.13383456908287,
-0.459697610602726));
#27117=CARTESIAN_POINT('Ctrl Pts',(-38.0109962994696,-4.03987288087036,
-0.989617065277204));
#27118=CARTESIAN_POINT('Ctrl Pts',(-37.9981471168202,-3.65770806718893,
-1.97851131193549));
#27119=CARTESIAN_POINT('Ctrl Pts',(-37.9925598467427,-3.37529914618813,
-2.4291338025587));
#27120=CARTESIAN_POINT('Ctrl Pts',(-37.979519328704,-2.64186452265411,-3.21503866544509));
#27121=CARTESIAN_POINT('Ctrl Pts',(-37.9724822573282,-2.1918677657622,-3.53717863291173));
#27122=CARTESIAN_POINT('Ctrl Pts',(-37.9587198550079,-1.21133133076715,
-3.97821685582181));
#27123=CARTESIAN_POINT('Ctrl Pts',(-37.9521195020808,-0.693525696132982,
-4.10031256189765));
#27124=CARTESIAN_POINT('Ctrl Pts',(-37.9453813564874,-0.111165010097093,
-4.12387746693034));
#27125=CARTESIAN_POINT('Ctrl Pts',(-37.9447447827213,-0.0555607109844483,
-4.12499999999999));
#27126=CARTESIAN_POINT('Ctrl Pts',(-37.9441154631359,3.30485893395059E-14,
-4.12499999999999));
#27127=CARTESIAN_POINT('Origin',(-44.,0.,0.));
#27128=CARTESIAN_POINT('',(-37.6266154631359,1.21767103030497E-14,-4.12499999999999));
#27129=CARTESIAN_POINT('',(-37.7059904640031,7.79577065882059E-16,-4.12499999999999));
#27130=CARTESIAN_POINT('',(-44.,-5.05166804648282E-16,-4.12499999999999));
#27131=CARTESIAN_POINT('Ctrl Pts',(-37.7059904640031,3.11209391590239E-14,
-4.12499999999999));
#27132=CARTESIAN_POINT('Ctrl Pts',(-37.7071719154616,-0.104306753770122,
-4.12499999999999));
#27133=CARTESIAN_POINT('Ctrl Pts',(-37.7083785054262,-0.208729338301771,
-4.12104375753856));
#27134=CARTESIAN_POINT('Ctrl Pts',(-37.7158245362891,-0.840548388610822,
-4.07295667726032));
#27135=CARTESIAN_POINT('Ctrl Pts',(-37.7225071923448,-1.35543391274962,
-3.93170313299287));
#27136=CARTESIAN_POINT('Ctrl Pts',(-37.7363450634051,-2.32263846728263,
-3.45306018718478));
#27137=CARTESIAN_POINT('Ctrl Pts',(-37.7433697948314,-2.76194610528908,
-3.11286588078123));
#27138=CARTESIAN_POINT('Ctrl Pts',(-37.7562205470214,-3.4642312144117,-2.29988670946835));
#27139=CARTESIAN_POINT('Ctrl Pts',(-37.7618098369706,-3.72815632765471,
-1.84152882982802));
#27140=CARTESIAN_POINT('Ctrl Pts',(-37.7748019154436,-4.07382258539091,
-0.840214112469761));
#27141=CARTESIAN_POINT('Ctrl Pts',(-37.7816944504239,-4.14835405482069,
-0.305197208511262));
#27142=CARTESIAN_POINT('Ctrl Pts',(-37.7955076304459,-4.08830380309599,
0.774331585360137));
#27143=CARTESIAN_POINT('Ctrl Pts',(-37.8022895529962,-3.95000804636215,
1.30815278024656));
#27144=CARTESIAN_POINT('Ctrl Pts',(-37.8144012239025,-3.48410861140897,
2.2691359668022));
#27145=CARTESIAN_POINT('Ctrl Pts',(-37.8204824693978,-3.16936772350144,
2.69130321045133));
#27146=CARTESIAN_POINT('Ctrl Pts',(-37.8338964591907,-2.38482443113829,
3.40901070340842));
#27147=CARTESIAN_POINT('Ctrl Pts',(-37.8409081934389,-1.91729343823775,
3.69225241593301));
#27148=CARTESIAN_POINT('Ctrl Pts',(-37.8545010384649,-0.898986506707305,
4.06217004115416));
#27149=CARTESIAN_POINT('Ctrl Pts',(-37.8605644897187,-0.358038443827645,
4.14502149368244));
#27150=CARTESIAN_POINT('Ctrl Pts',(-37.872951594501,0.710296533020388,4.09746768838102));
#27151=CARTESIAN_POINT('Ctrl Pts',(-37.8795617176277,1.22780524901194,3.97319128026447));
#27152=CARTESIAN_POINT('Ctrl Pts',(-37.8933336100623,2.20689647277595,3.52785923744461));
#27153=CARTESIAN_POINT('Ctrl Pts',(-37.9003697746898,2.65571311685408,3.20365036036623));
#27154=CARTESIAN_POINT('Ctrl Pts',(-37.9133890534834,3.38562313401503,2.41464331803595));
#27155=CARTESIAN_POINT('Ctrl Pts',(-37.9189727139994,3.66592175967749,1.96315157358555));
#27156=CARTESIAN_POINT('Ctrl Pts',(-37.9318382317976,4.04397461112516,0.972839587999278));
#27157=CARTESIAN_POINT('Ctrl Pts',(-37.9386809484601,4.13575917118188,0.442311017554957));
#27158=CARTESIAN_POINT('Ctrl Pts',(-37.9525072262703,4.11195377324833,-0.636973709161365));
#27159=CARTESIAN_POINT('Ctrl Pts',(-37.9593536664618,3.99159250933317,-1.17520101129804));
#27160=CARTESIAN_POINT('Ctrl Pts',(-37.9716696337007,3.55821552618004,-2.15098365823107));
#27161=CARTESIAN_POINT('Ctrl Pts',(-37.9775328773114,3.25803487894005,-2.58318509027641));
#27162=CARTESIAN_POINT('Ctrl Pts',(-37.9908281067754,2.49971153859421,-3.32538326764968));
#27163=CARTESIAN_POINT('Ctrl Pts',(-37.9978144833221,2.0437958034592,-3.62348308224314));
#27164=CARTESIAN_POINT('Ctrl Pts',(-38.0113139570659,1.0527773045935,-4.02333612530768));
#27165=CARTESIAN_POINT('Ctrl Pts',(-38.017501564914,0.528741675688592,-4.12499999795197));
#27166=CARTESIAN_POINT('Ctrl Pts',(-38.0234904638221,1.59777359460301E-8,
-4.12499999999999));
#27167=CARTESIAN_POINT('Ctrl Pts',(-37.9441154631359,3.30485893395059E-14,
-4.12499999999999));
#27168=CARTESIAN_POINT('Ctrl Pts',(-37.9386082192858,0.486217799373158,
-4.12499999999999));
#27169=CARTESIAN_POINT('Ctrl Pts',(-37.9329560684286,0.969089658383457,
-4.03902823711872));
#27170=CARTESIAN_POINT('Ctrl Pts',(-37.9200428786222,1.93393206262313,-3.68352885891709));
#27171=CARTESIAN_POINT('Ctrl Pts',(-37.9130339975976,2.39997383235154,-3.39832360911064));
#27172=CARTESIAN_POINT('Ctrl Pts',(-37.8996352616012,3.18110574425277,-2.6774006466607));
#27173=CARTESIAN_POINT('Ctrl Pts',(-37.893585808979,3.49394459573158,-2.25394013855885));
#27174=CARTESIAN_POINT('Ctrl Pts',(-37.8814474411251,3.9556418650188,-1.29102132570522));
#27175=CARTESIAN_POINT('Ctrl Pts',(-37.874656726913,4.09162469796749,-0.756595147888483));
#27176=CARTESIAN_POINT('Ctrl Pts',(-37.8608409692424,4.1469792361025,0.322970725341458));
#27177=CARTESIAN_POINT('Ctrl Pts',(-37.8539544842789,4.0702029115977,0.857437334283189));
#27178=CARTESIAN_POINT('Ctrl Pts',(-37.8409785885251,3.72034108541746,1.85734328266859));
#27179=CARTESIAN_POINT('Ctrl Pts',(-37.8353934033817,3.45431900223811,2.31480906659922));
#27180=CARTESIAN_POINT('Ctrl Pts',(-37.8225207064847,2.7484693577872,3.12472810048405));
#27181=CARTESIAN_POINT('Ctrl Pts',(-37.8154940725128,2.30790932846725,3.46288290694763));
#27182=CARTESIAN_POINT('Ctrl Pts',(-37.8016638830572,1.33911603179397,3.93726238194202));
#27183=CARTESIAN_POINT('Ctrl Pts',(-37.7949901848288,0.823862854142894,
4.07633708048196));
#27184=CARTESIAN_POINT('Ctrl Pts',(-37.7824839641823,-0.239538409426059,
4.15294827975522));
#27185=CARTESIAN_POINT('Ctrl Pts',(-37.7766085001214,-0.777902064061751,
4.08646922985062));
#27186=CARTESIAN_POINT('Ctrl Pts',(-37.7631489523892,-1.80425003631519,
3.74902840221135));
#27187=CARTESIAN_POINT('Ctrl Pts',(-37.7561215790285,-2.28160006467931,
3.47919986955755));
#27188=CARTESIAN_POINT('Ctrl Pts',(-37.7426068202433,-3.08904281714978,
2.78331574416901));
#27189=CARTESIAN_POINT('Ctrl Pts',(-37.7362858709818,-3.41662368201338,
2.36974547436992));
#27190=CARTESIAN_POINT('Ctrl Pts',(-37.7243542611244,-3.91051726854039,
1.42182952121731));
#27191=CARTESIAN_POINT('Ctrl Pts',(-37.7176343347561,-4.06417530920901,
0.892307582580152));
#27192=CARTESIAN_POINT('Ctrl Pts',(-37.7038450797497,-4.15557849765509,
-0.18644992224989));
#27193=CARTESIAN_POINT('Ctrl Pts',(-37.6969152330419,-4.09610964510732,
-0.72490314925878));
#27194=CARTESIAN_POINT('Ctrl Pts',(-37.6838166935475,-3.77847646188367,
-1.73550079173319));
#27195=CARTESIAN_POINT('Ctrl Pts',(-37.6781747173947,-3.52838754139827,
-2.19984681245613));
#27196=CARTESIAN_POINT('Ctrl Pts',(-37.6654712927782,-2.84980298586446,
-3.0329374391025));
#27197=CARTESIAN_POINT('Ctrl Pts',(-37.6584623742839,-2.41900734548028,
-3.38651484829051));
#27198=CARTESIAN_POINT('Ctrl Pts',(-37.6445796147704,-1.46276901221373,
-3.89323569776352));
#27199=CARTESIAN_POINT('Ctrl Pts',(-37.6378403980949,-0.950543086530867,
-4.048882749067));
#27200=CARTESIAN_POINT('Ctrl Pts',(-37.6298547851239,-0.2821464109366,-4.11777148580024));
#27201=CARTESIAN_POINT('Ctrl Pts',(-37.6282124466366,-0.140992813189271,
-4.12499999999999));
#27202=CARTESIAN_POINT('Ctrl Pts',(-37.6266154631359,3.37577188425087E-14,
-4.12499999999999));
#27203=CARTESIAN_POINT('Origin',(-44.,0.,0.));
#27204=CARTESIAN_POINT('',(-37.3091154631359,-1.27599396641169E-14,-4.12499999999999));
#27205=CARTESIAN_POINT('',(-37.3884904640031,2.95665502823295E-15,-4.12499999999999));
#27206=CARTESIAN_POINT('',(-44.,-5.05166804648282E-16,-4.12499999999999));
#27207=CARTESIAN_POINT('Ctrl Pts',(-37.3884904640031,4.18415302405606E-14,
-4.12499999999999));
#27208=CARTESIAN_POINT('Ctrl Pts',(-37.3906677996739,-0.192230340109688,
-4.12499999999999));
#27209=CARTESIAN_POINT('Ctrl Pts',(-37.3929279773324,-0.384630026067662,
-4.11156311004193));
#27210=CARTESIAN_POINT('Ctrl Pts',(-37.401674325966,-1.10297693745552,-4.01030180346646));
#27211=CARTESIAN_POINT('Ctrl Pts',(-37.4084846352612,-1.61082675698653,
-3.8346200178468));
#27212=CARTESIAN_POINT('Ctrl Pts',(-37.4223113259809,-2.54358162617868,
-3.29304306127044));
#27213=CARTESIAN_POINT('Ctrl Pts',(-37.4291918755208,-2.95678364777868,
-2.9276917129905));
#27214=CARTESIAN_POINT('Ctrl Pts',(-37.4416252892661,-3.60205440330305,
-2.07678052243481));
#27215=CARTESIAN_POINT('Ctrl Pts',(-37.447390089747,-3.83558733235126,-1.60501985013439));
#27216=CARTESIAN_POINT('Ctrl Pts',(-37.4606149346607,-4.11889089965305,
-0.583371534056672));
#27217=CARTESIAN_POINT('Ctrl Pts',(-37.467583052079,-4.15979311380797,-0.0412848199325075));
#27218=CARTESIAN_POINT('Ctrl Pts',(-37.4814017227819,-4.02940642868627,
1.04112845091884));
#27219=CARTESIAN_POINT('Ctrl Pts',(-37.4879109192177,-3.85417530706214,
1.57015298071717));
#27220=CARTESIAN_POINT('Ctrl Pts',(-37.5000810653711,-3.31937920069351,
2.5045662885685));
#27221=CARTESIAN_POINT('Ctrl Pts',(-37.50656775067,-2.9740844161738,2.9061905084859));
#27222=CARTESIAN_POINT('Ctrl Pts',(-37.5202112442221,-2.13546138659101,
3.57111304049778));
#27223=CARTESIAN_POINT('Ctrl Pts',(-37.5272499413056,-1.64514211144103,
3.82185219420493));
#27224=CARTESIAN_POINT('Ctrl Pts',(-37.5405169107563,-0.608441543413077,
4.11439654700987));
#27225=CARTESIAN_POINT('Ctrl Pts',(-37.5462064780509,-0.0734792402402831,
4.15849241465475));
#27226=CARTESIAN_POINT('Ctrl Pts',(-37.5588755836663,0.982700030052533,
4.0412526122613));
#27227=CARTESIAN_POINT('Ctrl Pts',(-37.5656305098631,1.4940702052209,3.88138766260919));
#27228=CARTESIAN_POINT('Ctrl Pts',(-37.5794471667734,2.44163648718631,3.36933297200938));
#27229=CARTESIAN_POINT('Ctrl Pts',(-37.5863755880347,2.86585992415229,3.01676109756999));
#27230=CARTESIAN_POINT('Ctrl Pts',(-37.5989893459416,3.53739310751232,2.18529735335871));
#27231=CARTESIAN_POINT('Ctrl Pts',(-37.6046425622615,3.78549972323502,1.72007830282347));
#27232=CARTESIAN_POINT('Ctrl Pts',(-37.6177562976578,4.09906719353762,0.708153398053445));
#27233=CARTESIAN_POINT('Ctrl Pts',(-37.6246911044208,4.15634329523982,0.169236712848066));
#27234=CARTESIAN_POINT('Ctrl Pts',(-37.6384759248595,4.06039816119926,-0.909333502735539));
#27235=CARTESIAN_POINT('Ctrl Pts',(-37.6451863953515,3.90452636076152,-1.43819518664312));
#27236=CARTESIAN_POINT('Ctrl Pts',(-37.6570916539256,3.40658457875049,-2.38419709865056));
#27237=CARTESIAN_POINT('Ctrl Pts',(-37.6634513160399,3.07712163443936,-2.79652624400761));
#27238=CARTESIAN_POINT('Ctrl Pts',(-37.6769805095977,2.26634299259602,-3.48919522994443));
#27239=CARTESIAN_POINT('Ctrl Pts',(-37.6840096457051,1.78758898584713,-3.75703623297596));
#27240=CARTESIAN_POINT('Ctrl Pts',(-37.69614742799,0.859635779401281,-4.0575058335108));
#27241=CARTESIAN_POINT('Ctrl Pts',(-37.7011108218793,0.430808752928153,
-4.12499999999999));
#27242=CARTESIAN_POINT('Ctrl Pts',(-37.7059904640031,3.27860210979314E-14,
-4.12499999999999));
#27243=CARTESIAN_POINT('Ctrl Pts',(-37.6266154631359,3.30485893395059E-14,
-4.12499999999999));
#27244=CARTESIAN_POINT('Ctrl Pts',(-37.6221989279767,0.389922448398557,
-4.12499999999999));
#27245=CARTESIAN_POINT('Ctrl Pts',(-37.6177368604089,0.778610707645908,
-4.06970972028326));
#27246=CARTESIAN_POINT('Ctrl Pts',(-37.6061774717959,1.67744214455319,-3.80771903698248));
#27247=CARTESIAN_POINT('Ctrl Pts',(-37.5991400897554,2.16520677060958,-3.55308503701036));
#27248=CARTESIAN_POINT('Ctrl Pts',(-37.5855208910561,2.99763324700018,-2.88181979463759));
#27249=CARTESIAN_POINT('Ctrl Pts',(-37.5790559484525,3.3393912706149,-2.47773399156515));
#27250=CARTESIAN_POINT('Ctrl Pts',(-37.5670063158095,3.86377204801705,-1.54438058168654));
#27251=CARTESIAN_POINT('Ctrl Pts',(-37.5605061416315,4.03407359169118,-1.01986013443005));
#27252=CARTESIAN_POINT('Ctrl Pts',(-37.5467534095254,4.15957777932814,0.0572394073939091));
#27253=CARTESIAN_POINT('Ctrl Pts',(-37.5397891031469,4.11662669254909,0.598957311171912));
#27254=CARTESIAN_POINT('Ctrl Pts',(-37.5265779358719,3.8295442392963,1.61940680611599));
#27255=CARTESIAN_POINT('Ctrl Pts',(-37.5208297206459,3.59420851434151,2.09034623789868));
#27256=CARTESIAN_POINT('Ctrl Pts',(-37.5083737788738,2.94567772194275,2.93886682586154));
#27257=CARTESIAN_POINT('Ctrl Pts',(-37.5014869460186,2.53108990773232,3.30265518170488));
#27258=CARTESIAN_POINT('Ctrl Pts',(-37.4876607917416,1.59645131974599,3.84060030559607));
#27259=CARTESIAN_POINT('Ctrl Pts',(-37.4808570234391,1.08813968038432,4.01432744434325));
#27260=CARTESIAN_POINT('Ctrl Pts',(-37.4680819755915,0.0369768069942605,
4.1585927484698));
#27261=CARTESIAN_POINT('Ctrl Pts',(-37.462466281356,-0.495884696062968,
4.12908705952985));
#27262=CARTESIAN_POINT('Ctrl Pts',(-37.4493308252688,-1.53893880112688,
3.86605651225515));
#27263=CARTESIAN_POINT('Ctrl Pts',(-37.4422912410479,-2.03738512301656,
3.62819285141658));
#27264=CARTESIAN_POINT('Ctrl Pts',(-37.4285746493976,-2.89589644148774,
2.98434527946527));
#27265=CARTESIAN_POINT('Ctrl Pts',(-37.4220197839471,-3.25260783241754,
2.59096193869904));
#27266=CARTESIAN_POINT('Ctrl Pts',(-37.4097317835589,-3.8093108483045,1.67427029362598));
#27267=CARTESIAN_POINT('Ctrl Pts',(-37.4034805956724,-3.99731289323383,
1.15565172979563));
#27268=CARTESIAN_POINT('Ctrl Pts',(-37.3897818306433,-4.15940421165096,
0.0814839838693053));
#27269=CARTESIAN_POINT('Ctrl Pts',(-37.3827876581262,-4.13433674295738,
-0.463187996524866));
#27270=CARTESIAN_POINT('Ctrl Pts',(-37.3694592448157,-3.88018263989796,
-1.49393259741077));
#27271=CARTESIAN_POINT('Ctrl Pts',(-37.3635417973747,-3.66040480140604,
-1.97207483992736));
#27272=CARTESIAN_POINT('Ctrl Pts',(-37.3512821135096,-3.04009209338073,
-2.8410785534224));
#27273=CARTESIAN_POINT('Ctrl Pts',(-37.3444528046473,-2.63765796626467,
-3.21817317843681));
#27274=CARTESIAN_POINT('Ctrl Pts',(-37.3306285945402,-1.7197367339296,-3.78723625854297));
#27275=CARTESIAN_POINT('Ctrl Pts',(-37.3237713357021,-1.21565176041362,
-3.97779436157307));
#27276=CARTESIAN_POINT('Ctrl Pts',(-37.3144537986562,-0.461036086366698,
-4.10568623576393));
#27277=CARTESIAN_POINT('Ctrl Pts',(-37.3117258674995,-0.230464657033585,
-4.12499999999999));
#27278=CARTESIAN_POINT('Ctrl Pts',(-37.3091154631359,-5.72458747072346E-14,
-4.12499999999999));
#27279=CARTESIAN_POINT('Origin',(-44.,0.,0.));
#27280=CARTESIAN_POINT('',(-36.9916154631359,-6.98331048911415E-15,-4.12499999999999));
#27281=CARTESIAN_POINT('',(-37.0709904640031,-1.50158430502744E-15,-4.12499999999999));
#27282=CARTESIAN_POINT('',(-44.,-5.05166804648282E-16,-4.12499999999999));
#27283=CARTESIAN_POINT('Ctrl Pts',(-37.0709904640031,2.24126273096203E-14,
-4.12499999999999));
#27284=CARTESIAN_POINT('Ctrl Pts',(-37.0741641489576,-0.280194986185825,
-4.12499999999999));
#27285=CARTESIAN_POINT('Ctrl Pts',(-37.0775086187982,-0.560288405338992,
-4.09645124016517));
#27286=CARTESIAN_POINT('Ctrl Pts',(-37.0875708944323,-1.36059888724556,
-3.93083971226053));
#27287=CARTESIAN_POINT('Ctrl Pts',(-37.0944813021594,-1.85915471210682,
-3.72105775932517));
#27288=CARTESIAN_POINT('Ctrl Pts',(-37.1082849003488,-2.75658981046722,
-3.11688834223419));
#27289=CARTESIAN_POINT('Ctrl Pts',(-37.1150389453404,-3.14452540889099,
-2.72502303584165));
#27290=CARTESIAN_POINT('Ctrl Pts',(-37.1270679765999,-3.73215915556418,
-1.83285752755093));
#27291=CARTESIAN_POINT('Ctrl Pts',(-37.1332538109737,-3.93401179253985,
-1.34608573887598));
#27292=CARTESIAN_POINT('Ctrl Pts',(-37.1467145081879,-4.1493789780694,-0.303668488579494));
#27293=CARTESIAN_POINT('Ctrl Pts',(-37.1537341990965,-4.15333077001792,
0.243731308968634));
#27294=CARTESIAN_POINT('Ctrl Pts',(-37.1672664587256,-3.94973777493262,
1.30636085895795));
#27295=CARTESIAN_POINT('Ctrl Pts',(-37.1732380847386,-3.74508229813653,
1.81145242736624));
#27296=CARTESIAN_POINT('Ctrl Pts',(-37.1856800465032,-3.15931852012689,
2.70428532402661));
#27297=CARTESIAN_POINT('Ctrl Pts',(-37.1923198543581,-2.78756277088135,
3.08608794801719));
#27298=CARTESIAN_POINT('Ctrl Pts',(-37.2061197479408,-1.903122333998,3.70069422731297));
#27299=CARTESIAN_POINT('Ctrl Pts',(-37.2131522829967,-1.39425855236916,
3.92084951372823));
#27300=CARTESIAN_POINT('Ctrl Pts',(-37.2261050125298,-0.343180026940343,
4.14415866512579));
#27301=CARTESIAN_POINT('Ctrl Pts',(-37.2316837078612,0.187054260758582,
4.15413466165872));
#27302=CARTESIAN_POINT('Ctrl Pts',(-37.2445998403375,1.2311046276491,3.97306647640316));
#27303=CARTESIAN_POINT('Ctrl Pts',(-37.2514631582721,1.7346373170358,3.78046360371346));
#27304=CARTESIAN_POINT('Ctrl Pts',(-37.2652861146008,2.65045053277971,3.20764410291976));
#27305=CARTESIAN_POINT('Ctrl Pts',(-37.2721079053092,3.05137392703989,2.82895654410468));
#27306=CARTESIAN_POINT('Ctrl Pts',(-37.2843433905178,3.66823469864112,1.95747871483541));
#27307=CARTESIAN_POINT('Ctrl Pts',(-37.2902855230812,3.88611550536358,1.47844008591746));
#27308=CARTESIAN_POINT('Ctrl Pts',(-37.3036280948907,4.13620649609111,0.44644923125366));
#27309=CARTESIAN_POINT('Ctrl Pts',(-37.3106254296513,4.15906352642556,-0.0985465952050307));
#27310=CARTESIAN_POINT('Ctrl Pts',(-37.3243071099761,3.99258790290023,-1.17153483285406));
#27311=CARTESIAN_POINT('Ctrl Pts',(-37.3305255755067,3.8028239865781,-1.68871883264315));
#27312=CARTESIAN_POINT('Ctrl Pts',(-37.3428298566585,3.24307198872039,-2.60292603704322));
#27313=CARTESIAN_POINT('Ctrl Pts',(-37.3493939366953,2.88477608020006,-2.99512911363186));
#27314=CARTESIAN_POINT('Ctrl Pts',(-37.3631200144422,2.02351857378712,-3.63597730023228));
#27315=CARTESIAN_POINT('Ctrl Pts',(-37.3701593059518,1.52395907130064,-3.87201644098539));
#27316=CARTESIAN_POINT('Ctrl Pts',(-37.3809217526081,0.667410969169671,
-4.08444198854481));
#27317=CARTESIAN_POINT('Ctrl Pts',(-37.3847077705848,0.333962490054018,
-4.12499999999999));
#27318=CARTESIAN_POINT('Ctrl Pts',(-37.3884904640031,3.27860210979314E-14,
-4.12499999999999));
#27319=CARTESIAN_POINT('Ctrl Pts',(-37.3091154631359,-5.54544126205271E-14,
-4.12499999999999));
#27320=CARTESIAN_POINT('Ctrl Pts',(-37.3057961344788,0.293053425445313,
-4.125));
#27321=CARTESIAN_POINT('Ctrl Pts',(-37.302496572808,0.585932270930643,-4.09377041876538));
#27322=CARTESIAN_POINT('Ctrl Pts',(-37.2923184130573,1.40993297946147,-3.91520855680477));
#27323=CARTESIAN_POINT('Ctrl Pts',(-37.2852846637679,1.91770377245598,-3.69312550545327));
#27324=CARTESIAN_POINT('Ctrl Pts',(-37.2714929077765,2.79939846988331,-3.07532218924127));
#27325=CARTESIAN_POINT('Ctrl Pts',(-37.26486186999,3.1695519937379,-2.6922455727142));
#27326=CARTESIAN_POINT('Ctrl Pts',(-37.2524362455398,3.75220749517648,-1.79684166298536));
#27327=CARTESIAN_POINT('Ctrl Pts',(-37.246438196426,3.95509588538512,-1.29031930269742));
#27328=CARTESIAN_POINT('Ctrl Pts',(-37.2328877493134,4.15428070878072,-0.226425060803106));
#27329=CARTESIAN_POINT('Ctrl Pts',(-37.225870294532,4.14806623944732,0.320721303783965));
#27330=CARTESIAN_POINT('Ctrl Pts',(-37.2124234556353,3.92854411626132,1.36191250792841));
#27331=CARTESIAN_POINT('Ctrl Pts',(-37.2062698062463,3.72479007920702,1.84775199830548));
#27332=CARTESIAN_POINT('Ctrl Pts',(-37.1942161120231,3.13368508465123,2.73748416652482));
#27333=CARTESIAN_POINT('Ctrl Pts',(-37.18745364341,2.74418912893683,3.12781355623797));
#27334=CARTESIAN_POINT('Ctrl Pts',(-37.1736469341447,1.84452264352381,3.7283029189356));
#27335=CARTESIAN_POINT('Ctrl Pts',(-37.1667417260539,1.34534790700189,3.93605750193924));
#27336=CARTESIAN_POINT('Ctrl Pts',(-37.1537148623995,0.307264370469522,
4.14673386817001));
#27337=CARTESIAN_POINT('Ctrl Pts',(-37.1481133025172,-0.2210657191477,4.15222126708393));
#27338=CARTESIAN_POINT('Ctrl Pts',(-37.1353101195756,-1.27811474097495,
3.96046567143204));
#27339=CARTESIAN_POINT('Ctrl Pts',(-37.1282899220348,-1.79481368830906,
3.75466415770538));
#27340=CARTESIAN_POINT('Ctrl Pts',(-37.1144363003646,-2.69913083967334,
3.16396370377404));
#27341=CARTESIAN_POINT('Ctrl Pts',(-37.1077347087709,-3.08255434702908,
2.79174481769875));
#27342=CARTESIAN_POINT('Ctrl Pts',(-37.095174106695,-3.6910726054665,1.91787434655503));
#27343=CARTESIAN_POINT('Ctrl Pts',(-37.0893701180906,-3.9085740653729,1.42313422703085));
#27344=CARTESIAN_POINT('Ctrl Pts',(-37.0759735564863,-4.14421102863299,
0.369970159798663));
#27345=CARTESIAN_POINT('Ctrl Pts',(-37.0689410874436,-4.15683990406862,
-0.179005345339644));
#27346=CARTESIAN_POINT('Ctrl Pts',(-37.0553814777069,-3.97193906272694,
-1.2302017074355));
#27347=CARTESIAN_POINT('Ctrl Pts',(-37.0489683455837,-3.78391418135595,
-1.72386178107584));
#27348=CARTESIAN_POINT('Ctrl Pts',(-37.0370537589836,-3.22150191021418,
-2.63356290217202));
#27349=CARTESIAN_POINT('Ctrl Pts',(-37.0303963268061,-2.84501717177573,
-3.03638425298011));
#27350=CARTESIAN_POINT('Ctrl Pts',(-37.0166210877952,-1.96412316641114,
-3.66695408089926));
#27351=CARTESIAN_POINT('Ctrl Pts',(-37.0096760739643,-1.47028239282131,
-3.89134987815664));
#27352=CARTESIAN_POINT('Ctrl Pts',(-36.9990436040111,-0.636218269325341,
-4.0881571656051));
#27353=CARTESIAN_POINT('Ctrl Pts',(-36.9952207715431,-0.318301707262144,
-4.12499999999999));
#27354=CARTESIAN_POINT('Ctrl Pts',(-36.9916154631359,3.06699110552699E-14,
-4.12499999999999));
#27355=CARTESIAN_POINT('Origin',(-44.,0.,0.));
#27356=CARTESIAN_POINT('',(-36.6741154631359,1.03986187401735E-14,-4.12499999999999));
#27357=CARTESIAN_POINT('',(-36.7534904640031,-3.56666810882749E-16,-4.12499999999999));
#27358=CARTESIAN_POINT('',(-44.,-5.05166804648282E-16,-4.12499999999999));
#27359=CARTESIAN_POINT('Ctrl Pts',(-36.7534904640031,2.82412981889024E-14,
-4.12499999999999));
#27360=CARTESIAN_POINT('Ctrl Pts',(-36.7576415599671,-0.366487629658998,
-4.12499999999999));
#27361=CARTESIAN_POINT('Ctrl Pts',(-36.7620762393622,-0.732041526592343,
-4.07615668580182));
#27362=CARTESIAN_POINT('Ctrl Pts',(-36.7734266674402,-1.60705638319277,
-3.83715416268648));
#27363=CARTESIAN_POINT('Ctrl Pts',(-36.7804077774656,-2.09434991444426,
-3.59445125081873));
#27364=CARTESIAN_POINT('Ctrl Pts',(-36.7941706433496,-2.9557531315232,-2.92927906028107));
#27365=CARTESIAN_POINT('Ctrl Pts',(-36.8005534185697,-3.31900785527471,
-2.51024406353054));
#27366=CARTESIAN_POINT('Ctrl Pts',(-36.8127792310965,-3.8484799759449,-1.57511694023483));
#27367=CARTESIAN_POINT('Ctrl Pts',(-36.8192984335145,-4.01764523711922,
-1.07252476234264));
#27368=CARTESIAN_POINT('Ctrl Pts',(-36.8329774021165,-4.16097543710129,
-0.0105666975561747));
#27369=CARTESIAN_POINT('Ctrl Pts',(-36.840017164917,-4.12583163241094,0.539763961332355));
#27370=CARTESIAN_POINT('Ctrl Pts',(-36.8532229045633,-3.84732929524882,
1.5795407558575));
#27371=CARTESIAN_POINT('Ctrl Pts',(-36.8588729602128,-3.61259971164264,
2.06058580728881));
#27372=CARTESIAN_POINT('Ctrl Pts',(-36.87159188163,-2.9731886495747,2.90830672082235));
#27373=CARTESIAN_POINT('Ctrl Pts',(-36.8783701907586,-2.57413217337487,
3.26679301273284));
#27374=CARTESIAN_POINT('Ctrl Pts',(-36.8921925295395,-1.649359153071,3.82015542390103));
#27375=CARTESIAN_POINT('Ctrl Pts',(-36.8991021422894,-1.12957504885575,
4.00475229120779));
#27376=CARTESIAN_POINT('Ctrl Pts',(-36.9116424946604,-0.0721770441526228,
4.1572862110603));
#27377=CARTESIAN_POINT('Ctrl Pts',(-36.9173352496109,0.454080222469922,
4.13304406660709));
#27378=CARTESIAN_POINT('Ctrl Pts',(-36.9304946576446,1.48451292117278,3.88597041916154));
#27379=CARTESIAN_POINT('Ctrl Pts',(-36.9374437971501,1.97770750081534,3.65967426590964));
#27380=CARTESIAN_POINT('Ctrl Pts',(-36.951214792953,2.85640483962125,3.02567766666973));
#27381=CARTESIAN_POINT('Ctrl Pts',(-36.9578387518307,3.23138713958174,2.62142868411158));
#27382=CARTESIAN_POINT('Ctrl Pts',(-36.9697812782337,3.79048149629175,1.70943238667739));
#27383=CARTESIAN_POINT('Ctrl Pts',(-36.9762051847253,3.97668136035649,1.21486817836494));
#27384=CARTESIAN_POINT('Ctrl Pts',(-36.9897773735142,4.1575446739385,0.162549653208822));
#27385=CARTESIAN_POINT('Ctrl Pts',(-36.9968110603857,4.14272189801142,-0.386597455608169));
#27386=CARTESIAN_POINT('Ctrl Pts',(-37.0101893544228,3.90287712781141,-1.43848358748678));
#27387=CARTESIAN_POINT('Ctrl Pts',(-37.01597459825,3.68368772343865,-1.93187128553373));
#27388=CARTESIAN_POINT('Ctrl Pts',(-37.028550762786,3.07216024767993,-2.8032152880964));
#27389=CARTESIAN_POINT('Ctrl Pts',(-37.0352601979701,2.68720264144112,-3.174132919078));
#27390=CARTESIAN_POINT('Ctrl Pts',(-37.0491201402536,1.78028797106041,-3.76160625531938));
#27391=CARTESIAN_POINT('Ctrl Pts',(-37.0561382455587,1.26257554819493,-3.96547809484026));
#27392=CARTESIAN_POINT('Ctrl Pts',(-37.0655724171135,0.481878270195129,
-4.10389697683738));
#27393=CARTESIAN_POINT('Ctrl Pts',(-37.0682618379416,0.240902090955855,
-4.12499999999999));
#27394=CARTESIAN_POINT('Ctrl Pts',(-37.0709904640031,3.27860210979314E-14,
-4.12499999999999));
#27395=CARTESIAN_POINT('Ctrl Pts',(-36.9916154631359,3.30485893395059E-14,
-4.12499999999999));
#27396=CARTESIAN_POINT('Ctrl Pts',(-36.9893305241456,0.201730309719417,
-4.12499999999999));
#27397=CARTESIAN_POINT('Ctrl Pts',(-36.9870917054975,0.403614853428467,
-4.11020203186251));
#27398=CARTESIAN_POINT('Ctrl Pts',(-36.978287832153,1.14435371916495,-4.0005551310462));
#27399=CARTESIAN_POINT('Ctrl Pts',(-36.971372561439,1.66345805077401,-3.81403809622079));
#27400=CARTESIAN_POINT('Ctrl Pts',(-36.9575516705327,2.58602406242228,-3.2573567197015));
#27401=CARTESIAN_POINT('Ctrl Pts',(-36.9507801515451,2.9836343999844,-2.89755497283861));
#27402=CARTESIAN_POINT('Ctrl Pts',(-36.9380758561353,3.62016474349483,-2.04737547667693));
#27403=CARTESIAN_POINT('Ctrl Pts',(-36.932415069113,3.85329630924313,-1.56507123600717));
#27404=CARTESIAN_POINT('Ctrl Pts',(-36.9191912398441,4.12783254379462,-0.524021945356768));
#27405=CARTESIAN_POINT('Ctrl Pts',(-36.9121516713196,4.16087846414009,0.0262203002124799));
#27406=CARTESIAN_POINT('Ctrl Pts',(-36.8984829167639,4.01366219794949,1.08724596219465));
#27407=CARTESIAN_POINT('Ctrl Pts',(-36.8919731779874,3.84272750092134,1.58903818341369));
#27408=CARTESIAN_POINT('Ctrl Pts',(-36.8797636626523,3.30962575391587,2.52276737198302));
#27409=CARTESIAN_POINT('Ctrl Pts',(-36.8733447064144,2.94424120069034,2.94099241861182));
#27410=CARTESIAN_POINT('Ctrl Pts',(-36.8595653478843,2.07966474064219,3.60293510571031));
#27411=CARTESIAN_POINT('Ctrl Pts',(-36.8525879158149,1.59159286110859,3.84356345624947));
#27412=CARTESIAN_POINT('Ctrl Pts',(-36.8393282713374,0.567367275551635,
4.11895460724689));
#27413=CARTESIAN_POINT('Ctrl Pts',(-36.8335175660888,0.0425157025061008,
4.1576289332339));
#27414=CARTESIAN_POINT('Ctrl Pts',(-36.8211418984236,-1.01813030924982,
4.03451853867593));
#27415=CARTESIAN_POINT('Ctrl Pts',(-36.814277838969,-1.5427859224169,3.86441874539541));
#27416=CARTESIAN_POINT('Ctrl Pts',(-36.8004506839492,-2.48374759460356,
3.33625510922713));
#27417=CARTESIAN_POINT('Ctrl Pts',(-36.7936240883164,-2.89352715898268,
2.98782625208009));
#27418=CARTESIAN_POINT('Ctrl Pts',(-36.7807967698813,-3.55446914547999,
2.15861648518414));
#27419=CARTESIAN_POINT('Ctrl Pts',(-36.7752031580768,-3.80110005427536,
1.68686532625811));
#27420=CARTESIAN_POINT('Ctrl Pts',(-36.7621343912782,-4.10904539493212,
0.656744278712707));
#27421=CARTESIAN_POINT('Ctrl Pts',(-36.7550963066766,-4.15984699262744,
0.105997737615902));
#27422=CARTESIAN_POINT('Ctrl Pts',(-36.7413469502353,-4.04560200847876,
-0.962466275870112));
#27423=CARTESIAN_POINT('Ctrl Pts',(-36.7347598186218,-3.88972121826326,
-1.47082085340387));
#27424=CARTESIAN_POINT('Ctrl Pts',(-36.7224143915539,-3.38720824987418,
-2.41621937772741));
#27425=CARTESIAN_POINT('Ctrl Pts',(-36.7162753541536,-3.03955768836155,
-2.8411958316692));
#27426=CARTESIAN_POINT('Ctrl Pts',(-36.7026374066437,-2.20172182822143,
-3.52994987558751));
#27427=CARTESIAN_POINT('Ctrl Pts',(-36.6956325634038,-1.72044144332667,
-3.78790261969301));
#27428=CARTESIAN_POINT('Ctrl Pts',(-36.6836820048752,-0.812559101531468,
-4.06473822366178));
#27429=CARTESIAN_POINT('Ctrl Pts',(-36.6787262751517,-0.407074560825465,
-4.12499999999999));
#27430=CARTESIAN_POINT('Ctrl Pts',(-36.6741154631359,2.99760216648792E-14,
-4.12499999999999));
#27431=CARTESIAN_POINT('Origin',(-44.,0.,0.));
#27432=CARTESIAN_POINT('',(-36.3566154631359,-2.34370863720154E-13,-4.12499999999999));
#27433=CARTESIAN_POINT('',(-36.4359904640031,-7.73000445117183E-16,-4.12499999999999));
#27434=CARTESIAN_POINT('',(-44.,-5.05166804648282E-16,-4.12499999999999));
#27435=CARTESIAN_POINT('Ctrl Pts',(-36.4359904640031,4.01068067645838E-14,
-4.12499999999999));
#27436=CARTESIAN_POINT('Ctrl Pts',(-36.4412017256467,-0.460086431121445,
-4.12499999999999));
#27437=CARTESIAN_POINT('Ctrl Pts',(-36.4468453199935,-0.917411502442056,
-4.04802055218068));
#27438=CARTESIAN_POINT('Ctrl Pts',(-36.4595704341114,-1.86580400053964,
-3.71876346043056));
#27439=CARTESIAN_POINT('Ctrl Pts',(-36.4665970710672,-2.338559030851,-3.44115814893948));
#27440=CARTESIAN_POINT('Ctrl Pts',(-36.4800644861582,-3.14536896278283,
-2.72236864022482));
#27441=CARTESIAN_POINT('Ctrl Pts',(-36.485949637797,-3.47301484091786,-2.28971621973573));
#27442=CARTESIAN_POINT('Ctrl Pts',(-36.4984489844205,-3.9399792698403,-1.3310705459252));
#27443=CARTESIAN_POINT('Ctrl Pts',(-36.5051191044568,-4.07798290471611,
-0.815618564857166));
#27444=CARTESIAN_POINT('Ctrl Pts',(-36.5189461858771,-4.15333093926841,
0.260266329513334));
#27445=CARTESIAN_POINT('Ctrl Pts',(-36.5259735381615,-4.081707850498,0.810902849443812));
#27446=CARTESIAN_POINT('Ctrl Pts',(-36.5388549047641,-3.73497882809028,
1.82776098681841));
#27447=CARTESIAN_POINT('Ctrl Pts',(-36.5444387415108,-3.47253378202807,
2.28741933524712));
#27448=CARTESIAN_POINT('Ctrl Pts',(-36.5574082200477,-2.78283398666363,
3.09151917646995));
#27449=CARTESIAN_POINT('Ctrl Pts',(-36.5642922791827,-2.35899467458484,
3.42590079205501));
#27450=CARTESIAN_POINT('Ctrl Pts',(-36.5781089839472,-1.39730663931997,
3.91935804898285));
#27451=CARTESIAN_POINT('Ctrl Pts',(-36.5849031395274,-0.866741587975729,
4.06971768907761));
#27452=CARTESIAN_POINT('Ctrl Pts',(-36.5970520462944,0.197849486082596,
4.15315743767392));
#27453=CARTESIAN_POINT('Ctrl Pts',(-36.6030892187348,0.721064415627516,
4.09486750473588));
#27454=CARTESIAN_POINT('Ctrl Pts',(-36.6164819110651,1.73639216168081,3.78065020492605));
#27455=CARTESIAN_POINT('Ctrl Pts',(-36.6234896276959,2.21678262677909,3.52054665687627));
#27456=CARTESIAN_POINT('Ctrl Pts',(-36.6371094361076,3.05125966565257,2.82848747037175));
#27457=CARTESIAN_POINT('Ctrl Pts',(-36.6432173154938,3.39671597472361,2.40267334681509));
#27458=CARTESIAN_POINT('Ctrl Pts',(-36.655579593977,3.89538494032113,1.45582617198234));
#27459=CARTESIAN_POINT('Ctrl Pts',(-36.6621760659865,4.04935176872739,0.946676204005937));
#27460=CARTESIAN_POINT('Ctrl Pts',(-36.6759346628,4.15941921450689,-0.122654443879365));
#27461=CARTESIAN_POINT('Ctrl Pts',(-36.6829720567077,4.10637495129219,-0.673425426266464));
#27462=CARTESIAN_POINT('Ctrl Pts',(-36.6960209247928,3.79423362638182,-1.70214089576033));
#27463=CARTESIAN_POINT('Ctrl Pts',(-36.7016098851731,3.54590018167344,-2.17257548776153));
#27464=CARTESIAN_POINT('Ctrl Pts',(-36.7144526217738,2.88186875113404,-2.99910917033283));
#27465=CARTESIAN_POINT('Ctrl Pts',(-36.7212857824561,2.47056366634082,-3.34606242349329));
#27466=CARTESIAN_POINT('Ctrl Pts',(-36.7351127493689,1.52732493058807,-3.87055432509153));
#27467=CARTESIAN_POINT('Ctrl Pts',(-36.7419697976526,1.00200118391928,-4.0385535164199));
#27468=CARTESIAN_POINT('Ctrl Pts',(-36.7500661838899,0.30646783432405,-4.11647083312409));
#27469=CARTESIAN_POINT('Ctrl Pts',(-36.7517557524127,0.153152407080955,
-4.12499999999999));
#27470=CARTESIAN_POINT('Ctrl Pts',(-36.7534904640031,3.27860210979314E-14,
-4.12499999999999));
#27471=CARTESIAN_POINT('Ctrl Pts',(-36.6741154631359,3.30485893395059E-14,
-4.12499999999999));
#27472=CARTESIAN_POINT('Ctrl Pts',(-36.6728350826434,0.113040897115812,
-4.12499999999999));
#27473=CARTESIAN_POINT('Ctrl Pts',(-36.6715907614374,0.226204519412501,
-4.12035343434328));
#27474=CARTESIAN_POINT('Ctrl Pts',(-36.6640718447843,0.883457903371157,
-4.0661229212802));
#27475=CARTESIAN_POINT('Ctrl Pts',(-36.6572695230822,1.41340994548097,-3.91358099965638));
#27476=CARTESIAN_POINT('Ctrl Pts',(-36.6434507152114,2.37288000651907,-3.41626486857158));
#27477=CARTESIAN_POINT('Ctrl Pts',(-36.6365725467785,2.79519512461284,-3.08031057313625));
#27478=CARTESIAN_POINT('Ctrl Pts',(-36.6236184889273,3.48174473184279,-2.27343780744332));
#27479=CARTESIAN_POINT('Ctrl Pts',(-36.6180372476477,3.74246021380861,-1.81247249131371));
#27480=CARTESIAN_POINT('Ctrl Pts',(-36.6051351225958,4.08497041813595,-0.794142513631144));
#27481=CARTESIAN_POINT('Ctrl Pts',(-36.5981061277905,4.15431924496963,-0.243457295605664));
#27482=CARTESIAN_POINT('Ctrl Pts',(-36.584286658258,4.07471049198571,0.831685081881199));
#27483=CARTESIAN_POINT('Ctrl Pts',(-36.5776251967898,3.93474251240417,1.34639309586123));
#27484=CARTESIAN_POINT('Ctrl Pts',(-36.5651423937967,3.46390921299336,2.30361325808074));
#27485=CARTESIAN_POINT('Ctrl Pts',(-36.559233334483,3.13411712446255,2.73543703572066));
#27486=CARTESIAN_POINT('Ctrl Pts',(-36.5457470723525,2.32393538993202,3.45101453663675));
#27487=CARTESIAN_POINT('Ctrl Pts',(-36.5387222919395,1.85022107673129,3.7265074323395));
#27488=CARTESIAN_POINT('Ctrl Pts',(-36.5252271503771,0.842349818432827,
4.07175938697056));
#27489=CARTESIAN_POINT('Ctrl Pts',(-36.5189570136296,0.320209919426375,
4.14562707604677));
#27490=CARTESIAN_POINT('Ctrl Pts',(-36.5069898247318,-0.747151170852962,
4.09335153829842));
#27491=CARTESIAN_POINT('Ctrl Pts',(-36.500257283483,-1.28181952513925,3.95862221351396));
#27492=CARTESIAN_POINT('Ctrl Pts',(-36.4864624135428,-2.25887014439116,
3.49296220009469));
#27493=CARTESIAN_POINT('Ctrl Pts',(-36.4795394640567,-2.69341161756348,
3.16998673200341));
#27494=CARTESIAN_POINT('Ctrl Pts',(-36.4664615956043,-3.40548350244653,
2.38574522771969));
#27495=CARTESIAN_POINT('Ctrl Pts',(-36.4608333961484,-3.68020610078538,
1.93524645577792));
#27496=CARTESIAN_POINT('Ctrl Pts',(-36.4481009583221,-4.05669264010034,
0.928965648007552));
#27497=CARTESIAN_POINT('Ctrl Pts',(-36.4410885169197,-4.14441036663435,
0.378930143789663));
#27498=CARTESIAN_POINT('Ctrl Pts',(-36.4272136983967,-4.09929943388298,
-0.701734160415109));
#27499=CARTESIAN_POINT('Ctrl Pts',(-36.4204851386975,-3.97527863817013,
-1.22223274256081));
#27500=CARTESIAN_POINT('Ctrl Pts',(-36.407870485071,-3.53561630564112,-2.19082580413866));
#27501=CARTESIAN_POINT('Ctrl Pts',(-36.4021282742375,-3.22290591681853,
-2.62929272235258));
#27502=CARTESIAN_POINT('Ctrl Pts',(-36.3887956204897,-2.43984218321108,
-3.37036607398834));
#27503=CARTESIAN_POINT('Ctrl Pts',(-36.381759386071,-1.97406363518828,-3.66268583780771));
#27504=CARTESIAN_POINT('Ctrl Pts',(-36.3684548786441,-0.996849952972246,
-4.03394272593325));
#27505=CARTESIAN_POINT('Ctrl Pts',(-36.3622833267925,-0.500398433273007,
-4.12499999999993));
#27506=CARTESIAN_POINT('Ctrl Pts',(-36.3566154631359,-4.95853358373211E-13,
-4.12499999999999));
#27507=CARTESIAN_POINT('Origin',(-44.,0.,0.));
#27508=CARTESIAN_POINT('',(-36.0391154631359,5.89701132001364E-15,-4.12499999999999));
#27509=CARTESIAN_POINT('',(-36.118490463256,3.29787998222272E-8,-4.12499999999999));
#27510=CARTESIAN_POINT('',(-44.,-5.05166804648282E-16,-4.12499999999999));
#27511=CARTESIAN_POINT('',(-36.,2.86773946748161,-2.96507931540595));
#27512=CARTESIAN_POINT('Ctrl Pts',(-36.0391154631359,3.30485893395058E-14,
-4.12499999999999));
#27513=CARTESIAN_POINT('Ctrl Pts',(-36.0337451023778,0.474132807753825,
-4.12499999999999));
#27514=CARTESIAN_POINT('Ctrl Pts',(-36.0282440585244,0.945254618717873,
-4.0432484302357));
#27515=CARTESIAN_POINT('Ctrl Pts',(-36.0186280448279,1.66734526282084,-3.78428978927984));
#27516=CARTESIAN_POINT('Ctrl Pts',(-36.014893553752,1.93096315570308,-3.65681146633632));
#27517=CARTESIAN_POINT('Ctrl Pts',(-36.0074010648044,2.42689448492082,-3.3482992956644));
#27518=CARTESIAN_POINT('Ctrl Pts',(-36.0036641910876,2.65780272692487,-3.16812409516617));
#27519=CARTESIAN_POINT('Ctrl Pts',(-36.,2.86773946747953,-2.96507931540796));
#27520=CARTESIAN_POINT('',(-36.,2.91366312592486,2.91996441564374));
#27521=CARTESIAN_POINT('Origin',(-36.,0.,0.));
#27522=CARTESIAN_POINT('Ctrl Pts',(-36.,2.91366312592486,2.91996441564374));
#27523=CARTESIAN_POINT('Ctrl Pts',(-36.0036344485079,3.12330794772784,2.71077200783361));
#27524=CARTESIAN_POINT('Ctrl Pts',(-36.0071391686434,3.30981666374636,2.4796074816148));
#27525=CARTESIAN_POINT('Ctrl Pts',(-36.0137501146596,3.6292482539912,1.98266554537504));
#27526=CARTESIAN_POINT('Ctrl Pts',(-36.0171520191282,3.76153650954986,1.71850385079139));
#27527=CARTESIAN_POINT('Ctrl Pts',(-36.0272316267131,4.05122661578133,0.9424079233371));
#27528=CARTESIAN_POINT('Ctrl Pts',(-36.0340864334346,4.13905909688259,0.410798315377361));
#27529=CARTESIAN_POINT('Ctrl Pts',(-36.0479110832572,4.10691957881801,-0.668650461754651));
#27530=CARTESIAN_POINT('Ctrl Pts',(-36.054743369101,3.98241785588811,-1.20591830893745));
#27531=CARTESIAN_POINT('Ctrl Pts',(-36.0670127170578,3.54154333993596,-2.17832645881722));
#27532=CARTESIAN_POINT('Ctrl Pts',(-36.0729205373609,3.23803788616501,-2.60820919952761));
#27533=CARTESIAN_POINT('Ctrl Pts',(-36.0862432780018,2.47370737118609,-3.34484086675196));
#27534=CARTESIAN_POINT('Ctrl Pts',(-36.0932361557912,2.01509670145264,-3.63958423728565));
#27535=CARTESIAN_POINT('Ctrl Pts',(-36.1065821902674,1.03078125812558,-4.02759302272963));
#27536=CARTESIAN_POINT('Ctrl Pts',(-36.1126283245692,0.517550452608532,
-4.12499999586171));
#27537=CARTESIAN_POINT('Ctrl Pts',(-36.1184904636295,3.29830760293365E-8,
-4.12499999999999));
#27538=CARTESIAN_POINT('Origin',(-44.,0.,0.));
#27539=CARTESIAN_POINT('',(-44.,-5.08228421646152E-16,-4.15));
#27540=CARTESIAN_POINT('',(-44.,-5.08228421646152E-16,-4.15));
#27541=CARTESIAN_POINT('Origin',(-44.,0.,0.));
#27542=CARTESIAN_POINT('Origin',(0.,0.,0.));
#27543=CARTESIAN_POINT('',(-36.,-9.79717439317882E-16,8.));
#27544=CARTESIAN_POINT('Origin',(-36.,0.,0.));
#27545=CARTESIAN_POINT('',(-34.5,-9.79717439317882E-16,8.));
#27546=CARTESIAN_POINT('',(0.,-9.79717439317882E-16,8.));
#27547=CARTESIAN_POINT('',(-34.5,-2.47065947129021,7.60893171062298));
#27548=CARTESIAN_POINT('Origin',(-34.5,0.,0.));
#27549=CARTESIAN_POINT('',(-27.5,-2.47065947129021,7.60893171062298));
#27550=CARTESIAN_POINT('Ctrl Pts',(-27.5,-2.47065947129021,7.60893171062298));
#27551=CARTESIAN_POINT('Ctrl Pts',(-27.5082762748436,-2.53363768497578,
7.58848235898667));
#27552=CARTESIAN_POINT('Ctrl Pts',(-27.5167952547663,-2.59610030182682,
7.56728331237343));
#27553=CARTESIAN_POINT('Ctrl Pts',(-27.531909539296,-2.69176254620422,7.5336703249928));
#27554=CARTESIAN_POINT('Ctrl Pts',(-27.541703143922,-2.74920364206476,7.51311905977958));
#27555=CARTESIAN_POINT('Ctrl Pts',(-27.5886747936238,-2.94732068709103,
7.43861628862778));
#27556=CARTESIAN_POINT('Ctrl Pts',(-27.6278318406471,-3.044268769857,7.39878659172515));
#27557=CARTESIAN_POINT('Ctrl Pts',(-27.8123603858098,-3.37981144694253,
7.25589234200809));
#27558=CARTESIAN_POINT('Ctrl Pts',(-28.022658308916,-3.57168495780948,7.15984048137768));
#27559=CARTESIAN_POINT('Ctrl Pts',(-28.336993665887,-3.81265791239897,7.03423030810345));
#27560=CARTESIAN_POINT('Ctrl Pts',(-28.4851452188162,-3.89961660935025,
6.98559531051076));
#27561=CARTESIAN_POINT('Ctrl Pts',(-28.7988210742809,-4.06294287716043,
6.89241495700718));
#27562=CARTESIAN_POINT('Ctrl Pts',(-29.0017446327031,-4.14499080192856,
6.84289918755403));
#27563=CARTESIAN_POINT('Ctrl Pts',(-29.4670154464834,-4.29594038338126,
6.74941755583053));
#27564=CARTESIAN_POINT('Ctrl Pts',(-29.7360700177731,-4.35777776217867,
6.70912896172516));
#27565=CARTESIAN_POINT('Ctrl Pts',(-30.3331963799111,-4.45215289547283,
6.64696430829746));
#27566=CARTESIAN_POINT('Ctrl Pts',(-30.667122960172,-4.47714488295397,6.62986981008182));
#27567=CARTESIAN_POINT('Ctrl Pts',(-31.4223356644344,-4.47722023321691,
6.62981892557196));
#27568=CARTESIAN_POINT('Ctrl Pts',(-31.7581570009252,-4.43692246189483,
6.65701260246374));
#27569=CARTESIAN_POINT('Ctrl Pts',(-32.4245916936501,-4.33028864634714,
6.72720608258351));
#27570=CARTESIAN_POINT('Ctrl Pts',(-32.9726605932112,-4.20069539173016,
6.81615080651099));
#27571=CARTESIAN_POINT('Ctrl Pts',(-33.620923016355,-3.83675530423863,7.02052775006877));
#27572=CARTESIAN_POINT('Ctrl Pts',(-33.7554605943269,-3.74680811900599,
7.0692841494146));
#27573=CARTESIAN_POINT('Ctrl Pts',(-33.9780038810456,-3.56413110131904,
7.16275145624606));
#27574=CARTESIAN_POINT('Ctrl Pts',(-34.0686873290645,-3.47735595456888,
7.20546101456539));
#27575=CARTESIAN_POINT('Ctrl Pts',(-34.1772650516204,-3.35016875610881,
7.26482911701887));
#27576=CARTESIAN_POINT('Ctrl Pts',(-34.2047645004423,-3.31541359912121,
7.2807667169273));
#27577=CARTESIAN_POINT('Ctrl Pts',(-34.2531499977949,-3.24829608019548,
7.3109342508995));
#27578=CARTESIAN_POINT('Ctrl Pts',(-34.2735415360389,-3.21738266753306,
7.32459320987789));
#27579=CARTESIAN_POINT('Ctrl Pts',(-34.3258608593232,-3.13079515769325,
7.36217786629595));
#27580=CARTESIAN_POINT('Ctrl Pts',(-34.3543988312875,-3.07492684441128,
7.38572796575362));
#27581=CARTESIAN_POINT('Ctrl Pts',(-34.4549669946965,-2.82653092707015,
7.48680369569123));
#27582=CARTESIAN_POINT('Ctrl Pts',(-34.4789671836597,-2.62428232032289,
7.55904957717719));
#27583=CARTESIAN_POINT('Ctrl Pts',(-34.5,-2.47065947129021,7.60893171062298));
#27584=CARTESIAN_POINT('',(-27.5,-9.79717439317882E-16,8.));
#27585=CARTESIAN_POINT('Origin',(-27.5,0.,0.));
#27586=CARTESIAN_POINT('',(-20.,-9.79717439317882E-16,8.));
#27587=CARTESIAN_POINT('',(0.,-9.79717439317882E-16,8.));
#27588=CARTESIAN_POINT('Origin',(-20.,0.,0.));
#27589=CARTESIAN_POINT('',(-27.5,6.19655913866284,5.0599066039853));
#27590=CARTESIAN_POINT('Origin',(-27.5,0.,0.));
#27591=CARTESIAN_POINT('',(-34.5,6.19655913866284,5.0599066039853));
#27592=CARTESIAN_POINT('Ctrl Pts',(-34.5,6.19655913866284,5.0599066039853));
#27593=CARTESIAN_POINT('Ctrl Pts',(-34.4917237251617,6.23843937773582,5.00861842843821));
#27594=CARTESIAN_POINT('Ctrl Pts',(-34.4832047452396,6.27948024728051,4.95697905290007));
#27595=CARTESIAN_POINT('Ctrl Pts',(-34.4680904607238,6.34171420244266,4.87692886408564));
#27596=CARTESIAN_POINT('Ctrl Pts',(-34.4582968560933,6.37888375730234,4.82855264885907));
#27597=CARTESIAN_POINT('Ctrl Pts',(-34.4113252064685,6.50512326594944,4.65865676098275));
#27598=CARTESIAN_POINT('Ctrl Pts',(-34.3721681594988,6.56507277118939,4.57268355368093));
#27599=CARTESIAN_POINT('Ctrl Pts',(-34.1876396142192,6.76983200977991,4.27088675275452));
#27600=CARTESIAN_POINT('Ctrl Pts',(-33.9773416916577,6.87915596409205,4.08625285297235));
#27601=CARTESIAN_POINT('Ctrl Pts',(-33.6630063342077,7.01375978486032,3.85018571820814));
#27602=CARTESIAN_POINT('Ctrl Pts',(-33.5148547815411,7.06054343608664,3.76221715605519));
#27603=CARTESIAN_POINT('Ctrl Pts',(-33.2011789257173,7.14741992935041,3.59545228256026));
#27604=CARTESIAN_POINT('Ctrl Pts',(-32.9982553672152,7.1895978636344,3.5094017436486));
#27605=CARTESIAN_POINT('Ctrl Pts',(-32.5329845533841,7.2659051532144,3.34908396804489));
#27606=CARTESIAN_POINT('Ctrl Pts',(-32.2639299821026,7.29608576292504,3.28173292478837));
#27607=CARTESIAN_POINT('Ctrl Pts',(-31.6668036200137,7.34178042907256,3.1783738061678));
#27608=CARTESIAN_POINT('Ctrl Pts',(-31.332877039813,7.35353874703556,3.15047105961028));
#27609=CARTESIAN_POINT('Ctrl Pts',(-30.5776643347629,7.353574552694,3.15038748419466));
#27610=CARTESIAN_POINT('Ctrl Pts',(-30.2418429982892,7.33441482688859,3.1950675844706));
#27611=CARTESIAN_POINT('Ctrl Pts',(-29.5754083083462,7.28275986922452,3.31181372141937));
#27612=CARTESIAN_POINT('Ctrl Pts',(-29.02733940778,7.22195244224698,3.45675520013408));
#27613=CARTESIAN_POINT('Ctrl Pts',(-28.3790769835261,7.02660224834134,3.82561916527211));
#27614=CARTESIAN_POINT('Ctrl Pts',(-28.2445394054004,6.97737165243015,3.91530768774012));
#27615=CARTESIAN_POINT('Ctrl Pts',(-28.0219961187517,6.87438073889736,4.09278980501267));
#27616=CARTESIAN_POINT('Ctrl Pts',(-27.9313126708239,6.82454353901441,4.17567699316933));
#27617=CARTESIAN_POINT('Ctrl Pts',(-27.8227349483168,6.74974708920182,4.29444839597648));
#27618=CARTESIAN_POINT('Ctrl Pts',(-27.7952354994949,6.72915375666957,4.32666396183648));
#27619=CARTESIAN_POINT('Ctrl Pts',(-27.7468500021218,6.68905442683588,4.3883639229692));
#27620=CARTESIAN_POINT('Ctrl Pts',(-27.7264584638972,6.67045756991583,4.41658383000757));
#27621=CARTESIAN_POINT('Ctrl Pts',(-27.6741391406086,6.61800364689995,4.49506050949652));
#27622=CARTESIAN_POINT('Ctrl Pts',(-27.6456011686512,6.58377994863887,4.54510662916641));
#27623=CARTESIAN_POINT('Ctrl Pts',(-27.5450330043088,6.4296527386651,4.76456423198599));
#27624=CARTESIAN_POINT('Ctrl Pts',(-27.5210328155748,6.29871766361913,4.93479928660682));
#27625=CARTESIAN_POINT('Ctrl Pts',(-27.5,6.19655913866284,5.0599066039853));
#27626=CARTESIAN_POINT('Origin',(-34.5,0.,0.));
#27627=CARTESIAN_POINT('Origin',(-43.,0.,0.));
#27628=CARTESIAN_POINT('',(-43.,-1.53080849893419E-15,12.5));
#27629=CARTESIAN_POINT('Origin',(-43.,0.,0.));
#27630=CARTESIAN_POINT('',(-44.,-1.40834381901945E-15,11.5));
#27631=CARTESIAN_POINT('Origin',(-43.,-1.40834381901945E-15,11.5));
#27632=CARTESIAN_POINT('Origin',(-44.,0.,0.));
#27633=CARTESIAN_POINT('Origin',(0.,0.,0.));
#27634=CARTESIAN_POINT('',(-25.,-1.53080849893419E-15,12.5));
#27635=CARTESIAN_POINT('Origin',(-25.,0.,0.));
#27636=CARTESIAN_POINT('',(-27.5,-1.53080849893419E-15,12.5));
#27637=CARTESIAN_POINT('',(0.,-1.53080849893419E-15,12.5));
#27638=CARTESIAN_POINT('',(-27.5,-3.86040542389096,11.8889557978484));
#27639=CARTESIAN_POINT('Origin',(-27.5,0.,0.));
#27640=CARTESIAN_POINT('',(-34.5,-3.86040542389096,11.8889557978484));
#27641=CARTESIAN_POINT('Ctrl Pts',(-34.5,-3.86040542389096,11.8889557978484));
#27642=CARTESIAN_POINT('Ctrl Pts',(-34.494970655399,-3.91780250120729,11.8703186700506));
#27643=CARTESIAN_POINT('Ctrl Pts',(-34.4903159600402,-3.96935886536347,
11.8531231208353));
#27644=CARTESIAN_POINT('Ctrl Pts',(-34.4860358608515,-4.01514468999518,
11.8375932147715));
#27645=CARTESIAN_POINT('Ctrl Pts',(-34.4848922703583,-4.02737810596607,
11.8334438125843));
#27646=CARTESIAN_POINT('Ctrl Pts',(-34.4837754220408,-4.03919950769951,
11.8294130376282));
#27647=CARTESIAN_POINT('Ctrl Pts',(-34.4826853148868,-4.05061009613366,
11.8255045494516));
#27648=CARTESIAN_POINT('Ctrl Pts',(-34.4801002973656,-4.07766851045364,
11.8162361849796));
#27649=CARTESIAN_POINT('Ctrl Pts',(-34.4776656615101,-4.10241686090276,
11.8076560597129));
#27650=CARTESIAN_POINT('Ctrl Pts',(-34.4753814073201,-4.1248695117463,11.799807265844));
#27651=CARTESIAN_POINT('Ctrl Pts',(-34.4742392802251,-4.13609583716807,
11.7958828689096));
#27652=CARTESIAN_POINT('Ctrl Pts',(-34.4731347485465,-4.14674820379434,
11.7921411785115));
#27653=CARTESIAN_POINT('Ctrl Pts',(-34.4720678122842,-4.15682819390705,
11.7885868265174));
#27654=CARTESIAN_POINT('Ctrl Pts',(-34.4713134278961,-4.1639553180311,11.7860736982743));
#27655=CARTESIAN_POINT('Ctrl Pts',(-34.47090989401,-4.16780274964417,11.784713577999));
#27656=CARTESIAN_POINT('Ctrl Pts',(-34.4701528645571,-4.17472128216715,
11.7822621858547));
#27657=CARTESIAN_POINT('Ctrl Pts',(-34.4698392167961,-4.17758772577372,
11.7812465402223));
#27658=CARTESIAN_POINT('Ctrl Pts',(-34.4694648894221,-4.1809812090102,11.7800431939136));
#27659=CARTESIAN_POINT('Ctrl Pts',(-34.4689797897467,-4.18535246715401,
11.7784899170347));
#27660=CARTESIAN_POINT('Ctrl Pts',(-34.4623559877182,-4.24503988817323,
11.7572806706389));
#27661=CARTESIAN_POINT('Ctrl Pts',(-34.4552691208995,-4.3014092606901,11.73674089348));
#27662=CARTESIAN_POINT('Ctrl Pts',(-34.4477191892904,-4.35450417596821,
11.7170087215755));
#27663=CARTESIAN_POINT('Ctrl Pts',(-34.4439442234859,-4.38105163360727,
11.7071426356232));
#27664=CARTESIAN_POINT('Ctrl Pts',(-34.4400534914838,-4.40678045394109,
11.6974781922229));
#27665=CARTESIAN_POINT('Ctrl Pts',(-34.4360469932842,-4.43169590229857,
11.688031118608));
#27666=CARTESIAN_POINT('Ctrl Pts',(-34.4336061624609,-4.44687484193522,
11.6822757913073));
#27667=CARTESIAN_POINT('Ctrl Pts',(-34.4314324547114,-4.46004496983625,
11.6772527958857));
#27668=CARTESIAN_POINT('Ctrl Pts',(-34.4289591340832,-4.4743282340168,11.6717773648352));
#27669=CARTESIAN_POINT('Ctrl Pts',(-34.4273726261688,-4.48349021302091,
11.6682651575633));
#27670=CARTESIAN_POINT('Ctrl Pts',(-34.4256628406678,-4.49310990046616,
11.6645659967412));
#27671=CARTESIAN_POINT('Ctrl Pts',(-34.4236802000926,-4.50400723835645,
11.6603567182498));
#27672=CARTESIAN_POINT('Ctrl Pts',(-34.4154020416518,-4.54950710896653,
11.6427816344403));
#27673=CARTESIAN_POINT('Ctrl Pts',(-34.406653472996,-4.59275567416098,11.6257749226861));
#27674=CARTESIAN_POINT('Ctrl Pts',(-34.3971295455735,-4.63477689237434,
11.60899837014));
#27675=CARTESIAN_POINT('Ctrl Pts',(-34.3873134488299,-4.67808721226327,
11.5917071565984));
#27676=CARTESIAN_POINT('Ctrl Pts',(-34.3766736916467,-4.72009374737927,
11.5746602240549));
#27677=CARTESIAN_POINT('Ctrl Pts',(-34.3648763906193,-4.76189818145385,
11.5574359487503));
#27678=CARTESIAN_POINT('Ctrl Pts',(-34.3600593412814,-4.77896768074119,
11.5504029686001));
#27679=CARTESIAN_POINT('Ctrl Pts',(-34.3550493021611,-4.79600326253241,
11.5433398564416));
#27680=CARTESIAN_POINT('Ctrl Pts',(-34.3498235437455,-4.81307899502436,
11.5362156094473));
#27681=CARTESIAN_POINT('Ctrl Pts',(-34.3365616064945,-4.85641381359207,
11.5181356851409));
#27682=CARTESIAN_POINT('Ctrl Pts',(-34.3215920418828,-4.90045195053886,
11.49947096044));
#27683=CARTESIAN_POINT('Ctrl Pts',(-34.3053895006549,-4.94413101835602,
11.4806606287848));
#27684=CARTESIAN_POINT('Ctrl Pts',(-34.2889938068611,-4.98833078992604,
11.4616260567607));
#27685=CARTESIAN_POINT('Ctrl Pts',(-34.2713355642849,-5.03216278653615,
11.4424424259165));
#27686=CARTESIAN_POINT('Ctrl Pts',(-34.2529066019543,-5.07454774569108,
11.4236143657208));
#27687=CARTESIAN_POINT('Ctrl Pts',(-34.2477440704824,-5.0864211046815,11.4183400343953));
#27688=CARTESIAN_POINT('Ctrl Pts',(-34.2425210578452,-5.0981810411742,11.4130938957045));
#27689=CARTESIAN_POINT('Ctrl Pts',(-34.2372483758835,-5.10980413280796,
11.407887697744));
#27690=CARTESIAN_POINT('Ctrl Pts',(-34.2060970380929,-5.17847409171857,
11.3771291516276));
#27691=CARTESIAN_POINT('Ctrl Pts',(-34.1713309554745,-5.24692483123779,
11.3457195635697));
#27692=CARTESIAN_POINT('Ctrl Pts',(-34.1334397960299,-5.31449179121027,
11.3139814831543));
#27693=CARTESIAN_POINT('Ctrl Pts',(-34.0948626907383,-5.38328191975986,
11.2816688464369));
#27694=CARTESIAN_POINT('Ctrl Pts',(-34.0530463375756,-5.45115583394936,
11.2490157906367));
#27695=CARTESIAN_POINT('Ctrl Pts',(-34.0085074823357,-5.51743673946892,
11.2164117179229));
#27696=CARTESIAN_POINT('Ctrl Pts',(-33.9768762953056,-5.56450898027351,
11.1932565309205));
#27697=CARTESIAN_POINT('Ctrl Pts',(-33.9438719484171,-5.61077827891772,
11.1701271129436));
#27698=CARTESIAN_POINT('Ctrl Pts',(-33.9096795416066,-5.65600990849816,
11.1471768585131));
#27699=CARTESIAN_POINT('Ctrl Pts',(-33.8448661510052,-5.74174868938547,
11.1036735212649));
#27700=CARTESIAN_POINT('Ctrl Pts',(-33.7764476368752,-5.82327304054431,
11.0610704051755));
#27701=CARTESIAN_POINT('Ctrl Pts',(-33.7039936885002,-5.90106683527327,
11.0194106106288));
#27702=CARTESIAN_POINT('Ctrl Pts',(-33.6315397401253,-5.97886063000223,
10.977750816082));
#27703=CARTESIAN_POINT('Ctrl Pts',(-33.5550503575055,-6.05292387508725,
10.9370337816686));
#27704=CARTESIAN_POINT('Ctrl Pts',(-33.4740952299247,-6.12372280736542,
10.8972482296474));
#27705=CARTESIAN_POINT('Ctrl Pts',(-33.3673080229709,-6.21711306514419,
10.8447674528959));
#27706=CARTESIAN_POINT('Ctrl Pts',(-33.2534811611839,-6.30331921585543,
10.7947479660883));
#27707=CARTESIAN_POINT('Ctrl Pts',(-33.1337150622316,-6.38220287634025,
10.7479061423718));
#27708=CARTESIAN_POINT('Ctrl Pts',(-33.0200172364479,-6.45708968291937,
10.703437686282));
#27709=CARTESIAN_POINT('Ctrl Pts',(-32.9009667812065,-6.52537806498607,
10.6618332745438));
#27710=CARTESIAN_POINT('Ctrl Pts',(-32.777505179161,-6.58694495509603,10.6236602053405));
#27711=CARTESIAN_POINT('Ctrl Pts',(-32.6598228499643,-6.64562988149819,
10.5872740284077));
#27712=CARTESIAN_POINT('Ctrl Pts',(-32.5381326823293,-6.69820844752292,
10.5540056089092));
#27713=CARTESIAN_POINT('Ctrl Pts',(-32.4132500380636,-6.74455973963733,
10.5243011130651));
#27714=CARTESIAN_POINT('Ctrl Pts',(-32.2959024600774,-6.78811432560992,
10.4963889026607));
#27715=CARTESIAN_POINT('Ctrl Pts',(-32.1757360330685,-6.82617076458576,
10.4716234758828));
#27716=CARTESIAN_POINT('Ctrl Pts',(-32.0534272550074,-6.85860954795537,
10.4503337300153));
#27717=CARTESIAN_POINT('Ctrl Pts',(-31.934697526644,-6.89009909432292,10.4296669734354));
#27718=CARTESIAN_POINT('Ctrl Pts',(-31.8139489934702,-6.91629525531148,
10.4122756081045));
#27719=CARTESIAN_POINT('Ctrl Pts',(-31.691800486454,-6.93706541972051,10.3984192722989));
#27720=CARTESIAN_POINT('Ctrl Pts',(-31.5747340084618,-6.95697143457143,
10.3851394339263));
#27721=CARTESIAN_POINT('Ctrl Pts',(-31.4563816260168,-6.97189371437512,
10.3751066275311));
#27722=CARTESIAN_POINT('Ctrl Pts',(-31.3372880991137,-6.98169062285308,
10.3685098276833));
#27723=CARTESIAN_POINT('Ctrl Pts',(-31.2253150028751,-6.99090178826543,
10.3623074410093));
#27724=CARTESIAN_POINT('Ctrl Pts',(-31.1126867367521,-6.9955821236098,10.3591423753097));
#27725=CARTESIAN_POINT('Ctrl Pts',(-30.9998560750767,-6.99559063859199,
10.3591366250882));
#27726=CARTESIAN_POINT('Ctrl Pts',(-30.8797994738452,-6.99559969889357,
10.3591305066091));
#27727=CARTESIAN_POINT('Ctrl Pts',(-30.7600926671373,-6.99048466724076,
10.3625901353736));
#27728=CARTESIAN_POINT('Ctrl Pts',(-30.6411870533517,-6.98031808007771,
10.3694339045553));
#27729=CARTESIAN_POINT('Ctrl Pts',(-30.5209337732766,-6.97003626566538,
10.3763552404449));
#27730=CARTESIAN_POINT('Ctrl Pts',(-30.4014999503503,-6.95458763079492,
10.3867377989898));
#27731=CARTESIAN_POINT('Ctrl Pts',(-30.2833525059205,-6.93401732448088,
10.4004520932409));
#27732=CARTESIAN_POINT('Ctrl Pts',(-30.1629637338705,-6.91305678716422,
10.414426555849));
#27733=CARTESIAN_POINT('Ctrl Pts',(-30.043910610001,-6.88677828371061,10.4318603772502));
#27734=CARTESIAN_POINT('Ctrl Pts',(-29.9266871362902,-6.85520048168457,
10.4525703229355));
#27735=CARTESIAN_POINT('Ctrl Pts',(-29.8368473729342,-6.8309993368838,10.4684423710892));
#27736=CARTESIAN_POINT('Ctrl Pts',(-29.7480822819468,-6.80368493907954,
10.4862377470792));
#27737=CARTESIAN_POINT('Ctrl Pts',(-29.6606142407677,-6.77325535385644,
10.5058560770389));
#27738=CARTESIAN_POINT('Ctrl Pts',(-29.5206149476823,-6.72455047419196,
10.5372567153617));
#27739=CARTESIAN_POINT('Ctrl Pts',(-29.3844295684138,-6.66785803981784,
10.57333373119));
#27740=CARTESIAN_POINT('Ctrl Pts',(-29.2532397481725,-6.60365955267175,
10.61327849971));
#27741=CARTESIAN_POINT('Ctrl Pts',(-29.1018107116331,-6.52955688953876,
10.6593857190099));
#27742=CARTESIAN_POINT('Ctrl Pts',(-28.9570375038436,-6.44545120919904,
10.710644896099));
#27743=CARTESIAN_POINT('Ctrl Pts',(-28.8207373726615,-6.35207155220489,
10.7657413583863));
#27744=CARTESIAN_POINT('Ctrl Pts',(-28.7172009582184,-6.28113842262358,
10.8075937770468));
#27745=CARTESIAN_POINT('Ctrl Pts',(-28.6185537102732,-6.2048534694645,10.8516584751742));
#27746=CARTESIAN_POINT('Ctrl Pts',(-28.525592163538,-6.1235467477601,10.8973471647001));
#27747=CARTESIAN_POINT('Ctrl Pts',(-28.4641697382623,-6.06982500781815,
10.9275350242712));
#27748=CARTESIAN_POINT('Ctrl Pts',(-28.4054615364755,-6.01445977844525,
10.9581285073625));
#27749=CARTESIAN_POINT('Ctrl Pts',(-28.3489685850519,-5.95676427999888,
10.9894021362643));
#27750=CARTESIAN_POINT('Ctrl Pts',(-28.2950240546477,-5.9016714499785,11.019264998491));
#27751=CARTESIAN_POINT('Ctrl Pts',(-28.2430994207628,-5.84445379489708,
11.0497481752732));
#27752=CARTESIAN_POINT('Ctrl Pts',(-28.192760236588,-5.78449380851062,11.0810482978508));
#27753=CARTESIAN_POINT('Ctrl Pts',(-28.1579080059993,-5.74298063530583,
11.1027188733162));
#27754=CARTESIAN_POINT('Ctrl Pts',(-28.1238157538695,-5.70015254261527,
11.1247802072868));
#27755=CARTESIAN_POINT('Ctrl Pts',(-28.0903392986022,-5.65579883898769,
11.1472839513895));
#27756=CARTESIAN_POINT('Ctrl Pts',(-28.0241068899402,-5.56804604076333,
11.1918070994926));
#27757=CARTESIAN_POINT('Ctrl Pts',(-27.9636909773592,-5.47865680552519,
11.2358577237503));
#27758=CARTESIAN_POINT('Ctrl Pts',(-27.9090915608592,-5.38761723205833,
11.2793430908377));
#27759=CARTESIAN_POINT('Ctrl Pts',(-27.8843690560396,-5.34639469822763,
11.2990331766722));
#27760=CARTESIAN_POINT('Ctrl Pts',(-27.8612040828302,-5.30562818737182,
11.318232711205));
#27761=CARTESIAN_POINT('Ctrl Pts',(-27.8391008292385,-5.26424125835,11.3374496238742));
#27762=CARTESIAN_POINT('Ctrl Pts',(-27.8174064239111,-5.22361987156048,
11.3563110774994));
#27763=CARTESIAN_POINT('Ctrl Pts',(-27.7967348237883,-5.18240074233437,
11.3751893510415));
#27764=CARTESIAN_POINT('Ctrl Pts',(-27.7766172244931,-5.1395454600324,11.3945194047077));
#27765=CARTESIAN_POINT('Ctrl Pts',(-27.77196471905,-5.12963451433504,11.3989897780648));
#27766=CARTESIAN_POINT('Ctrl Pts',(-27.7673418436229,-5.11963597385404,
11.4034841144338));
#27767=CARTESIAN_POINT('Ctrl Pts',(-27.7627427996022,-5.10953683452028,
11.4080074218367));
#27768=CARTESIAN_POINT('Ctrl Pts',(-27.7433129351307,-5.06687037869769,
11.4271173171552));
#27769=CARTESIAN_POINT('Ctrl Pts',(-27.7249399287126,-5.0232704538905,11.4463531880018));
#27770=CARTESIAN_POINT('Ctrl Pts',(-27.7079530152698,-4.97978848766015,
11.4652390563026));
#27771=CARTESIAN_POINT('Ctrl Pts',(-27.6907728782746,-4.93581192068873,
11.484339748478));
#27772=CARTESIAN_POINT('Ctrl Pts',(-27.6750105467902,-4.89195610261451,
11.5030823858444));
#27773=CARTESIAN_POINT('Ctrl Pts',(-27.6610066190104,-4.84933007757205,
11.5210241644897));
#27774=CARTESIAN_POINT('Ctrl Pts',(-27.6569688649967,-4.83703971115383,
11.5261973194701));
#27775=CARTESIAN_POINT('Ctrl Pts',(-27.6530772945585,-4.82485171033533,
11.5313042061676));
#27776=CARTESIAN_POINT('Ctrl Pts',(-27.6493400718713,-4.81279295543508,
11.5363349452118));
#27777=CARTESIAN_POINT('Ctrl Pts',(-27.6345827386579,-4.76517602727854,
11.5562000425308));
#27778=CARTESIAN_POINT('Ctrl Pts',(-27.6209916578288,-4.715632537521,11.5765232413219));
#27779=CARTESIAN_POINT('Ctrl Pts',(-27.6085668293839,-4.664138015756,11.5972331428656));
#27780=CARTESIAN_POINT('Ctrl Pts',(-27.6023544151614,-4.63839075487349,
11.6075880936374));
#27781=CARTESIAN_POINT('Ctrl Pts',(-27.596433564035,-4.61215573118547,11.6180396300778));
#27782=CARTESIAN_POINT('Ctrl Pts',(-27.5908042760046,-4.5854298718991,11.6285782832595));
#27783=CARTESIAN_POINT('Ctrl Pts',(-27.5873939612376,-4.56923890918867,
11.6349627717377));
#27784=CARTESIAN_POINT('Ctrl Pts',(-27.5837940741683,-4.5512419425587,11.642015449446));
#27785=CARTESIAN_POINT('Ctrl Pts',(-27.5805436336287,-4.53439193817792,
11.6485745802217));
#27786=CARTESIAN_POINT('Ctrl Pts',(-27.5784286849673,-4.52342822609788,
11.652842378597));
#27787=CARTESIAN_POINT('Ctrl Pts',(-27.5764616798231,-4.51295056810901,
11.6569024137903));
#27788=CARTESIAN_POINT('Ctrl Pts',(-27.5747911012017,-4.50377671744548,
11.6604457581773));
#27789=CARTESIAN_POINT('Ctrl Pts',(-27.566314957399,-4.45723064265866,11.6784238983155));
#27790=CARTESIAN_POINT('Ctrl Pts',(-27.5583409045667,-4.40744011781925,
11.6973363546891));
#27791=CARTESIAN_POINT('Ctrl Pts',(-27.5508689427049,-4.3543635178157,11.717060994751));
#27792=CARTESIAN_POINT('Ctrl Pts',(-27.5471329617739,-4.32782521781393,
11.726923314782));
#27793=CARTESIAN_POINT('Ctrl Pts',(-27.5435225035856,-4.300465355621,11.7369884258351));
#27794=CARTESIAN_POINT('Ctrl Pts',(-27.5400375681399,-4.27227851169748,
11.7472395190737));
#27795=CARTESIAN_POINT('Ctrl Pts',(-27.538295100417,-4.25818508973572,11.7523650656931));
#27796=CARTESIAN_POINT('Ctrl Pts',(-27.5365840133798,-4.24388492044556,
11.7575370916891));
#27797=CARTESIAN_POINT('Ctrl Pts',(-27.5349043070283,-4.22937731649073,
11.7627533985353));
#27798=CARTESIAN_POINT('Ctrl Pts',(-27.533779193636,-4.21965972538717,11.7662474239554));
#27799=CARTESIAN_POINT('Ctrl Pts',(-27.5323768483603,-4.20716236796442,
11.7707219324888));
#27800=CARTESIAN_POINT('Ctrl Pts',(-27.5312826563378,-4.19728311588018,
11.7742436888807));
#27801=CARTESIAN_POINT('Ctrl Pts',(-27.5307433051967,-4.19241341680146,
11.7759796395084));
#27802=CARTESIAN_POINT('Ctrl Pts',(-27.5302788266484,-4.18818021743347,
11.7774851415309));
#27803=CARTESIAN_POINT('Ctrl Pts',(-27.5299593300305,-4.1852315079248,11.7785328978219));
#27804=CARTESIAN_POINT('Ctrl Pts',(-27.5269020793694,-4.15701542177606,
11.788558836859));
#27805=CARTESIAN_POINT('Ctrl Pts',(-27.5234947220653,-4.12310099413958,
11.8004999619284));
#27806=CARTESIAN_POINT('Ctrl Pts',(-27.5197371907049,-4.08343722589056,
11.8142092592865));
#27807=CARTESIAN_POINT('Ctrl Pts',(-27.5159831432012,-4.04381023255444,
11.8279058458449));
#27808=CARTESIAN_POINT('Ctrl Pts',(-27.5118795706794,-3.99844438731281,
11.8433673740677));
#27809=CARTESIAN_POINT('Ctrl Pts',(-27.5074264059136,-3.94727538011812,
11.8603970031999));
#27810=CARTESIAN_POINT('Ctrl Pts',(-27.5050504578766,-3.91997459324096,
11.8694830164142));
#27811=CARTESIAN_POINT('Ctrl Pts',(-27.5025749926422,-3.89102162637507,
11.8790145585892));
#27812=CARTESIAN_POINT('Ctrl Pts',(-27.5,-3.86040542389096,11.8889557978484));
#27813=CARTESIAN_POINT('',(-34.5,-1.53080849893419E-15,12.5));
#27814=CARTESIAN_POINT('Origin',(-34.5,0.,0.));
#27815=CARTESIAN_POINT('',(0.,-1.53080849893419E-15,12.5));
#27816=CARTESIAN_POINT('',(-34.5,9.68212365416069,7.90610406872703));
#27817=CARTESIAN_POINT('Origin',(-34.5,0.,0.));
#27818=CARTESIAN_POINT('',(-27.5,9.68212365416069,7.90610406872703));
#27819=CARTESIAN_POINT('Ctrl Pts',(-27.5,9.68212365416069,7.90610406872703));
#27820=CARTESIAN_POINT('Ctrl Pts',(-27.5050293446173,9.72029246189198,7.85936105687521));
#27821=CARTESIAN_POINT('Ctrl Pts',(-27.509684039994,9.75433093310758,7.8169921048418));
#27822=CARTESIAN_POINT('Ctrl Pts',(-27.5139641392024,9.78441937113138,7.77914761203495));
#27823=CARTESIAN_POINT('Ctrl Pts',(-27.5151077296653,9.79245863589893,7.76903602374222));
#27824=CARTESIAN_POINT('Ctrl Pts',(-27.5162245779542,9.80021570799085,7.75924722860733));
#27825=CARTESIAN_POINT('Ctrl Pts',(-27.5173146850816,9.80769357831618,7.74978365335804));
#27826=CARTESIAN_POINT('Ctrl Pts',(-27.5198997026027,9.82542617112911,7.72734227377413));
#27827=CARTESIAN_POINT('Ctrl Pts',(-27.5223343384609,9.84158909730558,7.70673016037892));
#27828=CARTESIAN_POINT('Ctrl Pts',(-27.5246185926562,9.85621776302709,7.68797576789816));
#27829=CARTESIAN_POINT('Ctrl Pts',(-27.5257607197538,9.86353209588784,7.67859857165778));
#27830=CARTESIAN_POINT('Ctrl Pts',(-27.5268652514357,9.87046276675478,7.66968571779361));
#27831=CARTESIAN_POINT('Ctrl Pts',(-27.5279321877019,9.8770136135519,7.66124024409301));
#27832=CARTESIAN_POINT('Ctrl Pts',(-27.5286865720957,9.88164543341441,7.65526881565846));
#27833=CARTESIAN_POINT('Ctrl Pts',(-27.5290901059915,9.88414395336477,7.65204235381507));
#27834=CARTESIAN_POINT('Ctrl Pts',(-27.5298471354527,9.88863381537631,7.6462357579005));
#27835=CARTESIAN_POINT('Ctrl Pts',(-27.5301607832131,9.89049402721282,7.64383000502382));
#27836=CARTESIAN_POINT('Ctrl Pts',(-27.5305351105845,9.89269574853726,7.64098111157456));
#27837=CARTESIAN_POINT('Ctrl Pts',(-27.5310202102533,9.89553012268088,7.63730866150605));
#27838=CARTESIAN_POINT('Ctrl Pts',(-27.5398433802358,9.94708275500642,7.57051279810824));
#27839=CARTESIAN_POINT('Ctrl Pts',(-27.5494881803974,9.99432970581515,7.50790437538638));
#27840=CARTESIAN_POINT('Ctrl Pts',(-27.5599546107381,10.0375302558491,7.44969706517753));
#27841=CARTESIAN_POINT('Ctrl Pts',(-27.5612743460859,10.0429775087394,7.44235757670973));
#27842=CARTESIAN_POINT('Ctrl Pts',(-27.5626071447339,10.0483603838342,7.4350880100706));
#27843=CARTESIAN_POINT('Ctrl Pts',(-27.5639530066821,10.0536793631385,7.42788874870938));
#27844=CARTESIAN_POINT('Ctrl Pts',(-27.5663938375238,10.063325767623,7.41483229875763));
#27845=CARTESIAN_POINT('Ctrl Pts',(-27.568567545298,10.0716796635466,7.40347909748433));
#27846=CARTESIAN_POINT('Ctrl Pts',(-27.5710408659523,10.0807245282707,7.39114287408391));
#27847=CARTESIAN_POINT('Ctrl Pts',(-27.5726273738604,10.0865263434891,7.38322982166737));
#27848=CARTESIAN_POINT('Ctrl Pts',(-27.5743371593522,10.0926117802312,7.37491179089848));
#27849=CARTESIAN_POINT('Ctrl Pts',(-27.5763197999075,10.0994952788321,7.36547317643938));
#27850=CARTESIAN_POINT('Ctrl Pts',(-27.584597958343,10.1282360870729,7.32606394227561));
#27851=CARTESIAN_POINT('Ctrl Pts',(-27.5933465269982,10.1553917388671,7.28835138187274));
#27852=CARTESIAN_POINT('Ctrl Pts',(-27.6028704544253,10.1816400610147,7.25149678810799));
#27853=CARTESIAN_POINT('Ctrl Pts',(-27.6126865511699,10.2086936134022,7.21351159128179));
#27854=CARTESIAN_POINT('Ctrl Pts',(-27.6233263083588,10.2347832137565,7.17643761582166));
#27855=CARTESIAN_POINT('Ctrl Pts',(-27.6351236093967,10.2606068824975,7.13932394578398));
#27856=CARTESIAN_POINT('Ctrl Pts',(-27.6399406587293,10.2711511490102,7.12416976951004));
#27857=CARTESIAN_POINT('Ctrl Pts',(-27.6449506978443,10.2816505856281,7.10900862079852));
#27858=CARTESIAN_POINT('Ctrl Pts',(-27.6501764562545,10.2921506834825,7.09377433447739));
#27859=CARTESIAN_POINT('Ctrl Pts',(-27.6634383936158,10.318797847224,7.05511274029871));
#27860=CARTESIAN_POINT('Ctrl Pts',(-27.6784079583481,10.3457197533343,7.01557869851392));
#27861=CARTESIAN_POINT('Ctrl Pts',(-27.6946104997106,10.3722609327256,6.97611662341272));
#27862=CARTESIAN_POINT('Ctrl Pts',(-27.7110061936436,10.3991185129152,6.93618411586059));
#27863=CARTESIAN_POINT('Ctrl Pts',(-27.7286644363738,10.4255861779289,6.89632538582838));
#27864=CARTESIAN_POINT('Ctrl Pts',(-27.7470933988766,10.4510296958037,6.85754900073121));
#27865=CARTESIAN_POINT('Ctrl Pts',(-27.7522559300769,10.4581572242717,6.84668651740537));
#27866=CARTESIAN_POINT('Ctrl Pts',(-27.7574789424365,10.4652046518517,6.83590914184789));
#27867=CARTESIAN_POINT('Ctrl Pts',(-27.7627516241165,10.4721586455432,6.82523943188631));
#27868=CARTESIAN_POINT('Ctrl Pts',(-27.7939029620164,10.5132432814802,6.76220210847511));
#27869=CARTESIAN_POINT('Ctrl Pts',(-27.8286690447497,10.5537911448996,6.69873608001519));
#27870=CARTESIAN_POINT('Ctrl Pts',(-27.8665602043162,10.593418105067,6.63547231561086));
#27871=CARTESIAN_POINT('Ctrl Pts',(-27.9051373097431,10.6337624343938,6.57106328360848));
#27872=CARTESIAN_POINT('Ctrl Pts',(-27.94695366305,10.6731521330382,6.50686404722303));
#27873=CARTESIAN_POINT('Ctrl Pts',(-27.9914925184439,10.7112289762066,6.44356840727803));
#27874=CARTESIAN_POINT('Ctrl Pts',(-28.0231237052372,10.7382708866487,6.39861628193517));
#27875=CARTESIAN_POINT('Ctrl Pts',(-28.0561280518637,10.7646516481519,6.35412051415379));
#27876=CARTESIAN_POINT('Ctrl Pts',(-28.0903204583934,10.7902569501729,6.31033715020414));
#27877=CARTESIAN_POINT('Ctrl Pts',(-28.1551338489782,10.8387930612383,6.22734362746644));
#27878=CARTESIAN_POINT('Ctrl Pts',(-28.2235523631422,10.8842731098111,6.14738857434825));
#27879=CARTESIAN_POINT('Ctrl Pts',(-28.2960063115382,10.9271272613901,6.07024627287762));
#27880=CARTESIAN_POINT('Ctrl Pts',(-28.3684602599343,10.9699814129692,5.993103971407));
#27881=CARTESIAN_POINT('Ctrl Pts',(-28.4449496425624,11.0102093693281,5.91877394588719));
#27882=CARTESIAN_POINT('Ctrl Pts',(-28.5259047700753,11.0481970286813,5.8469943060891));
#27883=CARTESIAN_POINT('Ctrl Pts',(-28.6326919773777,11.0983062210067,5.75231040513453));
#27884=CARTESIAN_POINT('Ctrl Pts',(-28.7465188395995,11.1437076193583,5.66358519690919));
#27885=CARTESIAN_POINT('Ctrl Pts',(-28.8662849390525,11.1846726988873,5.58149591227711));
#27886=CARTESIAN_POINT('Ctrl Pts',(-28.9799827651499,11.2235621718653,5.50356590327462));
#27887=CARTESIAN_POINT('Ctrl Pts',(-29.0990332207493,11.258454322916,5.43161614291703));
#27888=CARTESIAN_POINT('Ctrl Pts',(-29.2224948231837,11.2895527991727,5.36619023094518));
#27889=CARTESIAN_POINT('Ctrl Pts',(-29.3401771526212,11.3191955468423,5.30382692466527));
#27890=CARTESIAN_POINT('Ctrl Pts',(-29.4618673205163,11.3453920449199,5.24739079413951));
#27891=CARTESIAN_POINT('Ctrl Pts',(-29.5867499650525,11.3682821739022,5.19732242741757));
#27892=CARTESIAN_POINT('Ctrl Pts',(-29.7040975431676,11.3897911770851,5.15027504467817));
#27893=CARTESIAN_POINT('Ctrl Pts',(-29.8242639703085,11.4083810197703,5.10884997192939));
#27894=CARTESIAN_POINT('Ctrl Pts',(-29.9465727484996,11.4241292774221,5.07338843897716));
#27895=CARTESIAN_POINT('Ctrl Pts',(-30.0653024769371,11.4394167030838,5.03896459598184));
#27896=CARTESIAN_POINT('Ctrl Pts',(-30.1860510101812,11.4520267529344,5.01016034153001));
#27897=CARTESIAN_POINT('Ctrl Pts',(-30.3081995172601,11.4619884910358,4.9872657670674));
#27898=CARTESIAN_POINT('Ctrl Pts',(-30.4252659952594,11.4715357677252,4.96532372895557));
#27899=CARTESIAN_POINT('Ctrl Pts',(-30.5436183777033,11.4786506641909,4.9488097989972));
#27900=CARTESIAN_POINT('Ctrl Pts',(-30.6627119045943,11.4833164009267,4.93795954177513));
#27901=CARTESIAN_POINT('Ctrl Pts',(-30.7746849996166,11.4877031799272,4.9277580059347));
#27902=CARTESIAN_POINT('Ctrl Pts',(-30.8873132644994,11.4899248413375,4.92256306618016));
#27903=CARTESIAN_POINT('Ctrl Pts',(-31.0001439249233,11.4899288875684,4.9225536217112));
#27904=CARTESIAN_POINT('Ctrl Pts',(-31.1202005261559,11.4899331929294,4.92254357239623));
#27905=CARTESIAN_POINT('Ctrl Pts',(-31.2399073328591,11.4875055150522,4.92822150864965));
#27906=CARTESIAN_POINT('Ctrl Pts',(-31.3588129466378,11.4826626615451,4.93947954759988));
#27907=CARTESIAN_POINT('Ctrl Pts',(-31.4790662266949,11.4777649195416,4.95086518422166));
#27908=CARTESIAN_POINT('Ctrl Pts',(-31.598500049601,11.4703968194364,4.96795813428723));
#27909=CARTESIAN_POINT('Ctrl Pts',(-31.7166474940121,11.4605262209518,4.99062508498457));
#27910=CARTESIAN_POINT('Ctrl Pts',(-31.8370362660239,11.4504683713172,5.01372204127766));
#27911=CARTESIAN_POINT('Ctrl Pts',(-31.9560893898572,11.4378120739152,5.04260657014114));
#27912=CARTESIAN_POINT('Ctrl Pts',(-32.0733128635378,11.4224738258393,5.07711450511167));
#27913=CARTESIAN_POINT('Ctrl Pts',(-32.163152626949,11.41071863266,5.10356129615291));
#27914=CARTESIAN_POINT('Ctrl Pts',(-32.2519177179933,11.3973871095325,5.13331061927783));
#27915=CARTESIAN_POINT('Ctrl Pts',(-32.3393857592323,11.3824232903062,5.16627912915032));
#27916=CARTESIAN_POINT('Ctrl Pts',(-32.4793850534024,11.3584725524127,5.219047752371));
#27917=CARTESIAN_POINT('Ctrl Pts',(-32.6155704337176,11.3303376850812,5.28007244007344));
#27918=CARTESIAN_POINT('Ctrl Pts',(-32.7467602549158,11.2979857588007,5.3484126424516));
#27919=CARTESIAN_POINT('Ctrl Pts',(-32.8981892942102,11.2606427616746,5.42729598185089));
#27920=CARTESIAN_POINT('Ctrl Pts',(-33.0429625044899,11.2176785361037,5.5159263629673));
#27921=CARTESIAN_POINT('Ctrl Pts',(-33.1792626377584,11.1689943179435,5.61280374908537));
#27922=CARTESIAN_POINT('Ctrl Pts',(-33.282799048435,11.1320127751963,5.68639382265225));
#27923=CARTESIAN_POINT('Ctrl Pts',(-33.3814462928861,11.0917291827592,5.76474127564139));
#27924=CARTESIAN_POINT('Ctrl Pts',(-33.474407836462,11.0481025616628,5.84717280290056));
#27925=CARTESIAN_POINT('Ctrl Pts',(-33.5358302627105,11.0192771698536,5.9016377376346));
#27926=CARTESIAN_POINT('Ctrl Pts',(-33.5945384654344,10.9892895547735,5.95733345481929));
#27927=CARTESIAN_POINT('Ctrl Pts',(-33.6510314177442,10.9577109032453,6.01486257207092));
#27928=CARTESIAN_POINT('Ctrl Pts',(-33.7049759490101,10.9275567780836,6.06979652643865));
#27929=CARTESIAN_POINT('Ctrl Pts',(-33.7569005837092,10.8959519591392,6.12640235390672));
#27930=CARTESIAN_POINT('Ctrl Pts',(-33.807239768638,10.8624837089529,6.18517967990693));
#27931=CARTESIAN_POINT('Ctrl Pts',(-33.8420919974232,10.8393120363447,6.22587403791129));
#27932=CARTESIAN_POINT('Ctrl Pts',(-33.8761842478221,10.8152463489225,6.26760880092171));
#27933=CARTESIAN_POINT('Ctrl Pts',(-33.9096607013978,10.7901374638712,6.3105414593966));
#27934=CARTESIAN_POINT('Ctrl Pts',(-33.9758931100084,10.7404601009238,6.39548275619247));
#27935=CARTESIAN_POINT('Ctrl Pts',(-34.0363090225637,10.6891510387895,6.4809126865769));
#27936=CARTESIAN_POINT('Ctrl Pts',(-34.0909084390637,10.6361483862253,6.56676080774973));
#27937=CARTESIAN_POINT('Ctrl Pts',(-34.115630943938,10.6121488928174,6.60563266261909));
#27938=CARTESIAN_POINT('Ctrl Pts',(-34.1387959172038,10.5882672441134,6.64384519197078));
#27939=CARTESIAN_POINT('Ctrl Pts',(-34.1608991708523,10.5638733668066,6.68240821037408));
#27940=CARTESIAN_POINT('Ctrl Pts',(-34.1825935762304,10.5399307078907,6.72025792097077));
#27941=CARTESIAN_POINT('Ctrl Pts',(-34.2032651764047,10.5154945835208,6.75844537524371));
#27942=CARTESIAN_POINT('Ctrl Pts',(-34.223382775751,10.4899273921746,6.79789844782233));
#27943=CARTESIAN_POINT('Ctrl Pts',(-34.2280352811117,10.4840145845503,6.80702257980792));
#27944=CARTESIAN_POINT('Ctrl Pts',(-34.2326581564576,10.4780411017129,6.81621428094331));
#27945=CARTESIAN_POINT('Ctrl Pts',(-34.2372572003978,10.4719987212801,6.82548480193958));
#27946=CARTESIAN_POINT('Ctrl Pts',(-34.2566870650782,10.4464711038701,6.86465054395384));
#27947=CARTESIAN_POINT('Ctrl Pts',(-34.2750600716674,10.4202268419957,6.9044275590959));
#27948=CARTESIAN_POINT('Ctrl Pts',(-34.2920469852468,10.3938922755973,6.94384643863036));
#27949=CARTESIAN_POINT('Ctrl Pts',(-34.3092271223809,10.3672581575172,6.98371370191544));
#27950=CARTESIAN_POINT('Ctrl Pts',(-34.3249894539689,10.3405317216853,7.02321454878686));
#27951=CARTESIAN_POINT('Ctrl Pts',(-34.3389933818204,10.3144057106446,7.06137627068701));
#27952=CARTESIAN_POINT('Ctrl Pts',(-34.3430311355361,10.3068727956457,7.07237944322795));
#27953=CARTESIAN_POINT('Ctrl Pts',(-34.3469227056967,10.299390071953,7.0832714805828));
#27954=CARTESIAN_POINT('Ctrl Pts',(-34.3506599281287,10.2919747916331,7.09402952407088));
#27955=CARTESIAN_POINT('Ctrl Pts',(-34.3654172613517,10.2626937508031,7.13651027962354));
#27956=CARTESIAN_POINT('Ctrl Pts',(-34.3790083421857,10.2320408948611,7.18041918774137));
#27957=CARTESIAN_POINT('Ctrl Pts',(-34.3914331706306,10.1999569961636,7.22570946526452));
#27958=CARTESIAN_POINT('Ctrl Pts',(-34.3976455848531,10.1839150468149,7.24835460402609));
#27959=CARTESIAN_POINT('Ctrl Pts',(-34.4035664359783,10.1675152840043,7.27134501205274));
#27960=CARTESIAN_POINT('Ctrl Pts',(-34.4091957240062,10.1507499979578,7.29467439156538));
#27961=CARTESIAN_POINT('Ctrl Pts',(-34.4126060387826,10.1405933134089,7.30880771131758));
#27962=CARTESIAN_POINT('Ctrl Pts',(-34.4162059258583,10.1292799124079,7.32448055502478));
#27963=CARTESIAN_POINT('Ctrl Pts',(-34.4194563664031,10.1186636639247,7.3391174984714));
#27964=CARTESIAN_POINT('Ctrl Pts',(-34.4215713150507,10.1117560401538,7.34864124865926));
#27965=CARTESIAN_POINT('Ctrl Pts',(-34.423538320183,10.1051446046541,7.3577271785419));
#27966=CARTESIAN_POINT('Ctrl Pts',(-34.4252088987983,10.0993496647521,7.36567283749913));
#27967=CARTESIAN_POINT('Ctrl Pts',(-34.4336850426113,10.0699474303711,7.40598734134544));
#27968=CARTESIAN_POINT('Ctrl Pts',(-34.4416590954488,10.0383231334541,7.44884386030834));
#27969=CARTESIAN_POINT('Ctrl Pts',(-34.4491310573107,10.004375657046,7.49416224221931));
#27970=CARTESIAN_POINT('Ctrl Pts',(-34.4528670382416,9.98740191884192,7.5168214331748));
#27971=CARTESIAN_POINT('Ctrl Pts',(-34.4564774964286,9.96984721127902,7.54009589904758));
#27972=CARTESIAN_POINT('Ctrl Pts',(-34.4599624318717,9.95169787784942,7.5639744412582));
#27973=CARTESIAN_POINT('Ctrl Pts',(-34.4617048995933,9.94262321113463,7.57591371236351));
#27974=CARTESIAN_POINT('Ctrl Pts',(-34.4634159866289,9.93339987760537,7.58800398998438));
#27975=CARTESIAN_POINT('Ctrl Pts',(-34.4650956929785,9.92402610913804,7.60024379774402));
#27976=CARTESIAN_POINT('Ctrl Pts',(-34.4662208063714,9.91774730186505,7.60844235675998));
#27977=CARTESIAN_POINT('Ctrl Pts',(-34.4676231516465,9.90966212344636,7.61897017985517));
#27978=CARTESIAN_POINT('Ctrl Pts',(-34.4687173436683,9.90326240728531,7.62727957350781));
#27979=CARTESIAN_POINT('Ctrl Pts',(-34.4692566948061,9.90010784746017,7.63137545506384));
#27980=CARTESIAN_POINT('Ctrl Pts',(-34.469721173352,9.89736368664817,7.63493299557365));
#27981=CARTESIAN_POINT('Ctrl Pts',(-34.4700406699694,9.89545169094337,7.63741028308719));
#27982=CARTESIAN_POINT('Ctrl Pts',(-34.4730979206465,9.87715587858438,7.66111535072587));
#27983=CARTESIAN_POINT('Ctrl Pts',(-34.4765052779658,9.85510583171491,7.68951560275804));
#27984=CARTESIAN_POINT('Ctrl Pts',(-34.4802628093407,9.82917908185892,7.72251504218328));
#27985=CARTESIAN_POINT('Ctrl Pts',(-34.4840168568587,9.80327637041435,7.75548388563696));
#27986=CARTESIAN_POINT('Ctrl Pts',(-34.4881204293941,9.77350402572956,7.79304352192599));
#27987=CARTESIAN_POINT('Ctrl Pts',(-34.4925735941727,9.73970141272728,7.83506326655492));
#27988=CARTESIAN_POINT('Ctrl Pts',(-34.4949495421839,9.72166631743482,7.85748254220371));
#27989=CARTESIAN_POINT('Ctrl Pts',(-34.4974250073895,9.70248329584503,7.88117085678994));
#27990=CARTESIAN_POINT('Ctrl Pts',(-34.5,9.68212365416069,7.90610406872703));
#27991=CARTESIAN_POINT('Origin',(-27.5,0.,0.));
#27992=CARTESIAN_POINT('Origin',(-22.75,0.,0.));
#27993=CARTESIAN_POINT('',(-22.75,-3.06161699786838E-15,25.));
#27994=CARTESIAN_POINT('Origin',(-22.75,0.,0.));
#27995=CARTESIAN_POINT('',(-25.,-2.78607146806023E-15,22.75));
#27996=CARTESIAN_POINT('Origin',(-22.75,-2.78607146806023E-15,22.75));
#27997=CARTESIAN_POINT('Origin',(-25.,0.,0.));
#27998=CARTESIAN_POINT('Origin',(0.,0.,0.));
#27999=CARTESIAN_POINT('',(-13.,-3.06161699786838E-15,25.));
#28000=CARTESIAN_POINT('Origin',(-13.,0.,0.));
#28001=CARTESIAN_POINT('',(0.,-3.06161699786838E-15,25.));
#28002=CARTESIAN_POINT('Origin',(0.,0.,0.));
#28003=CARTESIAN_POINT('',(-20.,-2.75545529808154E-15,22.5));
#28004=CARTESIAN_POINT('Origin',(-20.,0.,0.));
#28005=CARTESIAN_POINT('',(-13.,-2.75545529808154E-15,22.5));
#28006=CARTESIAN_POINT('',(0.,-2.75545529808154E-15,22.5));
#28007=CARTESIAN_POINT('Origin',(-13.,0.,0.));
#28008=CARTESIAN_POINT('Origin',(-44.,0.,0.));
#28009=CARTESIAN_POINT('Ctrl Pts',(-36.1184904636295,3.29830760293365E-8,
-4.12499999999999));
#28010=CARTESIAN_POINT('Ctrl Pts',(-36.1188129792782,-0.0284738922563784,
-4.12500000022766));
#28011=CARTESIAN_POINT('Ctrl Pts',(-36.119137418279,-0.0569608644091503,
-4.12470517782373));
#28012=CARTESIAN_POINT('Ctrl Pts',(-36.1254876843367,-0.611496856226084,
-4.11321455467404));
#28013=CARTESIAN_POINT('Ctrl Pts',(-36.1320388503183,-1.13062218918054,
-4.00176801844617));
#28014=CARTESIAN_POINT('Ctrl Pts',(-36.1457516055008,-2.11795055176676,
-3.58174714378506));
#28015=CARTESIAN_POINT('Ctrl Pts',(-36.1527912778546,-2.57357591918388,
-3.26976117732126));
#28016=CARTESIAN_POINT('Ctrl Pts',(-36.165934186153,-3.32415021752054,-2.49909010546225));
#28017=CARTESIAN_POINT('Ctrl Pts',(-36.1715529781619,-3.61689552156258,
-2.05267925260612));
#28018=CARTESIAN_POINT('Ctrl Pts',(-36.1843221264338,-4.0189975245572,-1.07072393112184));
#28019=CARTESIAN_POINT('Ctrl Pts',(-36.1911232640831,-4.12346679901638,
-0.543881494992523));
#28020=CARTESIAN_POINT('Ctrl Pts',(-36.2049491490745,-4.12653977793352,
0.534433978155843));
#28021=CARTESIAN_POINT('Ctrl Pts',(-36.2118384570041,-4.01959947188852,
1.07553630532412));
#28022=CARTESIAN_POINT('Ctrl Pts',(-36.2243033575539,-3.61049936724165,
2.0620880236769));
#28023=CARTESIAN_POINT('Ctrl Pts',(-36.2300451849934,-3.3209633622173,2.50182336289408));
#28024=CARTESIAN_POINT('Ctrl Pts',(-36.2432508971558,-2.58193474564445,
3.26173128216171));
#28025=CARTESIAN_POINT('Ctrl Pts',(-36.2502136603053,-2.13480494949125,
3.57041793481763));
#28026=CARTESIAN_POINT('Ctrl Pts',(-36.2639684640228,-1.14000541154513,
4.00177987603652));
#28027=CARTESIAN_POINT('Ctrl Pts',(-36.2704812921315,-0.60079422594595,
4.11738773792091));
#28028=CARTESIAN_POINT('Ctrl Pts',(-36.2825196776631,0.469593642929444,
4.13159746634345));
#28029=CARTESIAN_POINT('Ctrl Pts',(-36.2889803312695,0.990488073958131,
4.03850712175553));
#28030=CARTESIAN_POINT('Ctrl Pts',(-36.3025946858657,1.9884930745957,3.65490487200752));
#28031=CARTESIAN_POINT('Ctrl Pts',(-36.3096317543173,2.45329967538008,3.36061865545876));
#28032=CARTESIAN_POINT('Ctrl Pts',(-36.3229459347788,3.23315456097611,2.61657770970833));
#28033=CARTESIAN_POINT('Ctrl Pts',(-36.3286722456059,3.5438698456838,2.17732672202478));
#28034=CARTESIAN_POINT('Ctrl Pts',(-36.3413023232013,3.97983419336367,1.20740145021164));
#28035=CARTESIAN_POINT('Ctrl Pts',(-36.3480384347988,4.10194551352598,0.686247137589298));
#28036=CARTESIAN_POINT('Ctrl Pts',(-36.3619189074336,4.14293964986017,-0.395001950570159));
#28037=CARTESIAN_POINT('Ctrl Pts',(-36.368928880632,4.05303669850736,-0.944921243939712));
#28038=CARTESIAN_POINT('Ctrl Pts',(-36.3816408239285,3.67252141824346,-1.94974415955186));
#28039=CARTESIAN_POINT('Ctrl Pts',(-36.3872785848625,3.39612511880639,-2.39901076688027));
#28040=CARTESIAN_POINT('Ctrl Pts',(-36.4003710697463,2.68100395729819,-3.180522530576));
#28041=CARTESIAN_POINT('Ctrl Pts',(-36.4072989140441,2.24502112269832,-3.50191138006792));
#28042=CARTESIAN_POINT('Ctrl Pts',(-36.4210898632463,1.26593074560354,-3.96373034594873));
#28043=CARTESIAN_POINT('Ctrl Pts',(-36.4278135140083,0.730737603887081,
-4.09631201729583));
#28044=CARTESIAN_POINT('Ctrl Pts',(-36.4346052355924,0.123501653108671,
-4.12361452133081));
#28045=CARTESIAN_POINT('Ctrl Pts',(-36.4352913126543,0.0617259448598127,
-4.12499999999999));
#28046=CARTESIAN_POINT('Ctrl Pts',(-36.4359904640031,3.27860210979314E-14,
-4.12499999999999));
#28047=CARTESIAN_POINT('Ctrl Pts',(-36.3566154631359,-4.99089713584757E-13,
-4.12499999999999));
#28048=CARTESIAN_POINT('Ctrl Pts',(-36.356350447845,0.0233973935143799,
-4.12499999999999));
#28049=CARTESIAN_POINT('Ctrl Pts',(-36.3560865337059,0.0468034160332337,
-4.12480093196674));
#28050=CARTESIAN_POINT('Ctrl Pts',(-36.3496955247249,0.616200357154302,
-4.11510727677789));
#28051=CARTESIAN_POINT('Ctrl Pts',(-36.343151671704,1.15495332093977,-3.9974884183394));
#28052=CARTESIAN_POINT('Ctrl Pts',(-36.3293919969298,2.14793688048322,-3.562503756747));
#28053=CARTESIAN_POINT('Ctrl Pts',(-36.3224330248351,2.59376818274409,-3.25229675530295));
#28054=CARTESIAN_POINT('Ctrl Pts',(-36.3092405211388,3.329980523612,-2.48982485883441));
#28055=CARTESIAN_POINT('Ctrl Pts',(-36.3035136276204,3.61796642737089,-2.0489783562903));
#28056=CARTESIAN_POINT('Ctrl Pts',(-36.2910270965324,4.0234975201098,-1.06086408272591));
#28057=CARTESIAN_POINT('Ctrl Pts',(-36.2841318684387,4.1284637457095,-0.519368917559876));
#28058=CARTESIAN_POINT('Ctrl Pts',(-36.2703067656381,4.12145458755141,0.558748090084849));
#28059=CARTESIAN_POINT('Ctrl Pts',(-36.2635120490944,4.01513553202157,1.08502508246555));
#28060=CARTESIAN_POINT('Ctrl Pts',(-36.2507572006762,3.60950704474773,2.06574186393406));
#28061=CARTESIAN_POINT('Ctrl Pts',(-36.2451303961666,3.31491499256384,2.5114079653395));
#28062=CARTESIAN_POINT('Ctrl Pts',(-36.2319694875181,2.5613008089251,3.2793506876566));
#28063=CARTESIAN_POINT('Ctrl Pts',(-36.2249296693748,2.10469647472789,3.5895196928067));
#28064=CARTESIAN_POINT('Ctrl Pts',(-36.2112263289609,1.11620480638802,4.00578944532168));
#28065=CARTESIAN_POINT('Ctrl Pts',(-36.2046841781791,0.596867108969412,
4.11533966572925));
#28066=CARTESIAN_POINT('Ctrl Pts',(-36.1924184950835,-0.476214249019286,
4.13380553048062));
#28067=CARTESIAN_POINT('Ctrl Pts',(-36.1861212783578,-1.01984834863037,
4.03423470121718));
#28068=CARTESIAN_POINT('Ctrl Pts',(-36.1723992977249,-2.02953298946384,
3.63152228096813));
#28069=CARTESIAN_POINT('Ctrl Pts',(-36.1654096344374,-2.48679250804523,
3.33508947972833));
#28070=CARTESIAN_POINT('Ctrl Pts',(-36.1521006902102,-3.24810574947604,
2.59565866040361));
#28071=CARTESIAN_POINT('Ctrl Pts',(-36.1462156604452,-3.54994049759374,
2.16461282875544));
#28072=CARTESIAN_POINT('Ctrl Pts',(-36.1339228823,-3.98705269692777,1.1905085008082));
#28073=CARTESIAN_POINT('Ctrl Pts',(-36.1270834397453,-4.10947705763902,
0.652754971315038));
#28074=CARTESIAN_POINT('Ctrl Pts',(-36.1132578692447,-4.13743266360497,
-0.426619513520434));
#28075=CARTESIAN_POINT('Ctrl Pts',(-36.1064090845789,-4.04761502808193,
-0.957690076385819));
#28076=CARTESIAN_POINT('Ctrl Pts',(-36.0935288802234,-3.67327189816729,
-1.9492771637618));
#28077=CARTESIAN_POINT('Ctrl Pts',(-36.0879476338471,-3.39487095018637,
-2.40155343925716));
#28078=CARTESIAN_POINT('Ctrl Pts',(-36.0749475495251,-2.6681375583289,-3.19334772538381));
#28079=CARTESIAN_POINT('Ctrl Pts',(-36.067912310006,-2.22039104239074,-3.51941561244037));
#28080=CARTESIAN_POINT('Ctrl Pts',(-36.0541320734522,-1.24261636540952,
-3.96860920734908));
#28081=CARTESIAN_POINT('Ctrl Pts',(-36.0475132450743,-0.725382649545967,
-4.09484826686876));
#28082=CARTESIAN_POINT('Ctrl Pts',(-36.0406230669347,-0.132256996684131,
-4.12341124761089));
#28083=CARTESIAN_POINT('Ctrl Pts',(-36.0398641502892,-0.0660993102846563,
-4.12499999999999));
#28084=CARTESIAN_POINT('Ctrl Pts',(-36.0391154631359,3.30485893395058E-14,
-4.12499999999999));
#28085=CARTESIAN_POINT('Origin',(-36.,-4.40872847693047E-15,0.));
#28086=CARTESIAN_POINT('Ctrl Pts',(-36.,2.8677394674816,-2.96507931540595));
#28087=CARTESIAN_POINT('Ctrl Pts',(-36.,2.58211488762459,-3.25359758419502));
#28088=CARTESIAN_POINT('Ctrl Pts',(-36.,2.2556303657079,-3.49857150536326));
#28089=CARTESIAN_POINT('Ctrl Pts',(-36.,1.53011798561339,-3.89209437568881));
#28090=CARTESIAN_POINT('Ctrl Pts',(-36.0000000000009,1.13324515947091,-4.03492093053112));
#28091=CARTESIAN_POINT('Ctrl Pts',(-36.0000000000009,0.144604455351344,
-4.22907725009426));
#28092=CARTESIAN_POINT('Ctrl Pts',(-36.,-0.418973144257557,-4.2124931411291));
#28093=CARTESIAN_POINT('Ctrl Pts',(-36.,-1.46036865006272,-3.99898257282591));
#28094=CARTESIAN_POINT('Ctrl Pts',(-36.,-1.96289610596394,-3.79090818666882));
#28095=CARTESIAN_POINT('Ctrl Pts',(-36.,-2.75244104700568,-3.27033011728567));
#28096=CARTESIAN_POINT('Ctrl Pts',(-36.,-3.05797105898633,-2.99870283738677));
#28097=CARTESIAN_POINT('Ctrl Pts',(-36.,-3.60220512633872,-2.35292484380394));
#28098=CARTESIAN_POINT('Ctrl Pts',(-36.,-3.83066360686449,-1.97559567188751));
#28099=CARTESIAN_POINT('Ctrl Pts',(-36.,-3.99810942017504,-1.57418469260505));
#28100=CARTESIAN_POINT('Ctrl Pts',(-36.,-3.96679264203453,1.65151219106172));
#28101=CARTESIAN_POINT('Ctrl Pts',(-36.,-3.78888208787887,2.05652148838597));
#28102=CARTESIAN_POINT('Ctrl Pts',(-36.,-3.54982596258504,2.4323494533105));
#28103=CARTESIAN_POINT('Ctrl Pts',(-36.,-2.98666653493592,3.06859799774672));
#28104=CARTESIAN_POINT('Ctrl Pts',(-36.,-2.67569031699454,3.332187707082));
#28105=CARTESIAN_POINT('Ctrl Pts',(-36.,-1.88238697005194,3.82949480800279));
#28106=CARTESIAN_POINT('Ctrl Pts',(-36.,-1.38380077745684,4.02451205440474));
#28107=CARTESIAN_POINT('Ctrl Pts',(-36.,-0.364900368386679,4.21598353592192));
#28108=CARTESIAN_POINT('Ctrl Pts',(-35.9999999999974,0.197924631338814,
4.22987474907417));
#28109=CARTESIAN_POINT('Ctrl Pts',(-35.9999999999974,1.19242231635065,4.01726970897806));
#28110=CARTESIAN_POINT('Ctrl Pts',(-36.,1.58187588327058,3.87073756876392));
#28111=CARTESIAN_POINT('Ctrl Pts',(-36.,2.30197555597678,3.46876308718649));
#28112=CARTESIAN_POINT('Ctrl Pts',(-36.,2.62903433812351,3.21631429554064));
#28113=CARTESIAN_POINT('Ctrl Pts',(-36.,2.91366312592486,2.91996441564374));
#28114=CARTESIAN_POINT('Origin',(-20.,8.,0.));
#28115=CARTESIAN_POINT('Origin',(-13.,22.5,0.));
#28116=CARTESIAN_POINT('Origin',(-25.,22.75,0.));
#28117=CARTESIAN_POINT('Origin',(-44.,11.5,0.));
#28118=CARTESIAN_POINT('Ctrl Pts',(-27.4978820065166,9.67657286048411,7.93453028901309));
#28119=CARTESIAN_POINT('Ctrl Pts',(-27.5051002838282,9.73192148554358,7.86702396692179));
#28120=CARTESIAN_POINT('Ctrl Pts',(-27.5115777941627,9.77905015687421,7.80813914050018));
#28121=CARTESIAN_POINT('Ctrl Pts',(-27.5198997026027,9.8361990199015,7.73581472965319));
#28122=CARTESIAN_POINT('Ctrl Pts',(-27.5223343384609,9.85237966752398,7.71518001660921));
#28123=CARTESIAN_POINT('Ctrl Pts',(-27.5257607197538,9.8743467249716,7.68701758369407));
#28124=CARTESIAN_POINT('Ctrl Pts',(-27.5268652514357,9.8812849948035,7.67809495754876));
#28125=CARTESIAN_POINT('Ctrl Pts',(-27.5289991239681,9.89440105342999,7.66118549048045));
#28126=CARTESIAN_POINT('Ctrl Pts',(-27.5293642597536,9.89669372379413,7.65823253102818));
#28127=CARTESIAN_POINT('Ctrl Pts',(-27.5376440122518,9.9451242809251,7.59548188702668));
#28128=CARTESIAN_POINT('Ctrl Pts',(-27.5447308790556,9.98143874139635,7.54764313910302));
#28129=CARTESIAN_POINT('Ctrl Pts',(-27.5560557764691,10.0324327883853,7.4795666351035));
#28130=CARTESIAN_POINT('Ctrl Pts',(-27.5599465084749,10.0488510371663,7.45748786474674));
#28131=CARTESIAN_POINT('Ctrl Pts',(-27.5679595048892,10.0805539119409,7.41457788740912));
#28132=CARTESIAN_POINT('Ctrl Pts',(-27.5712462791805,10.0929346338891,7.39772849754879));
#28133=CARTESIAN_POINT('Ctrl Pts',(-27.5966138828154,10.1811045843937,7.27683035868852));
#28134=CARTESIAN_POINT('Ctrl Pts',(-27.6197351110962,10.2422025103862,7.19039294558005));
#28135=CARTESIAN_POINT('Ctrl Pts',(-27.6806178014129,10.3646680115295,7.0127113149185));
#28136=CARTESIAN_POINT('Ctrl Pts',(-27.7200563355264,10.4272692165682,6.91921499537165));
#28137=CARTESIAN_POINT('Ctrl Pts',(-27.8481422012966,10.5963833319316,6.65973840660726));
#28138=CARTESIAN_POINT('Ctrl Pts',(-27.9606936772239,10.7049090095097,6.48342500331331));
#28139=CARTESIAN_POINT('Ctrl Pts',(-28.2199472395629,10.8992663187099,6.15108692747109));
#28140=CARTESIAN_POINT('Ctrl Pts',(-28.3639945150494,10.9842519347326,5.99712178198714));
#28141=CARTESIAN_POINT('Ctrl Pts',(-29.1735457901792,11.364545034686,5.27853837366088));
#28142=CARTESIAN_POINT('Ctrl Pts',(-30.0801163558429,11.5024937103589,4.92802793068232));
#28143=CARTESIAN_POINT('Ctrl Pts',(-31.4601577094634,11.5025432544128,4.92791228792853));
#28144=CARTESIAN_POINT('Ctrl Pts',(-31.9150359953972,11.4675795904092,5.01182201720196));
#28145=CARTESIAN_POINT('Ctrl Pts',(-32.7637355230674,11.3222269507453,5.33206512247338));
#28146=CARTESIAN_POINT('Ctrl Pts',(-33.1530450432979,11.2111961005192,5.56831023126238));
#28147=CARTESIAN_POINT('Ctrl Pts',(-33.635089233044,10.9847259259335,5.99622057363153));
#28148=CARTESIAN_POINT('Ctrl Pts',(-33.7771958841765,10.90143170776,6.14739164137836));
#28149=CARTESIAN_POINT('Ctrl Pts',(-33.9758931100084,10.7522362163205,6.40249492720256));
#28150=CARTESIAN_POINT('Ctrl Pts',(-34.0363090225637,10.700870897617,6.48801852514955));
#28151=CARTESIAN_POINT('Ctrl Pts',(-34.1455078555637,10.5947493655584,6.65990301965054));
#28152=CARTESIAN_POINT('Ctrl Pts',(-34.1925105204025,10.5423346581866,6.74267144025955));
#28153=CARTESIAN_POINT('Ctrl Pts',(-34.282003880393,10.4246263193092,6.92326543614069));
#28154=CARTESIAN_POINT('Ctrl Pts',(-34.3211452616827,10.3618854668815,7.01675293455816));
#28155=CARTESIAN_POINT('Ctrl Pts',(-34.3654172613517,10.2739460309433,7.14433493217967));
#28156=CARTESIAN_POINT('Ctrl Pts',(-34.3790083421857,10.2432595664254,7.18829198314837));
#28157=CARTESIAN_POINT('Ctrl Pts',(-34.3976455848531,10.1950809519674,7.25630188556257));
#28158=CARTESIAN_POINT('Ctrl Pts',(-34.4035664359783,10.1786632080371,7.27931750086111));
#28159=CARTESIAN_POINT('Ctrl Pts',(-34.4148250120342,10.1450958721665,7.32602741774418));
#28160=CARTESIAN_POINT('Ctrl Pts',(-34.4209708268918,10.1251400861266,7.35356939689983));
#28161=CARTESIAN_POINT('Ctrl Pts',(-34.4336850426113,10.0809883785116,7.41410745545032));
#28162=CARTESIAN_POINT('Ctrl Pts',(-34.4416590954488,10.0493294079059,7.45701096339767));
#28163=CARTESIAN_POINT('Ctrl Pts',(-34.4528670382416,9.99835236197048,7.52506306861516));
#28164=CARTESIAN_POINT('Ctrl Pts',(-34.4564774964286,9.98077840697682,7.54836305320812));
#28165=CARTESIAN_POINT('Ctrl Pts',(-34.4617048995933,9.95352455774178,7.58422013809147));
#28166=CARTESIAN_POINT('Ctrl Pts',(-34.4634159866289,9.94429111151353,7.59632367180222));
#28167=CARTESIAN_POINT('Ctrl Pts',(-34.4667753993281,9.92552301929947,7.6208301273986));
#28168=CARTESIAN_POINT('Ctrl Pts',(-34.469073004422,9.91209856492485,7.6382729004231));
#28169=CARTESIAN_POINT('Ctrl Pts',(-34.47820638366,9.85738083779885,7.70916821772884));
#28170=CARTESIAN_POINT('Ctrl Pts',(-34.4888697183811,9.7817723769294,7.80619779242128));
#28171=CARTESIAN_POINT('Ctrl Pts',(-34.5020319587248,9.67657706129138,7.93452721162802));
#28172=CARTESIAN_POINT('Ctrl Pts',(-27.4978820071632,3.47975094352918,2.85330246801448));
#28173=CARTESIAN_POINT('Ctrl Pts',(-27.5051002818624,3.49965461851457,2.82902681724709));
#28174=CARTESIAN_POINT('Ctrl Pts',(-27.5115777941627,3.51660236362271,2.80785149032865));
#28175=CARTESIAN_POINT('Ctrl Pts',(-27.5198997026027,3.53715342160648,2.78184321855869));
#28176=CARTESIAN_POINT('Ctrl Pts',(-27.5223343384609,3.54297207503001,2.77442285773641));
#28177=CARTESIAN_POINT('Ctrl Pts',(-27.5257607197538,3.55087155451962,2.7642954857968));
#28178=CARTESIAN_POINT('Ctrl Pts',(-27.5268652514357,3.55336659603172,2.7610868584057));
#28179=CARTESIAN_POINT('Ctrl Pts',(-27.5289991239681,3.55808320572565,2.75500611734127));
#28180=CARTESIAN_POINT('Ctrl Pts',(-27.5293642597536,3.55890766310057,2.75394421623401));
#28181=CARTESIAN_POINT('Ctrl Pts',(-27.5376440122518,3.5763235684233,2.73137872577486));
#28182=CARTESIAN_POINT('Ctrl Pts',(-27.5447308790556,3.58938245609422,2.71417563842768));
#28183=CARTESIAN_POINT('Ctrl Pts',(-27.5560557764691,3.60772020703069,2.6896949382542));
#28184=CARTESIAN_POINT('Ctrl Pts',(-27.5599465084749,3.61362430318968,2.68175528616356));
#28185=CARTESIAN_POINT('Ctrl Pts',(-27.5679595048892,3.62502483827003,2.66632461290719));
#28186=CARTESIAN_POINT('Ctrl Pts',(-27.5712462791805,3.62947701668899,2.66026547595033));
#28187=CARTESIAN_POINT('Ctrl Pts',(-27.5966138828154,3.66118343514184,2.61678981378955));
#28188=CARTESIAN_POINT('Ctrl Pts',(-27.6197351110962,3.68315459875289,2.5857064256929));
#28189=CARTESIAN_POINT('Ctrl Pts',(-27.6806178014129,3.72719389335453,2.52181109513081));
#28190=CARTESIAN_POINT('Ctrl Pts',(-27.7200563355264,3.74970564470802,2.48818928390845));
#28191=CARTESIAN_POINT('Ctrl Pts',(-27.8481422012966,3.81052004777055,2.39488001862033));
#28192=CARTESIAN_POINT('Ctrl Pts',(-27.9606936772239,3.84954650209512,2.33147671044463));
#28193=CARTESIAN_POINT('Ctrl Pts',(-28.2199472395629,3.91943850202933,2.21196603770235));
#28194=CARTESIAN_POINT('Ctrl Pts',(-28.3639945150494,3.94999981559095,2.1565992908467));
#28195=CARTESIAN_POINT('Ctrl Pts',(-29.1735457901792,4.08675538926246,1.89819258757359));
#28196=CARTESIAN_POINT('Ctrl Pts',(-30.0801163558429,4.13636252197452,1.77214702767979));
#28197=CARTESIAN_POINT('Ctrl Pts',(-31.4601577094634,4.13638033829966,1.77210544188415));
#28198=CARTESIAN_POINT('Ctrl Pts',(-31.9150359953972,4.1238072047638,1.80227986041768));
#28199=CARTESIAN_POINT('Ctrl Pts',(-32.7637355230674,4.07153756425668,1.91744111257055));
#28200=CARTESIAN_POINT('Ctrl Pts',(-33.1530450432979,4.03161023552061,2.00239620479673));
#28201=CARTESIAN_POINT('Ctrl Pts',(-33.635089233044,3.9501702655376,2.15627521116793));
#28202=CARTESIAN_POINT('Ctrl Pts',(-33.7771958841765,3.92021718831577,2.21063719168975));
#28203=CARTESIAN_POINT('Ctrl Pts',(-33.9758931100084,3.86656563633256,2.30237379222929));
#28204=CARTESIAN_POINT('Ctrl Pts',(-34.0363090225637,3.84809437396421,2.33312856716768));
#28205=CARTESIAN_POINT('Ctrl Pts',(-34.1455078555637,3.80993246411797,2.39493921441212));
#28206=CARTESIAN_POINT('Ctrl Pts',(-34.1925105204025,3.79108383558294,2.42470321182269));
#28207=CARTESIAN_POINT('Ctrl Pts',(-34.282003880393,3.74875524373872,2.48964584557381));
#28208=CARTESIAN_POINT('Ctrl Pts',(-34.3211452616827,3.72619327438553,2.5232644846676));
#28209=CARTESIAN_POINT('Ctrl Pts',(-34.3654172613517,3.6945697502891,2.56914370066447));
#28210=CARTESIAN_POINT('Ctrl Pts',(-34.3790083421857,3.68353472214999,2.58495090758689));
#28211=CARTESIAN_POINT('Ctrl Pts',(-34.3976455848531,3.66620941685335,2.60940765744939));
#28212=CARTESIAN_POINT('Ctrl Pts',(-34.4035664359783,3.66030550224154,2.61768420433899));
#28213=CARTESIAN_POINT('Ctrl Pts',(-34.4148250120342,3.64823449628808,2.63448135758808));
#28214=CARTESIAN_POINT('Ctrl Pts',(-34.4209708268918,3.64105828149931,2.64438561080735));
#28215=CARTESIAN_POINT('Ctrl Pts',(-34.4336850426113,3.6251810749336,2.66615544288436));
#28216=CARTESIAN_POINT('Ctrl Pts',(-34.4416590954488,3.61379632804348,2.681583789711));
#28217=CARTESIAN_POINT('Ctrl Pts',(-34.4528670382416,3.59546469078309,2.70605571594293));
#28218=CARTESIAN_POINT('Ctrl Pts',(-34.4564774964286,3.58914499606044,2.71443452365713));
#28219=CARTESIAN_POINT('Ctrl Pts',(-34.4617048995933,3.57934435600846,2.72732893645086));
#28220=CARTESIAN_POINT('Ctrl Pts',(-34.4634159866289,3.57602395593793,2.73168143639438));
#28221=CARTESIAN_POINT('Ctrl Pts',(-34.4667753993281,3.56927484264146,2.74049409798132));
#28222=CARTESIAN_POINT('Ctrl Pts',(-34.469073004422,3.56444733207276,2.74676661891762));
#28223=CARTESIAN_POINT('Ctrl Pts',(-34.47820638366,3.54477052446296,2.77226098047704));
#28224=CARTESIAN_POINT('Ctrl Pts',(-34.4888697350336,3.51758124217551,2.80715342844052));
#28225=CARTESIAN_POINT('Ctrl Pts',(-34.5020319559861,3.47975246018584,2.85330135399401));
#28226=CARTESIAN_POINT('',(-27.5,6.19655913866284,5.0599066039853));
#28227=CARTESIAN_POINT('',(-34.5,6.19655913866284,5.0599066039853));
#28228=CARTESIAN_POINT('Origin',(-34.5,0.,0.));
#28229=CARTESIAN_POINT('',(-34.5,-2.47065947129021,7.60893171062298));
#28230=CARTESIAN_POINT('Ctrl Pts',(-34.5021179935156,-3.84034921836418,
11.9098510115161));
#28231=CARTESIAN_POINT('Ctrl Pts',(-34.494899716168,-3.92343148484306,11.8830571522946));
#28232=CARTESIAN_POINT('Ctrl Pts',(-34.4884222058122,-3.99493511172526,
11.8590620314241));
#28233=CARTESIAN_POINT('Ctrl Pts',(-34.4801002973656,-4.08213937064346,
11.8291918089636));
#28234=CARTESIAN_POINT('Ctrl Pts',(-34.4776656615101,-4.10691485581785,
11.8206022762278));
#28235=CARTESIAN_POINT('Ctrl Pts',(-34.4742392802251,-4.1406307585753,11.8088161769966));
#28236=CARTESIAN_POINT('Ctrl Pts',(-34.4731347485465,-4.15129480472915,
11.8050703841133));
#28237=CARTESIAN_POINT('Ctrl Pts',(-34.471000876022,-4.17147688887322,11.7979538859599));
#28238=CARTESIAN_POINT('Ctrl Pts',(-34.4706357402539,-4.17500317883281,
11.796712280233));
#28239=CARTESIAN_POINT('Ctrl Pts',(-34.4623559877182,-4.2496942586282,11.770171654287));
#28240=CARTESIAN_POINT('Ctrl Pts',(-34.4552691208995,-4.3061254359688,11.7496093567904));
#28241=CARTESIAN_POINT('Ctrl Pts',(-34.4439442234859,-4.38585513082339,
11.7199786466456));
#28242=CARTESIAN_POINT('Ctrl Pts',(-34.4400534914838,-4.41161216089477,
11.710303606902));
#28243=CARTESIAN_POINT('Ctrl Pts',(-34.4320404950846,-4.46149769348112,
11.6913887436455));
#28244=CARTESIAN_POINT('Ctrl Pts',(-34.4287537208257,-4.48102899522492,
11.6839246657677));
#28245=CARTESIAN_POINT('Ctrl Pts',(-34.4033861171601,-4.62061175533369,
11.6300084968999));
#28246=CARTESIAN_POINT('Ctrl Pts',(-34.3802648888803,-4.71877671883352,
11.5904102281741));
#28247=CARTESIAN_POINT('Ctrl Pts',(-34.3193821986106,-4.91793563737523,
11.507318195227));
#28248=CARTESIAN_POINT('Ctrl Pts',(-34.2799436644392,-5.02118603476733,
11.4625987574891));
#28249=CARTESIAN_POINT('Ctrl Pts',(-34.1518577987722,-5.30384788925113,
11.3359892789864));
#28250=CARTESIAN_POINT('Ctrl Pts',(-34.0393063228094,-5.49054572845524,
11.2465009795587));
#28251=CARTESIAN_POINT('Ctrl Pts',(-33.7800527604038,-5.83387687678551,
11.0722968378733));
#28252=CARTESIAN_POINT('Ctrl Pts',(-33.6360054850864,-5.98868389780719,
10.9888545995394));
#28253=CARTESIAN_POINT('Ctrl Pts',(-32.8264542092776,-6.69744947821504,
10.590562860345));
#28254=CARTESIAN_POINT('Ctrl Pts',(-31.9198836441155,-7.00319127556429,
10.3705415868347));
#28255=CARTESIAN_POINT('Ctrl Pts',(-30.5398422905574,-7.00329553722076,
10.3704711782771));
#28256=CARTESIAN_POINT('Ctrl Pts',(-30.08496400456,-6.92847222075559,10.4220926058383));
#28257=CARTESIAN_POINT('Ctrl Pts',(-29.2362644769754,-6.63289122824282,
10.6126573275853));
#28258=CARTESIAN_POINT('Ctrl Pts',(-28.8469549569745,-6.41164166105415,
10.7511789144381));
#28259=CARTESIAN_POINT('Ctrl Pts',(-28.3649107668198,-5.98957031134368,
10.9883534856232));
#28260=CARTESIAN_POINT('Ctrl Pts',(-28.2228041159262,-5.83769802696752,
11.0703621901657));
#28261=CARTESIAN_POINT('Ctrl Pts',(-28.0241068899402,-5.57415098904807,
11.2040780834347));
#28262=CARTESIAN_POINT('Ctrl Pts',(-27.9636909773592,-5.48466374516304,
11.2481770059251));
#28263=CARTESIAN_POINT('Ctrl Pts',(-27.8544921443592,-5.30238496198931,
11.3352430970402));
#28264=CARTESIAN_POINT('Ctrl Pts',(-27.8074894795624,-5.21350699011682,
11.3764574039751));
#28265=CARTESIAN_POINT('Ctrl Pts',(-27.717996119642,-5.01677113301965,11.4645735027238));
#28266=CARTESIAN_POINT('Ctrl Pts',(-27.678854738298,-4.91340809804618,11.5092099224669));
#28267=CARTESIAN_POINT('Ctrl Pts',(-27.6345827386579,-4.77040068831785,
11.5688705562283));
#28268=CARTESIAN_POINT('Ctrl Pts',(-27.6209916578288,-4.72080287780926,
11.5892160378951));
#28269=CARTESIAN_POINT('Ctrl Pts',(-27.6023544151614,-4.64347640529298,
11.6203149505103));
#28270=CARTESIAN_POINT('Ctrl Pts',(-27.596433564035,-4.61721261685308,11.6307779462829));
#28271=CARTESIAN_POINT('Ctrl Pts',(-27.5851749879742,-4.56370229244711,
11.6518783623449));
#28272=CARTESIAN_POINT('Ctrl Pts',(-27.579029173103,-4.53201332813435,11.6642316436317));
#28273=CARTESIAN_POINT('Ctrl Pts',(-27.566314957399,-4.46211766449134,11.6912284213788));
#28274=CARTESIAN_POINT('Ctrl Pts',(-27.5583409045667,-4.4122725480453,11.710161613854));
#28275=CARTESIAN_POINT('Ctrl Pts',(-27.5471329617739,-4.33257035622456,
11.7397810138477));
#28276=CARTESIAN_POINT('Ctrl Pts',(-27.5435225035856,-4.305180495978,11.7498571605463));
#28277=CARTESIAN_POINT('Ctrl Pts',(-27.538295100417,-4.26285387292635,11.7652506597461));
#28278=CARTESIAN_POINT('Ctrl Pts',(-27.5365840133798,-4.24853802456432,
11.7704283564838));
#28279=CARTESIAN_POINT('Ctrl Pts',(-27.5332246006767,-4.21949100363759,
11.7808724087611));
#28280=CARTESIAN_POINT('Ctrl Pts',(-27.5309269955758,-4.19876090805562,
11.7882703439938));
#28281=CARTESIAN_POINT('Ctrl Pts',(-27.521793616354,-4.11437437864175,11.8182551616966));
#28282=CARTESIAN_POINT('Ctrl Pts',(-27.5111302816239,-3.99827490007513,
11.8589035174418));
#28283=CARTESIAN_POINT('Ctrl Pts',(-27.4979680412483,-3.84035441638973,
11.9098506982947));
#28284=CARTESIAN_POINT('Ctrl Pts',(-34.502117992869,-1.38101154484016,4.2828505362653));
#28285=CARTESIAN_POINT('Ctrl Pts',(-34.4948997181338,-1.41088839229903,
4.2732153147342));
#28286=CARTESIAN_POINT('Ctrl Pts',(-34.4884222058122,-1.43660151352823,
4.26458652941962));
#28287=CARTESIAN_POINT('Ctrl Pts',(-34.4801002973656,-1.46796066376331,
4.25384502659264));
#28288=CARTESIAN_POINT('Ctrl Pts',(-34.4776656615101,-1.47687006992499,
4.25075618149666));
#28289=CARTESIAN_POINT('Ctrl Pts',(-34.4742392802251,-1.4889945013805,4.24651783280745));
#28290=CARTESIAN_POINT('Ctrl Pts',(-34.4731347485465,-1.49282935336596,
4.24517082426415));
#28291=CARTESIAN_POINT('Ctrl Pts',(-34.471000876022,-1.50008694624711,4.24261169082837));
#28292=CARTESIAN_POINT('Ctrl Pts',(-34.4706357402539,-1.50135502028371,
4.24216520230811));
#28293=CARTESIAN_POINT('Ctrl Pts',(-34.4623559877182,-1.52821435974236,
4.23262104143));
#28294=CARTESIAN_POINT('Ctrl Pts',(-34.4552691208995,-1.54850733384844,
4.2252267216528));
#28295=CARTESIAN_POINT('Ctrl Pts',(-34.4439442234859,-1.57717858809862,
4.21457134882434));
#28296=CARTESIAN_POINT('Ctrl Pts',(-34.4400534914838,-1.58644096341879,
4.21109214920023));
#28297=CARTESIAN_POINT('Ctrl Pts',(-34.4320404950845,-1.60438008623618,
4.20429025619756));
#28298=CARTESIAN_POINT('Ctrl Pts',(-34.4287537208257,-1.61140365404432,
4.20160613110506));
#28299=CARTESIAN_POINT('Ctrl Pts',(-34.4033861171601,-1.66159841286434,
4.18221756842935));
#28300=CARTESIAN_POINT('Ctrl Pts',(-34.3802648888803,-1.69689909515212,
4.16797780452988));
#28301=CARTESIAN_POINT('Ctrl Pts',(-34.3193821986106,-1.76851778126542,
4.13809743427216));
#28302=CARTESIAN_POINT('Ctrl Pts',(-34.2799436644392,-1.80564721466486,
4.12201606870759));
#28303=CARTESIAN_POINT('Ctrl Pts',(-34.1518577987722,-1.90729403410288,
4.07648657614834));
#28304=CARTESIAN_POINT('Ctrl Pts',(-34.0393063228094,-1.97443164482047,
4.04430607188342));
#28305=CARTESIAN_POINT('Ctrl Pts',(-33.7800527604038,-2.0978954892982,3.98166126624602));
#28306=CARTESIAN_POINT('Ctrl Pts',(-33.6360054850864,-2.15356497941127,
3.95165496012834));
#28307=CARTESIAN_POINT('Ctrl Pts',(-32.8264542092776,-2.40844113561269,
3.80842697285189));
#28308=CARTESIAN_POINT('Ctrl Pts',(-31.9198836441155,-2.51838763450115,
3.72930606457842));
#28309=CARTESIAN_POINT('Ctrl Pts',(-30.5398422905574,-2.5184251275891,3.72928074525843));
#28310=CARTESIAN_POINT('Ctrl Pts',(-30.08496400456,-2.49151823506772,3.74784410583648));
#28311=CARTESIAN_POINT('Ctrl Pts',(-29.2362644769754,-2.38522561970891,
3.81637226963152));
#28312=CARTESIAN_POINT('Ctrl Pts',(-28.8469549569745,-2.30566301000398,
3.86618542447976));
#28313=CARTESIAN_POINT('Ctrl Pts',(-28.3649107668198,-2.15388373878846,
3.95147475669815));
#28314=CARTESIAN_POINT('Ctrl Pts',(-28.2228041159262,-2.09926959675711,
3.98096555586596));
#28315=CARTESIAN_POINT('Ctrl Pts',(-28.0241068899402,-2.0044965746748,4.02905055581734));
#28316=CARTESIAN_POINT('Ctrl Pts',(-27.9636909773592,-1.97231644998907,
4.04490878055012));
#28317=CARTESIAN_POINT('Ctrl Pts',(-27.8544921443592,-1.90676795709293,
4.07621824485302));
#28318=CARTESIAN_POINT('Ctrl Pts',(-27.8074894795624,-1.87480693010739,
4.09103914533469));
#28319=CARTESIAN_POINT('Ctrl Pts',(-27.717996119642,-1.80405959074722,4.12272619838771));
#28320=CARTESIAN_POINT('Ctrl Pts',(-27.678854738298,-1.76688965222934,4.13877771020656));
#28321=CARTESIAN_POINT('Ctrl Pts',(-27.6345827386579,-1.71546336982027,
4.16023201531108));
#28322=CARTESIAN_POINT('Ctrl Pts',(-27.6209916578288,-1.69762771350756,
4.1675483668759));
#28323=CARTESIAN_POINT('Ctrl Pts',(-27.6023544151614,-1.66982067175446,
4.17873171370946));
#28324=CARTESIAN_POINT('Ctrl Pts',(-27.596433564035,-1.66037606322677,4.18249426682801));
#28325=CARTESIAN_POINT('Ctrl Pts',(-27.5851749879742,-1.64113344454058,
4.19008209711886));
#28326=CARTESIAN_POINT('Ctrl Pts',(-27.579029173103,-1.629737911742,4.19452440771899));
#28327=CARTESIAN_POINT('Ctrl Pts',(-27.566314957399,-1.60460303135711,4.20423260339357));
#28328=CARTESIAN_POINT('Ctrl Pts',(-27.5583409045667,-1.58667844241493,
4.21104108768807));
#28329=CARTESIAN_POINT('Ctrl Pts',(-27.5471329617739,-1.55801707841301,
4.22169239332151));
#28330=CARTESIAN_POINT('Ctrl Pts',(-27.5435225035856,-1.54816752802356,
4.22531583330063));
#28331=CARTESIAN_POINT('Ctrl Pts',(-27.538295100417,-1.53294663230486,4.23085142364951));
#28332=CARTESIAN_POINT('Ctrl Pts',(-27.5365840133798,-1.5277985713604,4.23271335300807));
#28333=CARTESIAN_POINT('Ctrl Pts',(-27.5332246006767,-1.51735309651292,
4.23646909393735));
#28334=CARTESIAN_POINT('Ctrl Pts',(-27.5309269955758,-1.50989843558458,
4.2391294337564));
#28335=CARTESIAN_POINT('Ctrl Pts',(-27.521793616354,-1.47955255699408,4.24991214568788));
#28336=CARTESIAN_POINT('Ctrl Pts',(-27.5111302649714,-1.43780244931942,
4.26452955000402));
#28337=CARTESIAN_POINT('Ctrl Pts',(-27.497968043987,-1.38101342313609,4.28285042068849));
#28338=CARTESIAN_POINT('',(-27.5,-2.47065947129021,7.60893171062298));
#28339=CARTESIAN_POINT('Origin',(-27.5,0.,0.));
#28340=CARTESIAN_POINT('Origin',(-43.8559375004336,0.149957969249583,-4.29423438922274));
#28341=CARTESIAN_POINT('',(-43.9253906252168,0.1469591965737,-4.20836077533825));
#28342=CARTESIAN_POINT('',(-43.7864843756504,0.1469591965737,-4.20836077533825));
#28343=CARTESIAN_POINT('Origin',(-43.8559375004335,-3.93782229046735E-15,
8.32667268468867E-14));
#28344=CARTESIAN_POINT('Ctrl Pts',(-36.4145312504336,-0.149957969249583,
4.29423438922274));
#28345=CARTESIAN_POINT('Ctrl Pts',(-36.3880729171003,-2.62923534983068,
4.20765611530936));
#28346=CARTESIAN_POINT('Ctrl Pts',(-36.3616145837669,-3.79389505549643,
2.01724978374131));
#28347=CARTESIAN_POINT('Ctrl Pts',(-36.3351562504336,-4.95855476116219,
-0.173156547826752));
#28348=CARTESIAN_POINT('Ctrl Pts',(-36.3086979171003,-3.64393708624685,
-2.27698460548143));
#28349=CARTESIAN_POINT('Ctrl Pts',(-36.2822395837669,-2.32931941133151,
-4.38081266313611));
#28350=CARTESIAN_POINT('Ctrl Pts',(-36.2557812504336,0.149957969249583,
-4.29423438922274));
#28351=CARTESIAN_POINT('Ctrl Pts',(-36.2293229171003,2.62923534983068,-4.20765611530936));
#28352=CARTESIAN_POINT('Ctrl Pts',(-36.2028645837669,3.79389505549643,-2.0172497837413));
#28353=CARTESIAN_POINT('Ctrl Pts',(-36.1764062504336,4.95855476116219,0.173156547826753));
#28354=CARTESIAN_POINT('Ctrl Pts',(-36.1499479171003,3.64393708624685,2.27698460548143));
#28355=CARTESIAN_POINT('Ctrl Pts',(-36.1234895837669,2.32931941133151,4.38081266313611));
#28356=CARTESIAN_POINT('Ctrl Pts',(-36.0970312504336,-0.149957969249583,
4.29423438922274));
#28357=CARTESIAN_POINT('Ctrl Pts',(-36.3748437504336,-0.149957969249583,
4.29423438922274));
#28358=CARTESIAN_POINT('Ctrl Pts',(-36.3483854171003,-2.62923534983068,
4.20765611530936));
#28359=CARTESIAN_POINT('Ctrl Pts',(-36.3219270837669,-3.79389505549643,
2.01724978374131));
#28360=CARTESIAN_POINT('Ctrl Pts',(-36.2954687504336,-4.95855476116219,
-0.173156547826752));
#28361=CARTESIAN_POINT('Ctrl Pts',(-36.2690104171003,-3.64393708624685,
-2.27698460548143));
#28362=CARTESIAN_POINT('Ctrl Pts',(-36.2425520837669,-2.32931941133151,
-4.38081266313611));
#28363=CARTESIAN_POINT('Ctrl Pts',(-36.2160937504336,0.149957969249583,
-4.29423438922274));
#28364=CARTESIAN_POINT('Ctrl Pts',(-36.1896354171003,2.62923534983068,-4.20765611530936));
#28365=CARTESIAN_POINT('Ctrl Pts',(-36.1631770837669,3.79389505549644,-2.0172497837413));
#28366=CARTESIAN_POINT('Ctrl Pts',(-36.1367187504336,4.95855476116219,0.173156547826753));
#28367=CARTESIAN_POINT('Ctrl Pts',(-36.1102604171003,3.64393708624685,2.27698460548143));
#28368=CARTESIAN_POINT('Ctrl Pts',(-36.0838020837669,2.32931941133151,4.38081266313611));
#28369=CARTESIAN_POINT('Ctrl Pts',(-36.0573437504336,-0.149957969249583,
4.29423438922274));
#28370=CARTESIAN_POINT('Ctrl Pts',(-43.975,0.143960423897816,-4.12248716145376));
#28371=CARTESIAN_POINT('Ctrl Pts',(-43.9485416666667,2.52407949629392,-4.03937157196371));
#28372=CARTESIAN_POINT('Ctrl Pts',(-43.9220833333334,3.64215882054307,-1.9365701964918));
#28373=CARTESIAN_POINT('Ctrl Pts',(-43.895625,4.76023814479221,0.166231178980113));
#28374=CARTESIAN_POINT('Ctrl Pts',(-43.8691666666667,3.49819839664525,2.18591696496197));
#28375=CARTESIAN_POINT('Ctrl Pts',(-43.8427083333333,2.23615864849829,4.20560275094382));
#28376=CARTESIAN_POINT('Ctrl Pts',(-43.81625,-0.143960423897816,4.12248716145376));
#28377=CARTESIAN_POINT('Ctrl Pts',(-43.7897916666667,-2.52407949629392,
4.03937157196371));
#28378=CARTESIAN_POINT('Ctrl Pts',(-43.7633333333333,-3.64215882054307,
1.9365701964918));
#28379=CARTESIAN_POINT('Ctrl Pts',(-43.736875,-4.76023814479221,-0.166231178980113));
#28380=CARTESIAN_POINT('Ctrl Pts',(-43.7104166666667,-3.49819839664525,
-2.18591696496196));
#28381=CARTESIAN_POINT('Ctrl Pts',(-43.6839583333334,-2.23615864849829,
-4.20560275094382));
#28382=CARTESIAN_POINT('Ctrl Pts',(-43.6575,0.143960423897816,-4.12248716145376));
#28383=CARTESIAN_POINT('Ctrl Pts',(-43.6310416666667,2.52407949629392,-4.03937157196371));
#28384=CARTESIAN_POINT('Ctrl Pts',(-43.6045833333334,3.64215882054307,-1.9365701964918));
#28385=CARTESIAN_POINT('Ctrl Pts',(-43.578125,4.76023814479221,0.166231178980113));
#28386=CARTESIAN_POINT('Ctrl Pts',(-43.5516666666667,3.49819839664525,2.18591696496197));
#28387=CARTESIAN_POINT('Ctrl Pts',(-43.5252083333334,2.23615864849829,4.20560275094382));
#28388=CARTESIAN_POINT('Ctrl Pts',(-43.49875,-0.143960423897816,4.12248716145376));
#28389=CARTESIAN_POINT('Ctrl Pts',(-43.4722916666667,-2.52407949629392,
4.03937157196371));
#28390=CARTESIAN_POINT('Ctrl Pts',(-43.4458333333334,-3.64215882054307,
1.9365701964918));
#28391=CARTESIAN_POINT('Ctrl Pts',(-43.419375,-4.76023814479221,-0.166231178980113));
#28392=CARTESIAN_POINT('Ctrl Pts',(-43.3929166666667,-3.49819839664525,
-2.18591696496196));
#28393=CARTESIAN_POINT('Ctrl Pts',(-43.3664583333334,-2.23615864849829,
-4.20560275094382));
#28394=CARTESIAN_POINT('Ctrl Pts',(-43.34,0.143960423897816,-4.12248716145376));
#28395=CARTESIAN_POINT('Ctrl Pts',(-43.3135416666667,2.52407949629392,-4.03937157196371));
#28396=CARTESIAN_POINT('Ctrl Pts',(-43.2870833333333,3.64215882054307,-1.9365701964918));
#28397=CARTESIAN_POINT('Ctrl Pts',(-43.260625,4.76023814479221,0.166231178980113));
#28398=CARTESIAN_POINT('Ctrl Pts',(-43.2341666666667,3.49819839664525,2.18591696496197));
#28399=CARTESIAN_POINT('Ctrl Pts',(-43.2077083333333,2.23615864849829,4.20560275094382));
#28400=CARTESIAN_POINT('Ctrl Pts',(-43.18125,-0.143960423897816,4.12248716145376));
#28401=CARTESIAN_POINT('Ctrl Pts',(-43.1547916666667,-2.52407949629392,
4.03937157196371));
#28402=CARTESIAN_POINT('Ctrl Pts',(-43.1283333333333,-3.64215882054307,
1.9365701964918));
#28403=CARTESIAN_POINT('Ctrl Pts',(-43.101875,-4.76023814479221,-0.166231178980113));
#28404=CARTESIAN_POINT('Ctrl Pts',(-43.0754166666667,-3.49819839664525,
-2.18591696496196));
#28405=CARTESIAN_POINT('Ctrl Pts',(-43.0489583333333,-2.23615864849829,
-4.20560275094382));
#28406=CARTESIAN_POINT('Ctrl Pts',(-43.0225,0.143960423897816,-4.12248716145376));
#28407=CARTESIAN_POINT('Ctrl Pts',(-42.9960416666667,2.52407949629392,-4.03937157196371));
#28408=CARTESIAN_POINT('Ctrl Pts',(-42.9695833333334,3.64215882054307,-1.9365701964918));
#28409=CARTESIAN_POINT('Ctrl Pts',(-42.943125,4.76023814479221,0.166231178980113));
#28410=CARTESIAN_POINT('Ctrl Pts',(-42.9166666666667,3.49819839664525,2.18591696496197));
#28411=CARTESIAN_POINT('Ctrl Pts',(-42.8902083333333,2.23615864849829,4.20560275094382));
#28412=CARTESIAN_POINT('Ctrl Pts',(-42.86375,-0.143960423897816,4.12248716145376));
#28413=CARTESIAN_POINT('Ctrl Pts',(-42.8372916666667,-2.52407949629392,
4.03937157196371));
#28414=CARTESIAN_POINT('Ctrl Pts',(-42.8108333333333,-3.64215882054307,
1.9365701964918));
#28415=CARTESIAN_POINT('Ctrl Pts',(-42.784375,-4.76023814479221,-0.166231178980113));
#28416=CARTESIAN_POINT('Ctrl Pts',(-42.7579166666667,-3.49819839664525,
-2.18591696496196));
#28417=CARTESIAN_POINT('Ctrl Pts',(-42.7314583333334,-2.23615864849829,
-4.20560275094382));
#28418=CARTESIAN_POINT('Ctrl Pts',(-42.705,0.143960423897816,-4.12248716145376));
#28419=CARTESIAN_POINT('Ctrl Pts',(-42.6785416666667,2.52407949629392,-4.03937157196371));
#28420=CARTESIAN_POINT('Ctrl Pts',(-42.6520833333333,3.64215882054307,-1.9365701964918));
#28421=CARTESIAN_POINT('Ctrl Pts',(-42.625625,4.76023814479221,0.166231178980113));
#28422=CARTESIAN_POINT('Ctrl Pts',(-42.5991666666667,3.49819839664525,2.18591696496197));
#28423=CARTESIAN_POINT('Ctrl Pts',(-42.5727083333334,2.23615864849829,4.20560275094382));
#28424=CARTESIAN_POINT('Ctrl Pts',(-42.54625,-0.143960423897816,4.12248716145376));
#28425=CARTESIAN_POINT('Ctrl Pts',(-42.5197916666667,-2.52407949629392,
4.03937157196371));
#28426=CARTESIAN_POINT('Ctrl Pts',(-42.4933333333334,-3.64215882054307,
1.9365701964918));
#28427=CARTESIAN_POINT('Ctrl Pts',(-42.466875,-4.76023814479221,-0.166231178980113));
#28428=CARTESIAN_POINT('Ctrl Pts',(-42.4404166666667,-3.49819839664525,
-2.18591696496196));
#28429=CARTESIAN_POINT('Ctrl Pts',(-42.4139583333333,-2.23615864849829,
-4.20560275094382));
#28430=CARTESIAN_POINT('Ctrl Pts',(-42.3875,0.143960423897816,-4.12248716145376));
#28431=CARTESIAN_POINT('Ctrl Pts',(-42.3610416666667,2.52407949629392,-4.03937157196371));
#28432=CARTESIAN_POINT('Ctrl Pts',(-42.3345833333333,3.64215882054307,-1.9365701964918));
#28433=CARTESIAN_POINT('Ctrl Pts',(-42.308125,4.76023814479221,0.166231178980113));
#28434=CARTESIAN_POINT('Ctrl Pts',(-42.2816666666667,3.49819839664525,2.18591696496197));
#28435=CARTESIAN_POINT('Ctrl Pts',(-42.2552083333333,2.23615864849829,4.20560275094382));
#28436=CARTESIAN_POINT('Ctrl Pts',(-42.22875,-0.143960423897816,4.12248716145376));
#28437=CARTESIAN_POINT('Ctrl Pts',(-42.2022916666667,-2.52407949629392,
4.03937157196371));
#28438=CARTESIAN_POINT('Ctrl Pts',(-42.1758333333334,-3.64215882054307,
1.9365701964918));
#28439=CARTESIAN_POINT('Ctrl Pts',(-42.149375,-4.76023814479221,-0.166231178980113));
#28440=CARTESIAN_POINT('Ctrl Pts',(-42.1229166666667,-3.49819839664525,
-2.18591696496196));
#28441=CARTESIAN_POINT('Ctrl Pts',(-42.0964583333333,-2.23615864849829,
-4.20560275094382));
#28442=CARTESIAN_POINT('Ctrl Pts',(-42.07,0.143960423897816,-4.12248716145376));
#28443=CARTESIAN_POINT('Ctrl Pts',(-42.0435416666667,2.52407949629392,-4.03937157196371));
#28444=CARTESIAN_POINT('Ctrl Pts',(-42.0170833333334,3.64215882054307,-1.9365701964918));
#28445=CARTESIAN_POINT('Ctrl Pts',(-41.990625,4.76023814479221,0.166231178980113));
#28446=CARTESIAN_POINT('Ctrl Pts',(-41.9641666666667,3.49819839664525,2.18591696496197));
#28447=CARTESIAN_POINT('Ctrl Pts',(-41.9377083333333,2.23615864849829,4.20560275094382));
#28448=CARTESIAN_POINT('Ctrl Pts',(-41.91125,-0.143960423897816,4.12248716145376));
#28449=CARTESIAN_POINT('Ctrl Pts',(-41.8847916666667,-2.52407949629392,
4.03937157196371));
#28450=CARTESIAN_POINT('Ctrl Pts',(-41.8583333333333,-3.64215882054307,
1.9365701964918));
#28451=CARTESIAN_POINT('Ctrl Pts',(-41.831875,-4.76023814479221,-0.166231178980113));
#28452=CARTESIAN_POINT('Ctrl Pts',(-41.8054166666667,-3.49819839664525,
-2.18591696496196));
#28453=CARTESIAN_POINT('Ctrl Pts',(-41.7789583333333,-2.23615864849829,
-4.20560275094382));
#28454=CARTESIAN_POINT('Ctrl Pts',(-41.7525,0.143960423897816,-4.12248716145376));
#28455=CARTESIAN_POINT('Ctrl Pts',(-41.7260416666667,2.52407949629392,-4.03937157196371));
#28456=CARTESIAN_POINT('Ctrl Pts',(-41.6995833333333,3.64215882054307,-1.9365701964918));
#28457=CARTESIAN_POINT('Ctrl Pts',(-41.673125,4.76023814479221,0.166231178980113));
#28458=CARTESIAN_POINT('Ctrl Pts',(-41.6466666666667,3.49819839664525,2.18591696496197));
#28459=CARTESIAN_POINT('Ctrl Pts',(-41.6202083333334,2.23615864849829,4.20560275094382));
#28460=CARTESIAN_POINT('Ctrl Pts',(-41.59375,-0.143960423897816,4.12248716145376));
#28461=CARTESIAN_POINT('Ctrl Pts',(-41.5672916666667,-2.52407949629392,
4.03937157196371));
#28462=CARTESIAN_POINT('Ctrl Pts',(-41.5408333333334,-3.64215882054307,
1.9365701964918));
#28463=CARTESIAN_POINT('Ctrl Pts',(-41.514375,-4.76023814479221,-0.166231178980113));
#28464=CARTESIAN_POINT('Ctrl Pts',(-41.4879166666667,-3.49819839664525,
-2.18591696496196));
#28465=CARTESIAN_POINT('Ctrl Pts',(-41.4614583333333,-2.23615864849829,
-4.20560275094382));
#28466=CARTESIAN_POINT('Ctrl Pts',(-41.435,0.143960423897816,-4.12248716145376));
#28467=CARTESIAN_POINT('Ctrl Pts',(-41.4085416666667,2.52407949629392,-4.03937157196371));
#28468=CARTESIAN_POINT('Ctrl Pts',(-41.3820833333333,3.64215882054307,-1.9365701964918));
#28469=CARTESIAN_POINT('Ctrl Pts',(-41.355625,4.76023814479221,0.166231178980113));
#28470=CARTESIAN_POINT('Ctrl Pts',(-41.3291666666667,3.49819839664525,2.18591696496197));
#28471=CARTESIAN_POINT('Ctrl Pts',(-41.3027083333333,2.23615864849829,4.20560275094382));
#28472=CARTESIAN_POINT('Ctrl Pts',(-41.27625,-0.143960423897816,4.12248716145376));
#28473=CARTESIAN_POINT('Ctrl Pts',(-41.2497916666667,-2.52407949629392,
4.03937157196371));
#28474=CARTESIAN_POINT('Ctrl Pts',(-41.2233333333334,-3.64215882054307,
1.9365701964918));
#28475=CARTESIAN_POINT('Ctrl Pts',(-41.196875,-4.76023814479221,-0.166231178980113));
#28476=CARTESIAN_POINT('Ctrl Pts',(-41.1704166666667,-3.49819839664525,
-2.18591696496196));
#28477=CARTESIAN_POINT('Ctrl Pts',(-41.1439583333334,-2.23615864849829,
-4.20560275094382));
#28478=CARTESIAN_POINT('Ctrl Pts',(-41.1175,0.143960423897816,-4.12248716145376));
#28479=CARTESIAN_POINT('Ctrl Pts',(-41.0910416666667,2.52407949629392,-4.03937157196371));
#28480=CARTESIAN_POINT('Ctrl Pts',(-41.0645833333334,3.64215882054307,-1.9365701964918));
#28481=CARTESIAN_POINT('Ctrl Pts',(-41.038125,4.76023814479221,0.166231178980113));
#28482=CARTESIAN_POINT('Ctrl Pts',(-41.0116666666667,3.49819839664525,2.18591696496197));
#28483=CARTESIAN_POINT('Ctrl Pts',(-40.9852083333334,2.23615864849829,4.20560275094382));
#28484=CARTESIAN_POINT('Ctrl Pts',(-40.95875,-0.143960423897816,4.12248716145376));
#28485=CARTESIAN_POINT('Ctrl Pts',(-40.9322916666667,-2.52407949629392,
4.03937157196371));
#28486=CARTESIAN_POINT('Ctrl Pts',(-40.9058333333333,-3.64215882054307,
1.9365701964918));
#28487=CARTESIAN_POINT('Ctrl Pts',(-40.879375,-4.76023814479221,-0.166231178980113));
#28488=CARTESIAN_POINT('Ctrl Pts',(-40.8529166666667,-3.49819839664525,
-2.18591696496196));
#28489=CARTESIAN_POINT('Ctrl Pts',(-40.8264583333333,-2.23615864849829,
-4.20560275094382));
#28490=CARTESIAN_POINT('Ctrl Pts',(-40.8,0.143960423897816,-4.12248716145376));
#28491=CARTESIAN_POINT('Ctrl Pts',(-40.7735416666667,2.52407949629392,-4.03937157196371));
#28492=CARTESIAN_POINT('Ctrl Pts',(-40.7470833333333,3.64215882054307,-1.9365701964918));
#28493=CARTESIAN_POINT('Ctrl Pts',(-40.720625,4.76023814479221,0.166231178980113));
#28494=CARTESIAN_POINT('Ctrl Pts',(-40.6941666666667,3.49819839664525,2.18591696496197));
#28495=CARTESIAN_POINT('Ctrl Pts',(-40.6677083333334,2.23615864849829,4.20560275094382));
#28496=CARTESIAN_POINT('Ctrl Pts',(-40.64125,-0.143960423897816,4.12248716145376));
#28497=CARTESIAN_POINT('Ctrl Pts',(-40.6147916666667,-2.52407949629392,
4.03937157196371));
#28498=CARTESIAN_POINT('Ctrl Pts',(-40.5883333333334,-3.64215882054307,
1.9365701964918));
#28499=CARTESIAN_POINT('Ctrl Pts',(-40.561875,-4.76023814479221,-0.166231178980113));
#28500=CARTESIAN_POINT('Ctrl Pts',(-40.5354166666667,-3.49819839664525,
-2.18591696496196));
#28501=CARTESIAN_POINT('Ctrl Pts',(-40.5089583333333,-2.23615864849829,
-4.20560275094382));
#28502=CARTESIAN_POINT('Ctrl Pts',(-40.4825,0.143960423897816,-4.12248716145376));
#28503=CARTESIAN_POINT('Ctrl Pts',(-40.4560416666667,2.52407949629392,-4.03937157196371));
#28504=CARTESIAN_POINT('Ctrl Pts',(-40.4295833333333,3.64215882054307,-1.9365701964918));
#28505=CARTESIAN_POINT('Ctrl Pts',(-40.403125,4.76023814479221,0.166231178980113));
#28506=CARTESIAN_POINT('Ctrl Pts',(-40.3766666666667,3.49819839664525,2.18591696496197));
#28507=CARTESIAN_POINT('Ctrl Pts',(-40.3502083333333,2.23615864849829,4.20560275094382));
#28508=CARTESIAN_POINT('Ctrl Pts',(-40.32375,-0.143960423897816,4.12248716145376));
#28509=CARTESIAN_POINT('Ctrl Pts',(-40.2972916666667,-2.52407949629392,
4.03937157196371));
#28510=CARTESIAN_POINT('Ctrl Pts',(-40.2708333333333,-3.64215882054307,
1.9365701964918));
#28511=CARTESIAN_POINT('Ctrl Pts',(-40.244375,-4.76023814479221,-0.166231178980113));
#28512=CARTESIAN_POINT('Ctrl Pts',(-40.2179166666667,-3.49819839664525,
-2.18591696496196));
#28513=CARTESIAN_POINT('Ctrl Pts',(-40.1914583333333,-2.23615864849829,
-4.20560275094382));
#28514=CARTESIAN_POINT('Ctrl Pts',(-40.165,0.143960423897816,-4.12248716145376));
#28515=CARTESIAN_POINT('Ctrl Pts',(-40.1385416666667,2.52407949629392,-4.03937157196371));
#28516=CARTESIAN_POINT('Ctrl Pts',(-40.1120833333334,3.64215882054307,-1.9365701964918));
#28517=CARTESIAN_POINT('Ctrl Pts',(-40.085625,4.76023814479221,0.166231178980113));
#28518=CARTESIAN_POINT('Ctrl Pts',(-40.0591666666667,3.49819839664525,2.18591696496197));
#28519=CARTESIAN_POINT('Ctrl Pts',(-40.0327083333333,2.23615864849829,4.20560275094382));
#28520=CARTESIAN_POINT('Ctrl Pts',(-40.00625,-0.143960423897816,4.12248716145376));
#28521=CARTESIAN_POINT('Ctrl Pts',(-39.9797916666667,-2.52407949629392,
4.03937157196371));
#28522=CARTESIAN_POINT('Ctrl Pts',(-39.9533333333333,-3.64215882054307,
1.9365701964918));
#28523=CARTESIAN_POINT('Ctrl Pts',(-39.926875,-4.76023814479221,-0.166231178980113));
#28524=CARTESIAN_POINT('Ctrl Pts',(-39.9004166666667,-3.49819839664525,
-2.18591696496196));
#28525=CARTESIAN_POINT('Ctrl Pts',(-39.8739583333333,-2.23615864849829,
-4.20560275094382));
#28526=CARTESIAN_POINT('Ctrl Pts',(-39.8475,0.143960423897816,-4.12248716145376));
#28527=CARTESIAN_POINT('Ctrl Pts',(-39.8210416666667,2.52407949629392,-4.03937157196371));
#28528=CARTESIAN_POINT('Ctrl Pts',(-39.7945833333333,3.64215882054307,-1.9365701964918));
#28529=CARTESIAN_POINT('Ctrl Pts',(-39.768125,4.76023814479221,0.166231178980113));
#28530=CARTESIAN_POINT('Ctrl Pts',(-39.7416666666667,3.49819839664525,2.18591696496197));
#28531=CARTESIAN_POINT('Ctrl Pts',(-39.7152083333334,2.23615864849829,4.20560275094382));
#28532=CARTESIAN_POINT('Ctrl Pts',(-39.68875,-0.143960423897816,4.12248716145376));
#28533=CARTESIAN_POINT('Ctrl Pts',(-39.6622916666667,-2.52407949629392,
4.03937157196371));
#28534=CARTESIAN_POINT('Ctrl Pts',(-39.6358333333333,-3.64215882054307,
1.9365701964918));
#28535=CARTESIAN_POINT('Ctrl Pts',(-39.609375,-4.76023814479221,-0.166231178980113));
#28536=CARTESIAN_POINT('Ctrl Pts',(-39.5829166666667,-3.49819839664525,
-2.18591696496196));
#28537=CARTESIAN_POINT('Ctrl Pts',(-39.5564583333333,-2.23615864849829,
-4.20560275094382));
#28538=CARTESIAN_POINT('Ctrl Pts',(-39.53,0.143960423897816,-4.12248716145376));
#28539=CARTESIAN_POINT('Ctrl Pts',(-39.5035416666667,2.52407949629392,-4.03937157196371));
#28540=CARTESIAN_POINT('Ctrl Pts',(-39.4770833333333,3.64215882054307,-1.9365701964918));
#28541=CARTESIAN_POINT('Ctrl Pts',(-39.450625,4.76023814479221,0.166231178980113));
#28542=CARTESIAN_POINT('Ctrl Pts',(-39.4241666666667,3.49819839664525,2.18591696496197));
#28543=CARTESIAN_POINT('Ctrl Pts',(-39.3977083333333,2.23615864849829,4.20560275094382));
#28544=CARTESIAN_POINT('Ctrl Pts',(-39.37125,-0.143960423897816,4.12248716145376));
#28545=CARTESIAN_POINT('Ctrl Pts',(-39.3447916666667,-2.52407949629392,
4.03937157196371));
#28546=CARTESIAN_POINT('Ctrl Pts',(-39.3183333333333,-3.64215882054307,
1.9365701964918));
#28547=CARTESIAN_POINT('Ctrl Pts',(-39.291875,-4.76023814479221,-0.166231178980113));
#28548=CARTESIAN_POINT('Ctrl Pts',(-39.2654166666667,-3.49819839664525,
-2.18591696496196));
#28549=CARTESIAN_POINT('Ctrl Pts',(-39.2389583333333,-2.23615864849829,
-4.20560275094382));
#28550=CARTESIAN_POINT('Ctrl Pts',(-39.2125,0.143960423897816,-4.12248716145376));
#28551=CARTESIAN_POINT('Ctrl Pts',(-39.1860416666667,2.52407949629392,-4.03937157196371));
#28552=CARTESIAN_POINT('Ctrl Pts',(-39.1595833333333,3.64215882054307,-1.9365701964918));
#28553=CARTESIAN_POINT('Ctrl Pts',(-39.133125,4.76023814479221,0.166231178980113));
#28554=CARTESIAN_POINT('Ctrl Pts',(-39.1066666666667,3.49819839664525,2.18591696496197));
#28555=CARTESIAN_POINT('Ctrl Pts',(-39.0802083333333,2.23615864849829,4.20560275094382));
#28556=CARTESIAN_POINT('Ctrl Pts',(-39.05375,-0.143960423897816,4.12248716145376));
#28557=CARTESIAN_POINT('Ctrl Pts',(-39.0272916666667,-2.52407949629392,
4.03937157196371));
#28558=CARTESIAN_POINT('Ctrl Pts',(-39.0008333333333,-3.64215882054307,
1.9365701964918));
#28559=CARTESIAN_POINT('Ctrl Pts',(-38.974375,-4.76023814479221,-0.166231178980113));
#28560=CARTESIAN_POINT('Ctrl Pts',(-38.9479166666667,-3.49819839664525,
-2.18591696496196));
#28561=CARTESIAN_POINT('Ctrl Pts',(-38.9214583333333,-2.23615864849829,
-4.20560275094382));
#28562=CARTESIAN_POINT('Ctrl Pts',(-38.895,0.143960423897816,-4.12248716145376));
#28563=CARTESIAN_POINT('Ctrl Pts',(-38.8685416666667,2.52407949629392,-4.03937157196371));
#28564=CARTESIAN_POINT('Ctrl Pts',(-38.8420833333333,3.64215882054307,-1.9365701964918));
#28565=CARTESIAN_POINT('Ctrl Pts',(-38.815625,4.76023814479221,0.166231178980113));
#28566=CARTESIAN_POINT('Ctrl Pts',(-38.7891666666667,3.49819839664525,2.18591696496197));
#28567=CARTESIAN_POINT('Ctrl Pts',(-38.7627083333334,2.23615864849829,4.20560275094382));
#28568=CARTESIAN_POINT('Ctrl Pts',(-38.73625,-0.143960423897816,4.12248716145376));
#28569=CARTESIAN_POINT('Ctrl Pts',(-38.7097916666667,-2.52407949629392,
4.03937157196371));
#28570=CARTESIAN_POINT('Ctrl Pts',(-38.6833333333333,-3.64215882054307,
1.9365701964918));
#28571=CARTESIAN_POINT('Ctrl Pts',(-38.656875,-4.76023814479221,-0.166231178980113));
#28572=CARTESIAN_POINT('Ctrl Pts',(-38.6304166666667,-3.49819839664525,
-2.18591696496196));
#28573=CARTESIAN_POINT('Ctrl Pts',(-38.6039583333333,-2.23615864849829,
-4.20560275094382));
#28574=CARTESIAN_POINT('Ctrl Pts',(-38.5775,0.143960423897816,-4.12248716145376));
#28575=CARTESIAN_POINT('Ctrl Pts',(-38.5510416666667,2.52407949629392,-4.03937157196371));
#28576=CARTESIAN_POINT('Ctrl Pts',(-38.5245833333333,3.64215882054307,-1.9365701964918));
#28577=CARTESIAN_POINT('Ctrl Pts',(-38.498125,4.76023814479221,0.166231178980113));
#28578=CARTESIAN_POINT('Ctrl Pts',(-38.4716666666667,3.49819839664525,2.18591696496197));
#28579=CARTESIAN_POINT('Ctrl Pts',(-38.4452083333333,2.23615864849829,4.20560275094382));
#28580=CARTESIAN_POINT('Ctrl Pts',(-38.41875,-0.143960423897816,4.12248716145376));
#28581=CARTESIAN_POINT('Ctrl Pts',(-38.3922916666667,-2.52407949629392,
4.03937157196371));
#28582=CARTESIAN_POINT('Ctrl Pts',(-38.3658333333334,-3.64215882054307,
1.9365701964918));
#28583=CARTESIAN_POINT('Ctrl Pts',(-38.339375,-4.76023814479221,-0.166231178980113));
#28584=CARTESIAN_POINT('Ctrl Pts',(-38.3129166666667,-3.49819839664525,
-2.18591696496196));
#28585=CARTESIAN_POINT('Ctrl Pts',(-38.2864583333333,-2.23615864849829,
-4.20560275094382));
#28586=CARTESIAN_POINT('Ctrl Pts',(-38.26,0.143960423897816,-4.12248716145376));
#28587=CARTESIAN_POINT('Ctrl Pts',(-38.2335416666667,2.52407949629392,-4.03937157196371));
#28588=CARTESIAN_POINT('Ctrl Pts',(-38.2070833333333,3.64215882054307,-1.9365701964918));
#28589=CARTESIAN_POINT('Ctrl Pts',(-38.180625,4.76023814479221,0.166231178980113));
#28590=CARTESIAN_POINT('Ctrl Pts',(-38.1541666666667,3.49819839664525,2.18591696496197));
#28591=CARTESIAN_POINT('Ctrl Pts',(-38.1277083333333,2.23615864849829,4.20560275094382));
#28592=CARTESIAN_POINT('Ctrl Pts',(-38.10125,-0.143960423897816,4.12248716145376));
#28593=CARTESIAN_POINT('Ctrl Pts',(-38.0747916666667,-2.52407949629392,
4.03937157196371));
#28594=CARTESIAN_POINT('Ctrl Pts',(-38.0483333333333,-3.64215882054307,
1.9365701964918));
#28595=CARTESIAN_POINT('Ctrl Pts',(-38.021875,-4.76023814479221,-0.166231178980113));
#28596=CARTESIAN_POINT('Ctrl Pts',(-37.9954166666667,-3.49819839664525,
-2.18591696496196));
#28597=CARTESIAN_POINT('Ctrl Pts',(-37.9689583333333,-2.23615864849829,
-4.20560275094382));
#28598=CARTESIAN_POINT('Ctrl Pts',(-37.9425,0.143960423897816,-4.12248716145376));
#28599=CARTESIAN_POINT('Ctrl Pts',(-37.9160416666667,2.52407949629392,-4.03937157196371));
#28600=CARTESIAN_POINT('Ctrl Pts',(-37.8895833333333,3.64215882054307,-1.9365701964918));
#28601=CARTESIAN_POINT('Ctrl Pts',(-37.863125,4.76023814479221,0.166231178980113));
#28602=CARTESIAN_POINT('Ctrl Pts',(-37.8366666666667,3.49819839664525,2.18591696496197));
#28603=CARTESIAN_POINT('Ctrl Pts',(-37.8102083333333,2.23615864849829,4.20560275094382));
#28604=CARTESIAN_POINT('Ctrl Pts',(-37.78375,-0.143960423897816,4.12248716145376));
#28605=CARTESIAN_POINT('Ctrl Pts',(-37.7572916666667,-2.52407949629392,
4.03937157196371));
#28606=CARTESIAN_POINT('Ctrl Pts',(-37.7308333333333,-3.64215882054307,
1.9365701964918));
#28607=CARTESIAN_POINT('Ctrl Pts',(-37.704375,-4.76023814479221,-0.166231178980113));
#28608=CARTESIAN_POINT('Ctrl Pts',(-37.6779166666667,-3.49819839664525,
-2.18591696496196));
#28609=CARTESIAN_POINT('Ctrl Pts',(-37.6514583333333,-2.23615864849829,
-4.20560275094382));
#28610=CARTESIAN_POINT('Ctrl Pts',(-37.625,0.143960423897816,-4.12248716145376));
#28611=CARTESIAN_POINT('Ctrl Pts',(-37.5985416666667,2.52407949629392,-4.03937157196371));
#28612=CARTESIAN_POINT('Ctrl Pts',(-37.5720833333333,3.64215882054307,-1.9365701964918));
#28613=CARTESIAN_POINT('Ctrl Pts',(-37.545625,4.76023814479221,0.166231178980113));
#28614=CARTESIAN_POINT('Ctrl Pts',(-37.5191666666667,3.49819839664525,2.18591696496197));
#28615=CARTESIAN_POINT('Ctrl Pts',(-37.4927083333333,2.23615864849829,4.20560275094382));
#28616=CARTESIAN_POINT('Ctrl Pts',(-37.46625,-0.143960423897816,4.12248716145376));
#28617=CARTESIAN_POINT('Ctrl Pts',(-37.4397916666667,-2.52407949629392,
4.03937157196371));
#28618=CARTESIAN_POINT('Ctrl Pts',(-37.4133333333334,-3.64215882054307,
1.9365701964918));
#28619=CARTESIAN_POINT('Ctrl Pts',(-37.386875,-4.76023814479221,-0.166231178980113));
#28620=CARTESIAN_POINT('Ctrl Pts',(-37.3604166666667,-3.49819839664525,
-2.18591696496196));
#28621=CARTESIAN_POINT('Ctrl Pts',(-37.3339583333333,-2.23615864849829,
-4.20560275094382));
#28622=CARTESIAN_POINT('Ctrl Pts',(-37.3075,0.143960423897816,-4.12248716145376));
#28623=CARTESIAN_POINT('Ctrl Pts',(-37.2810416666667,2.52407949629392,-4.03937157196371));
#28624=CARTESIAN_POINT('Ctrl Pts',(-37.2545833333334,3.64215882054307,-1.9365701964918));
#28625=CARTESIAN_POINT('Ctrl Pts',(-37.228125,4.76023814479221,0.166231178980113));
#28626=CARTESIAN_POINT('Ctrl Pts',(-37.2016666666667,3.49819839664525,2.18591696496197));
#28627=CARTESIAN_POINT('Ctrl Pts',(-37.1752083333334,2.23615864849829,4.20560275094382));
#28628=CARTESIAN_POINT('Ctrl Pts',(-37.14875,-0.143960423897816,4.12248716145376));
#28629=CARTESIAN_POINT('Ctrl Pts',(-37.1222916666667,-2.52407949629392,
4.03937157196371));
#28630=CARTESIAN_POINT('Ctrl Pts',(-37.0958333333333,-3.64215882054307,
1.9365701964918));
#28631=CARTESIAN_POINT('Ctrl Pts',(-37.069375,-4.76023814479221,-0.166231178980113));
#28632=CARTESIAN_POINT('Ctrl Pts',(-37.0429166666667,-3.49819839664525,
-2.18591696496196));
#28633=CARTESIAN_POINT('Ctrl Pts',(-37.0164583333333,-2.23615864849829,
-4.20560275094382));
#28634=CARTESIAN_POINT('Ctrl Pts',(-36.99,0.143960423897816,-4.12248716145376));
#28635=CARTESIAN_POINT('Ctrl Pts',(-36.9635416666667,2.52407949629392,-4.03937157196371));
#28636=CARTESIAN_POINT('Ctrl Pts',(-36.9370833333333,3.64215882054307,-1.9365701964918));
#28637=CARTESIAN_POINT('Ctrl Pts',(-36.910625,4.76023814479221,0.166231178980113));
#28638=CARTESIAN_POINT('Ctrl Pts',(-36.8841666666667,3.49819839664525,2.18591696496197));
#28639=CARTESIAN_POINT('Ctrl Pts',(-36.8577083333333,2.23615864849829,4.20560275094382));
#28640=CARTESIAN_POINT('Ctrl Pts',(-36.83125,-0.143960423897816,4.12248716145376));
#28641=CARTESIAN_POINT('Ctrl Pts',(-36.8047916666667,-2.52407949629392,
4.03937157196371));
#28642=CARTESIAN_POINT('Ctrl Pts',(-36.7783333333333,-3.64215882054307,
1.9365701964918));
#28643=CARTESIAN_POINT('Ctrl Pts',(-36.751875,-4.76023814479221,-0.166231178980113));
#28644=CARTESIAN_POINT('Ctrl Pts',(-36.7254166666667,-3.49819839664525,
-2.18591696496196));
#28645=CARTESIAN_POINT('Ctrl Pts',(-36.6989583333333,-2.23615864849829,
-4.20560275094382));
#28646=CARTESIAN_POINT('Ctrl Pts',(-36.6725,0.143960423897816,-4.12248716145376));
#28647=CARTESIAN_POINT('Ctrl Pts',(-36.6460416666667,2.52407949629392,-4.03937157196371));
#28648=CARTESIAN_POINT('Ctrl Pts',(-36.6195833333333,3.64215882054307,-1.9365701964918));
#28649=CARTESIAN_POINT('Ctrl Pts',(-36.593125,4.76023814479221,0.166231178980113));
#28650=CARTESIAN_POINT('Ctrl Pts',(-36.5666666666667,3.49819839664525,2.18591696496197));
#28651=CARTESIAN_POINT('Ctrl Pts',(-36.5402083333333,2.23615864849829,4.20560275094382));
#28652=CARTESIAN_POINT('Ctrl Pts',(-36.51375,-0.143960423897816,4.12248716145376));
#28653=CARTESIAN_POINT('Ctrl Pts',(-36.4872916666667,-2.52407949629392,
4.03937157196371));
#28654=CARTESIAN_POINT('Ctrl Pts',(-36.4608333333334,-3.64215882054307,
1.9365701964918));
#28655=CARTESIAN_POINT('Ctrl Pts',(-36.434375,-4.76023814479221,-0.166231178980113));
#28656=CARTESIAN_POINT('Ctrl Pts',(-36.4079166666667,-3.49819839664525,
-2.18591696496196));
#28657=CARTESIAN_POINT('Ctrl Pts',(-36.3814583333333,-2.23615864849829,
-4.20560275094382));
#28658=CARTESIAN_POINT('Ctrl Pts',(-36.355,0.143960423897816,-4.12248716145376));
#28659=CARTESIAN_POINT('Ctrl Pts',(-36.3285416666667,2.52407949629392,-4.03937157196371));
#28660=CARTESIAN_POINT('Ctrl Pts',(-36.3020833333333,3.64215882054307,-1.9365701964918));
#28661=CARTESIAN_POINT('Ctrl Pts',(-36.275625,4.76023814479221,0.166231178980113));
#28662=CARTESIAN_POINT('Ctrl Pts',(-36.2491666666667,3.49819839664525,2.18591696496197));
#28663=CARTESIAN_POINT('Ctrl Pts',(-36.2227083333333,2.23615864849829,4.20560275094382));
#28664=CARTESIAN_POINT('Ctrl Pts',(-36.19625,-0.143960423897816,4.12248716145376));
#28665=CARTESIAN_POINT('Ctrl Pts',(-36.1697916666667,-2.52407949629392,
4.03937157196371));
#28666=CARTESIAN_POINT('Ctrl Pts',(-36.1433333333333,-3.64215882054307,
1.9365701964918));
#28667=CARTESIAN_POINT('Ctrl Pts',(-36.116875,-4.76023814479221,-0.166231178980113));
#28668=CARTESIAN_POINT('Ctrl Pts',(-36.0904166666667,-3.49819839664525,
-2.18591696496196));
#28669=CARTESIAN_POINT('Ctrl Pts',(-36.0639583333334,-2.23615864849829,
-4.20560275094382));
#28670=CARTESIAN_POINT('Ctrl Pts',(-36.0375,0.143960423897816,-4.12248716145376));
#28671=CARTESIAN_POINT('Ctrl Pts',(-36.0110416666667,2.52407949629392,-4.03937157196371));
#28672=CARTESIAN_POINT('Ctrl Pts',(-35.9845833333333,3.64215882054307,-1.9365701964918));
#28673=CARTESIAN_POINT('Ctrl Pts',(-35.958125,4.76023814479221,0.166231178980113));
#28674=CARTESIAN_POINT('Ctrl Pts',(-35.9316666666667,3.49819839664525,2.18591696496197));
#28675=CARTESIAN_POINT('Ctrl Pts',(-35.9052083333333,2.23615864849829,4.20560275094382));
#28676=CARTESIAN_POINT('Ctrl Pts',(-35.87875,-0.143960423897816,4.12248716145376));
#28677=CARTESIAN_POINT('Ctrl Pts',(-35.8522916666667,-2.52407949629392,
4.03937157196371));
#28678=CARTESIAN_POINT('Ctrl Pts',(-35.8258333333333,-3.64215882054307,
1.9365701964918));
#28679=CARTESIAN_POINT('Ctrl Pts',(-35.799375,-4.76023814479221,-0.166231178980113));
#28680=CARTESIAN_POINT('Ctrl Pts',(-35.7729166666667,-3.49819839664525,
-2.18591696496196));
#28681=CARTESIAN_POINT('Ctrl Pts',(-35.7464583333333,-2.23615864849829,
-4.20560275094382));
#28682=CARTESIAN_POINT('Ctrl Pts',(-35.72,0.143960423897816,-4.12248716145376));
#28683=CARTESIAN_POINT('Ctrl Pts',(-35.6935416666667,2.52407949629392,-4.03937157196371));
#28684=CARTESIAN_POINT('Ctrl Pts',(-35.6670833333334,3.64215882054307,-1.9365701964918));
#28685=CARTESIAN_POINT('Ctrl Pts',(-35.640625,4.76023814479221,0.166231178980113));
#28686=CARTESIAN_POINT('Ctrl Pts',(-35.6141666666667,3.49819839664525,2.18591696496197));
#28687=CARTESIAN_POINT('Ctrl Pts',(-35.5877083333333,2.23615864849829,4.20560275094382));
#28688=CARTESIAN_POINT('Ctrl Pts',(-35.56125,-0.143960423897816,4.12248716145376));
#28689=CARTESIAN_POINT('Ctrl Pts',(-35.5347916666667,-2.52407949629392,
4.03937157196371));
#28690=CARTESIAN_POINT('Ctrl Pts',(-35.5083333333333,-3.64215882054307,
1.9365701964918));
#28691=CARTESIAN_POINT('Ctrl Pts',(-35.481875,-4.76023814479221,-0.166231178980113));
#28692=CARTESIAN_POINT('Ctrl Pts',(-35.4554166666667,-3.49819839664525,
-2.18591696496196));
#28693=CARTESIAN_POINT('Ctrl Pts',(-35.4289583333333,-2.23615864849829,
-4.20560275094382));
#28694=CARTESIAN_POINT('Ctrl Pts',(-35.4025,0.143960423897816,-4.12248716145376));
#28695=CARTESIAN_POINT('Ctrl Pts',(-35.3760416666667,2.52407949629392,-4.03937157196371));
#28696=CARTESIAN_POINT('Ctrl Pts',(-35.3495833333333,3.64215882054307,-1.9365701964918));
#28697=CARTESIAN_POINT('Ctrl Pts',(-35.323125,4.76023814479221,0.166231178980113));
#28698=CARTESIAN_POINT('Ctrl Pts',(-35.2966666666667,3.49819839664525,2.18591696496197));
#28699=CARTESIAN_POINT('Ctrl Pts',(-35.2702083333333,2.23615864849829,4.20560275094382));
#28700=CARTESIAN_POINT('Ctrl Pts',(-35.24375,-0.143960423897816,4.12248716145376));
#28701=CARTESIAN_POINT('Ctrl Pts',(-35.2172916666667,-2.52407949629392,
4.03937157196371));
#28702=CARTESIAN_POINT('Ctrl Pts',(-35.1908333333333,-3.64215882054307,
1.9365701964918));
#28703=CARTESIAN_POINT('Ctrl Pts',(-35.164375,-4.76023814479221,-0.166231178980113));
#28704=CARTESIAN_POINT('Ctrl Pts',(-35.1379166666667,-3.49819839664525,
-2.18591696496196));
#28705=CARTESIAN_POINT('Ctrl Pts',(-35.1114583333333,-2.23615864849829,
-4.20560275094382));
#28706=CARTESIAN_POINT('Ctrl Pts',(-35.085,0.143960423897816,-4.12248716145376));
#28707=CARTESIAN_POINT('Ctrl Pts',(-35.0585416666667,2.52407949629392,-4.03937157196371));
#28708=CARTESIAN_POINT('Ctrl Pts',(-35.0320833333333,3.64215882054307,-1.9365701964918));
#28709=CARTESIAN_POINT('Ctrl Pts',(-35.005625,4.76023814479221,0.166231178980113));
#28710=CARTESIAN_POINT('Ctrl Pts',(-34.9791666666667,3.49819839664525,2.18591696496197));
#28711=CARTESIAN_POINT('Ctrl Pts',(-34.9527083333333,2.23615864849829,4.20560275094382));
#28712=CARTESIAN_POINT('Ctrl Pts',(-34.92625,-0.143960423897816,4.12248716145376));
#28713=CARTESIAN_POINT('Ctrl Pts',(-34.8997916666667,-2.52407949629392,
4.03937157196371));
#28714=CARTESIAN_POINT('Ctrl Pts',(-34.8733333333333,-3.64215882054307,
1.9365701964918));
#28715=CARTESIAN_POINT('Ctrl Pts',(-34.846875,-4.76023814479221,-0.166231178980113));
#28716=CARTESIAN_POINT('Ctrl Pts',(-34.8204166666667,-3.49819839664525,
-2.18591696496196));
#28717=CARTESIAN_POINT('Ctrl Pts',(-34.7939583333333,-2.23615864849829,
-4.20560275094382));
#28718=CARTESIAN_POINT('Ctrl Pts',(-34.7675,0.143960423897816,-4.12248716145376));
#28719=CARTESIAN_POINT('Ctrl Pts',(-34.7410416666667,2.52407949629392,-4.03937157196371));
#28720=CARTESIAN_POINT('Ctrl Pts',(-34.7145833333333,3.64215882054307,-1.9365701964918));
#28721=CARTESIAN_POINT('Ctrl Pts',(-34.688125,4.76023814479221,0.166231178980113));
#28722=CARTESIAN_POINT('Ctrl Pts',(-34.6616666666667,3.49819839664525,2.18591696496197));
#28723=CARTESIAN_POINT('Ctrl Pts',(-34.6352083333333,2.23615864849829,4.20560275094382));
#28724=CARTESIAN_POINT('Ctrl Pts',(-34.60875,-0.143960423897816,4.12248716145376));
#28725=CARTESIAN_POINT('Ctrl Pts',(-34.5822916666667,-2.52407949629392,
4.03937157196371));
#28726=CARTESIAN_POINT('Ctrl Pts',(-34.5558333333333,-3.64215882054307,
1.9365701964918));
#28727=CARTESIAN_POINT('Ctrl Pts',(-34.529375,-4.76023814479221,-0.166231178980113));
#28728=CARTESIAN_POINT('Ctrl Pts',(-34.5029166666667,-3.49819839664525,
-2.18591696496196));
#28729=CARTESIAN_POINT('Ctrl Pts',(-34.4764583333333,-2.23615864849829,
-4.20560275094382));
#28730=CARTESIAN_POINT('Ctrl Pts',(-34.45,0.143960423897816,-4.12248716145376));
#28731=CARTESIAN_POINT('Ctrl Pts',(-34.4235416666667,2.52407949629392,-4.03937157196371));
#28732=CARTESIAN_POINT('Ctrl Pts',(-34.3970833333333,3.64215882054307,-1.9365701964918));
#28733=CARTESIAN_POINT('Ctrl Pts',(-34.370625,4.76023814479221,0.166231178980113));
#28734=CARTESIAN_POINT('Ctrl Pts',(-34.3441666666667,3.49819839664525,2.18591696496197));
#28735=CARTESIAN_POINT('Ctrl Pts',(-34.3177083333333,2.23615864849829,4.20560275094382));
#28736=CARTESIAN_POINT('Ctrl Pts',(-34.29125,-0.143960423897816,4.12248716145376));
#28737=CARTESIAN_POINT('Ctrl Pts',(-34.2647916666667,-2.52407949629392,
4.03937157196371));
#28738=CARTESIAN_POINT('Ctrl Pts',(-34.2383333333333,-3.64215882054307,
1.9365701964918));
#28739=CARTESIAN_POINT('Ctrl Pts',(-34.211875,-4.76023814479221,-0.166231178980113));
#28740=CARTESIAN_POINT('Ctrl Pts',(-34.1854166666667,-3.49819839664525,
-2.18591696496196));
#28741=CARTESIAN_POINT('Ctrl Pts',(-34.1589583333333,-2.23615864849829,
-4.20560275094382));
#28742=CARTESIAN_POINT('Ctrl Pts',(-34.1325,0.143960423897816,-4.12248716145376));
#28743=CARTESIAN_POINT('Ctrl Pts',(-34.1060416666667,2.52407949629392,-4.03937157196371));
#28744=CARTESIAN_POINT('Ctrl Pts',(-34.0795833333333,3.64215882054307,-1.9365701964918));
#28745=CARTESIAN_POINT('Ctrl Pts',(-34.053125,4.76023814479221,0.166231178980113));
#28746=CARTESIAN_POINT('Ctrl Pts',(-34.0266666666667,3.49819839664525,2.18591696496197));
#28747=CARTESIAN_POINT('Ctrl Pts',(-34.0009587714797,2.2719539027698,4.14831836955731));
#28748=CARTESIAN_POINT('Ctrl Pts',(-33.9748916174808,-0.0419478005003553,
4.12478670745932));
#28749=CARTESIAN_POINT('Ctrl Pts',(-43.8757812504336,0.149957969249583,
-4.29423438922274));
#28750=CARTESIAN_POINT('Ctrl Pts',(-43.8493229171003,2.62923534983068,-4.20765611530936));
#28751=CARTESIAN_POINT('Ctrl Pts',(-43.8228645837669,3.79389505549643,-2.0172497837413));
#28752=CARTESIAN_POINT('Ctrl Pts',(-43.7964062504336,4.95855476116219,0.173156547826753));
#28753=CARTESIAN_POINT('Ctrl Pts',(-43.7699479171003,3.64393708624685,2.27698460548143));
#28754=CARTESIAN_POINT('Ctrl Pts',(-43.7434895837669,2.32931941133151,4.38081266313611));
#28755=CARTESIAN_POINT('Ctrl Pts',(-43.7170312504336,-0.149957969249583,
4.29423438922274));
#28756=CARTESIAN_POINT('Ctrl Pts',(-43.6905729171003,-2.62923534983068,
4.20765611530936));
#28757=CARTESIAN_POINT('Ctrl Pts',(-43.6641145837669,-3.79389505549643,
2.01724978374131));
#28758=CARTESIAN_POINT('Ctrl Pts',(-43.6376562504336,-4.95855476116219,
-0.173156547826752));
#28759=CARTESIAN_POINT('Ctrl Pts',(-43.6111979171003,-3.64393708624685,
-2.27698460548143));
#28760=CARTESIAN_POINT('Ctrl Pts',(-43.5847395837669,-2.32931941133151,
-4.38081266313611));
#28761=CARTESIAN_POINT('Ctrl Pts',(-43.5582812504336,0.149957969249583,
-4.29423438922274));
#28762=CARTESIAN_POINT('Ctrl Pts',(-43.5318229171003,2.62923534983068,-4.20765611530936));
#28763=CARTESIAN_POINT('Ctrl Pts',(-43.5053645837669,3.79389505549643,-2.0172497837413));
#28764=CARTESIAN_POINT('Ctrl Pts',(-43.4789062504336,4.95855476116219,0.173156547826753));
#28765=CARTESIAN_POINT('Ctrl Pts',(-43.4524479171003,3.64393708624685,2.27698460548143));
#28766=CARTESIAN_POINT('Ctrl Pts',(-43.4259895837669,2.32931941133151,4.38081266313611));
#28767=CARTESIAN_POINT('Ctrl Pts',(-43.3995312504336,-0.149957969249583,
4.29423438922274));
#28768=CARTESIAN_POINT('Ctrl Pts',(-43.3730729171003,-2.62923534983068,
4.20765611530936));
#28769=CARTESIAN_POINT('Ctrl Pts',(-43.3466145837669,-3.79389505549643,
2.01724978374131));
#28770=CARTESIAN_POINT('Ctrl Pts',(-43.3201562504336,-4.95855476116219,
-0.173156547826752));
#28771=CARTESIAN_POINT('Ctrl Pts',(-43.2936979171003,-3.64393708624685,
-2.27698460548143));
#28772=CARTESIAN_POINT('Ctrl Pts',(-43.2672395837669,-2.32931941133151,
-4.38081266313611));
#28773=CARTESIAN_POINT('Ctrl Pts',(-43.2407812504336,0.149957969249583,
-4.29423438922274));
#28774=CARTESIAN_POINT('Ctrl Pts',(-43.2143229171003,2.62923534983068,-4.20765611530936));
#28775=CARTESIAN_POINT('Ctrl Pts',(-43.1878645837669,3.79389505549643,-2.0172497837413));
#28776=CARTESIAN_POINT('Ctrl Pts',(-43.1614062504336,4.95855476116219,0.173156547826753));
#28777=CARTESIAN_POINT('Ctrl Pts',(-43.1349479171003,3.64393708624685,2.27698460548143));
#28778=CARTESIAN_POINT('Ctrl Pts',(-43.1084895837669,2.32931941133151,4.38081266313611));
#28779=CARTESIAN_POINT('Ctrl Pts',(-43.0820312504336,-0.149957969249583,
4.29423438922274));
#28780=CARTESIAN_POINT('Ctrl Pts',(-43.0555729171003,-2.62923534983068,
4.20765611530936));
#28781=CARTESIAN_POINT('Ctrl Pts',(-43.0291145837669,-3.79389505549643,
2.01724978374131));
#28782=CARTESIAN_POINT('Ctrl Pts',(-43.0026562504336,-4.95855476116219,
-0.173156547826752));
#28783=CARTESIAN_POINT('Ctrl Pts',(-42.9761979171003,-3.64393708624685,
-2.27698460548143));
#28784=CARTESIAN_POINT('Ctrl Pts',(-42.9497395837669,-2.32931941133151,
-4.38081266313611));
#28785=CARTESIAN_POINT('Ctrl Pts',(-42.9232812504336,0.149957969249583,
-4.29423438922274));
#28786=CARTESIAN_POINT('Ctrl Pts',(-42.8968229171003,2.62923534983068,-4.20765611530936));
#28787=CARTESIAN_POINT('Ctrl Pts',(-42.8703645837669,3.79389505549643,-2.0172497837413));
#28788=CARTESIAN_POINT('Ctrl Pts',(-42.8439062504336,4.95855476116219,0.173156547826753));
#28789=CARTESIAN_POINT('Ctrl Pts',(-42.8174479171003,3.64393708624685,2.27698460548143));
#28790=CARTESIAN_POINT('Ctrl Pts',(-42.7909895837669,2.32931941133151,4.38081266313611));
#28791=CARTESIAN_POINT('Ctrl Pts',(-42.7645312504336,-0.149957969249583,
4.29423438922274));
#28792=CARTESIAN_POINT('Ctrl Pts',(-42.7380729171003,-2.62923534983068,
4.20765611530936));
#28793=CARTESIAN_POINT('Ctrl Pts',(-42.7116145837669,-3.79389505549643,
2.01724978374131));
#28794=CARTESIAN_POINT('Ctrl Pts',(-42.6851562504336,-4.95855476116219,
-0.173156547826752));
#28795=CARTESIAN_POINT('Ctrl Pts',(-42.6586979171003,-3.64393708624685,
-2.27698460548143));
#28796=CARTESIAN_POINT('Ctrl Pts',(-42.6322395837669,-2.32931941133151,
-4.38081266313611));
#28797=CARTESIAN_POINT('Ctrl Pts',(-42.6057812504336,0.149957969249583,
-4.29423438922274));
#28798=CARTESIAN_POINT('Ctrl Pts',(-42.5793229171003,2.62923534983068,-4.20765611530936));
#28799=CARTESIAN_POINT('Ctrl Pts',(-42.5528645837669,3.79389505549643,-2.0172497837413));
#28800=CARTESIAN_POINT('Ctrl Pts',(-42.5264062504336,4.95855476116219,0.173156547826753));
#28801=CARTESIAN_POINT('Ctrl Pts',(-42.4999479171003,3.64393708624685,2.27698460548143));
#28802=CARTESIAN_POINT('Ctrl Pts',(-42.4734895837669,2.32931941133151,4.38081266313611));
#28803=CARTESIAN_POINT('Ctrl Pts',(-42.4470312504336,-0.149957969249583,
4.29423438922274));
#28804=CARTESIAN_POINT('Ctrl Pts',(-42.4205729171003,-2.62923534983068,
4.20765611530936));
#28805=CARTESIAN_POINT('Ctrl Pts',(-42.3941145837669,-3.79389505549643,
2.01724978374131));
#28806=CARTESIAN_POINT('Ctrl Pts',(-42.3676562504336,-4.95855476116219,
-0.173156547826752));
#28807=CARTESIAN_POINT('Ctrl Pts',(-42.3411979171003,-3.64393708624685,
-2.27698460548143));
#28808=CARTESIAN_POINT('Ctrl Pts',(-42.3147395837669,-2.32931941133151,
-4.38081266313611));
#28809=CARTESIAN_POINT('Ctrl Pts',(-42.2882812504336,0.149957969249583,
-4.29423438922274));
#28810=CARTESIAN_POINT('Ctrl Pts',(-42.2618229171003,2.62923534983068,-4.20765611530936));
#28811=CARTESIAN_POINT('Ctrl Pts',(-42.2353645837669,3.79389505549643,-2.0172497837413));
#28812=CARTESIAN_POINT('Ctrl Pts',(-42.2089062504336,4.95855476116219,0.173156547826753));
#28813=CARTESIAN_POINT('Ctrl Pts',(-42.1824479171003,3.64393708624685,2.27698460548143));
#28814=CARTESIAN_POINT('Ctrl Pts',(-42.1559895837669,2.32931941133151,4.38081266313611));
#28815=CARTESIAN_POINT('Ctrl Pts',(-42.1295312504336,-0.149957969249583,
4.29423438922274));
#28816=CARTESIAN_POINT('Ctrl Pts',(-42.1030729171003,-2.62923534983068,
4.20765611530936));
#28817=CARTESIAN_POINT('Ctrl Pts',(-42.0766145837669,-3.79389505549643,
2.01724978374131));
#28818=CARTESIAN_POINT('Ctrl Pts',(-42.0501562504336,-4.95855476116219,
-0.173156547826752));
#28819=CARTESIAN_POINT('Ctrl Pts',(-42.0236979171003,-3.64393708624685,
-2.27698460548143));
#28820=CARTESIAN_POINT('Ctrl Pts',(-41.9972395837669,-2.32931941133151,
-4.38081266313611));
#28821=CARTESIAN_POINT('Ctrl Pts',(-41.9707812504336,0.149957969249583,
-4.29423438922274));
#28822=CARTESIAN_POINT('Ctrl Pts',(-41.9443229171003,2.62923534983068,-4.20765611530936));
#28823=CARTESIAN_POINT('Ctrl Pts',(-41.9178645837669,3.79389505549643,-2.0172497837413));
#28824=CARTESIAN_POINT('Ctrl Pts',(-41.8914062504336,4.95855476116219,0.173156547826753));
#28825=CARTESIAN_POINT('Ctrl Pts',(-41.8649479171003,3.64393708624685,2.27698460548143));
#28826=CARTESIAN_POINT('Ctrl Pts',(-41.8384895837669,2.32931941133151,4.38081266313611));
#28827=CARTESIAN_POINT('Ctrl Pts',(-41.8120312504336,-0.149957969249583,
4.29423438922274));
#28828=CARTESIAN_POINT('Ctrl Pts',(-41.7855729171003,-2.62923534983068,
4.20765611530936));
#28829=CARTESIAN_POINT('Ctrl Pts',(-41.7591145837669,-3.79389505549643,
2.01724978374131));
#28830=CARTESIAN_POINT('Ctrl Pts',(-41.7326562504336,-4.95855476116219,
-0.173156547826752));
#28831=CARTESIAN_POINT('Ctrl Pts',(-41.7061979171003,-3.64393708624685,
-2.27698460548143));
#28832=CARTESIAN_POINT('Ctrl Pts',(-41.6797395837669,-2.32931941133151,
-4.38081266313611));
#28833=CARTESIAN_POINT('Ctrl Pts',(-41.6532812504336,0.149957969249583,
-4.29423438922274));
#28834=CARTESIAN_POINT('Ctrl Pts',(-41.6268229171003,2.62923534983068,-4.20765611530936));
#28835=CARTESIAN_POINT('Ctrl Pts',(-41.6003645837669,3.79389505549643,-2.0172497837413));
#28836=CARTESIAN_POINT('Ctrl Pts',(-41.5739062504336,4.95855476116219,0.173156547826753));
#28837=CARTESIAN_POINT('Ctrl Pts',(-41.5474479171003,3.64393708624685,2.27698460548143));
#28838=CARTESIAN_POINT('Ctrl Pts',(-41.5209895837669,2.32931941133151,4.38081266313611));
#28839=CARTESIAN_POINT('Ctrl Pts',(-41.4945312504336,-0.149957969249583,
4.29423438922274));
#28840=CARTESIAN_POINT('Ctrl Pts',(-41.4680729171003,-2.62923534983068,
4.20765611530936));
#28841=CARTESIAN_POINT('Ctrl Pts',(-41.4416145837669,-3.79389505549643,
2.01724978374131));
#28842=CARTESIAN_POINT('Ctrl Pts',(-41.4151562504336,-4.95855476116219,
-0.173156547826752));
#28843=CARTESIAN_POINT('Ctrl Pts',(-41.3886979171003,-3.64393708624685,
-2.27698460548143));
#28844=CARTESIAN_POINT('Ctrl Pts',(-41.3622395837669,-2.32931941133151,
-4.38081266313611));
#28845=CARTESIAN_POINT('Ctrl Pts',(-41.3357812504336,0.149957969249583,
-4.29423438922274));
#28846=CARTESIAN_POINT('Ctrl Pts',(-41.3093229171003,2.62923534983068,-4.20765611530936));
#28847=CARTESIAN_POINT('Ctrl Pts',(-41.2828645837669,3.79389505549643,-2.0172497837413));
#28848=CARTESIAN_POINT('Ctrl Pts',(-41.2564062504336,4.95855476116219,0.173156547826753));
#28849=CARTESIAN_POINT('Ctrl Pts',(-41.2299479171003,3.64393708624685,2.27698460548143));
#28850=CARTESIAN_POINT('Ctrl Pts',(-41.2034895837669,2.32931941133151,4.38081266313611));
#28851=CARTESIAN_POINT('Ctrl Pts',(-41.1770312504336,-0.149957969249583,
4.29423438922274));
#28852=CARTESIAN_POINT('Ctrl Pts',(-41.1505729171003,-2.62923534983068,
4.20765611530936));
#28853=CARTESIAN_POINT('Ctrl Pts',(-41.1241145837669,-3.79389505549643,
2.01724978374131));
#28854=CARTESIAN_POINT('Ctrl Pts',(-41.0976562504336,-4.95855476116219,
-0.173156547826752));
#28855=CARTESIAN_POINT('Ctrl Pts',(-41.0711979171003,-3.64393708624685,
-2.27698460548143));
#28856=CARTESIAN_POINT('Ctrl Pts',(-41.0447395837669,-2.32931941133151,
-4.38081266313611));
#28857=CARTESIAN_POINT('Ctrl Pts',(-41.0182812504336,0.149957969249583,
-4.29423438922274));
#28858=CARTESIAN_POINT('Ctrl Pts',(-40.9918229171003,2.62923534983068,-4.20765611530936));
#28859=CARTESIAN_POINT('Ctrl Pts',(-40.9653645837669,3.79389505549643,-2.0172497837413));
#28860=CARTESIAN_POINT('Ctrl Pts',(-40.9389062504336,4.95855476116219,0.173156547826753));
#28861=CARTESIAN_POINT('Ctrl Pts',(-40.9124479171003,3.64393708624685,2.27698460548143));
#28862=CARTESIAN_POINT('Ctrl Pts',(-40.8859895837669,2.32931941133151,4.38081266313611));
#28863=CARTESIAN_POINT('Ctrl Pts',(-40.8595312504336,-0.149957969249583,
4.29423438922274));
#28864=CARTESIAN_POINT('Ctrl Pts',(-40.8330729171003,-2.62923534983068,
4.20765611530936));
#28865=CARTESIAN_POINT('Ctrl Pts',(-40.8066145837669,-3.79389505549643,
2.01724978374131));
#28866=CARTESIAN_POINT('Ctrl Pts',(-40.7801562504336,-4.95855476116219,
-0.173156547826752));
#28867=CARTESIAN_POINT('Ctrl Pts',(-40.7536979171003,-3.64393708624685,
-2.27698460548143));
#28868=CARTESIAN_POINT('Ctrl Pts',(-40.7272395837669,-2.32931941133151,
-4.38081266313611));
#28869=CARTESIAN_POINT('Ctrl Pts',(-40.7007812504336,0.149957969249583,
-4.29423438922274));
#28870=CARTESIAN_POINT('Ctrl Pts',(-40.6743229171003,2.62923534983068,-4.20765611530936));
#28871=CARTESIAN_POINT('Ctrl Pts',(-40.6478645837669,3.79389505549643,-2.0172497837413));
#28872=CARTESIAN_POINT('Ctrl Pts',(-40.6214062504336,4.95855476116219,0.173156547826753));
#28873=CARTESIAN_POINT('Ctrl Pts',(-40.5949479171003,3.64393708624685,2.27698460548143));
#28874=CARTESIAN_POINT('Ctrl Pts',(-40.5684895837669,2.32931941133151,4.38081266313611));
#28875=CARTESIAN_POINT('Ctrl Pts',(-40.5420312504336,-0.149957969249583,
4.29423438922274));
#28876=CARTESIAN_POINT('Ctrl Pts',(-40.5155729171003,-2.62923534983068,
4.20765611530936));
#28877=CARTESIAN_POINT('Ctrl Pts',(-40.4891145837669,-3.79389505549643,
2.01724978374131));
#28878=CARTESIAN_POINT('Ctrl Pts',(-40.4626562504336,-4.95855476116219,
-0.173156547826752));
#28879=CARTESIAN_POINT('Ctrl Pts',(-40.4361979171003,-3.64393708624685,
-2.27698460548143));
#28880=CARTESIAN_POINT('Ctrl Pts',(-40.4097395837669,-2.32931941133151,
-4.38081266313611));
#28881=CARTESIAN_POINT('Ctrl Pts',(-40.3832812504336,0.149957969249583,
-4.29423438922274));
#28882=CARTESIAN_POINT('Ctrl Pts',(-40.3568229171003,2.62923534983068,-4.20765611530936));
#28883=CARTESIAN_POINT('Ctrl Pts',(-40.3303645837669,3.79389505549643,-2.0172497837413));
#28884=CARTESIAN_POINT('Ctrl Pts',(-40.3039062504336,4.95855476116219,0.173156547826753));
#28885=CARTESIAN_POINT('Ctrl Pts',(-40.2774479171003,3.64393708624685,2.27698460548143));
#28886=CARTESIAN_POINT('Ctrl Pts',(-40.2509895837669,2.32931941133151,4.38081266313611));
#28887=CARTESIAN_POINT('Ctrl Pts',(-40.2245312504336,-0.149957969249583,
4.29423438922274));
#28888=CARTESIAN_POINT('Ctrl Pts',(-40.1980729171003,-2.62923534983068,
4.20765611530936));
#28889=CARTESIAN_POINT('Ctrl Pts',(-40.1716145837669,-3.79389505549643,
2.01724978374131));
#28890=CARTESIAN_POINT('Ctrl Pts',(-40.1451562504336,-4.95855476116219,
-0.173156547826752));
#28891=CARTESIAN_POINT('Ctrl Pts',(-40.1186979171003,-3.64393708624685,
-2.27698460548143));
#28892=CARTESIAN_POINT('Ctrl Pts',(-40.0922395837669,-2.32931941133151,
-4.38081266313611));
#28893=CARTESIAN_POINT('Ctrl Pts',(-40.0657812504336,0.149957969249583,
-4.29423438922274));
#28894=CARTESIAN_POINT('Ctrl Pts',(-40.0393229171003,2.62923534983068,-4.20765611530936));
#28895=CARTESIAN_POINT('Ctrl Pts',(-40.0128645837669,3.79389505549643,-2.0172497837413));
#28896=CARTESIAN_POINT('Ctrl Pts',(-39.9864062504336,4.95855476116219,0.173156547826753));
#28897=CARTESIAN_POINT('Ctrl Pts',(-39.9599479171003,3.64393708624685,2.27698460548143));
#28898=CARTESIAN_POINT('Ctrl Pts',(-39.9334895837669,2.32931941133151,4.38081266313611));
#28899=CARTESIAN_POINT('Ctrl Pts',(-39.9070312504336,-0.149957969249583,
4.29423438922274));
#28900=CARTESIAN_POINT('Ctrl Pts',(-39.8805729171003,-2.62923534983068,
4.20765611530936));
#28901=CARTESIAN_POINT('Ctrl Pts',(-39.8541145837669,-3.79389505549643,
2.01724978374131));
#28902=CARTESIAN_POINT('Ctrl Pts',(-39.8276562504336,-4.95855476116219,
-0.173156547826752));
#28903=CARTESIAN_POINT('Ctrl Pts',(-39.8011979171003,-3.64393708624685,
-2.27698460548143));
#28904=CARTESIAN_POINT('Ctrl Pts',(-39.7747395837669,-2.32931941133151,
-4.38081266313611));
#28905=CARTESIAN_POINT('Ctrl Pts',(-39.7482812504336,0.149957969249583,
-4.29423438922274));
#28906=CARTESIAN_POINT('Ctrl Pts',(-39.7218229171003,2.62923534983068,-4.20765611530936));
#28907=CARTESIAN_POINT('Ctrl Pts',(-39.6953645837669,3.79389505549643,-2.0172497837413));
#28908=CARTESIAN_POINT('Ctrl Pts',(-39.6689062504336,4.95855476116219,0.173156547826753));
#28909=CARTESIAN_POINT('Ctrl Pts',(-39.6424479171003,3.64393708624685,2.27698460548143));
#28910=CARTESIAN_POINT('Ctrl Pts',(-39.6159895837669,2.32931941133151,4.38081266313611));
#28911=CARTESIAN_POINT('Ctrl Pts',(-39.5895312504336,-0.149957969249583,
4.29423438922274));
#28912=CARTESIAN_POINT('Ctrl Pts',(-39.5630729171003,-2.62923534983068,
4.20765611530936));
#28913=CARTESIAN_POINT('Ctrl Pts',(-39.5366145837669,-3.79389505549643,
2.01724978374131));
#28914=CARTESIAN_POINT('Ctrl Pts',(-39.5101562504336,-4.95855476116219,
-0.173156547826752));
#28915=CARTESIAN_POINT('Ctrl Pts',(-39.4836979171003,-3.64393708624685,
-2.27698460548143));
#28916=CARTESIAN_POINT('Ctrl Pts',(-39.4572395837669,-2.32931941133151,
-4.38081266313611));
#28917=CARTESIAN_POINT('Ctrl Pts',(-39.4307812504336,0.149957969249583,
-4.29423438922274));
#28918=CARTESIAN_POINT('Ctrl Pts',(-39.4043229171003,2.62923534983068,-4.20765611530936));
#28919=CARTESIAN_POINT('Ctrl Pts',(-39.3778645837669,3.79389505549643,-2.0172497837413));
#28920=CARTESIAN_POINT('Ctrl Pts',(-39.3514062504336,4.95855476116219,0.173156547826753));
#28921=CARTESIAN_POINT('Ctrl Pts',(-39.3249479171003,3.64393708624685,2.27698460548143));
#28922=CARTESIAN_POINT('Ctrl Pts',(-39.2984895837669,2.32931941133151,4.38081266313611));
#28923=CARTESIAN_POINT('Ctrl Pts',(-39.2720312504336,-0.149957969249583,
4.29423438922274));
#28924=CARTESIAN_POINT('Ctrl Pts',(-39.2455729171003,-2.62923534983068,
4.20765611530936));
#28925=CARTESIAN_POINT('Ctrl Pts',(-39.2191145837669,-3.79389505549643,
2.01724978374131));
#28926=CARTESIAN_POINT('Ctrl Pts',(-39.1926562504336,-4.95855476116219,
-0.173156547826752));
#28927=CARTESIAN_POINT('Ctrl Pts',(-39.1661979171003,-3.64393708624685,
-2.27698460548143));
#28928=CARTESIAN_POINT('Ctrl Pts',(-39.1397395837669,-2.32931941133151,
-4.38081266313611));
#28929=CARTESIAN_POINT('Ctrl Pts',(-39.1132812504336,0.149957969249583,
-4.29423438922274));
#28930=CARTESIAN_POINT('Ctrl Pts',(-39.0868229171003,2.62923534983068,-4.20765611530936));
#28931=CARTESIAN_POINT('Ctrl Pts',(-39.0603645837669,3.79389505549643,-2.0172497837413));
#28932=CARTESIAN_POINT('Ctrl Pts',(-39.0339062504336,4.95855476116219,0.173156547826753));
#28933=CARTESIAN_POINT('Ctrl Pts',(-39.0074479171003,3.64393708624685,2.27698460548143));
#28934=CARTESIAN_POINT('Ctrl Pts',(-38.9809895837669,2.32931941133151,4.38081266313611));
#28935=CARTESIAN_POINT('Ctrl Pts',(-38.9545312504336,-0.149957969249583,
4.29423438922274));
#28936=CARTESIAN_POINT('Ctrl Pts',(-38.9280729171003,-2.62923534983068,
4.20765611530936));
#28937=CARTESIAN_POINT('Ctrl Pts',(-38.9016145837669,-3.79389505549643,
2.01724978374131));
#28938=CARTESIAN_POINT('Ctrl Pts',(-38.8751562504336,-4.95855476116219,
-0.173156547826752));
#28939=CARTESIAN_POINT('Ctrl Pts',(-38.8486979171003,-3.64393708624685,
-2.27698460548143));
#28940=CARTESIAN_POINT('Ctrl Pts',(-38.8222395837669,-2.32931941133151,
-4.38081266313611));
#28941=CARTESIAN_POINT('Ctrl Pts',(-38.7957812504336,0.149957969249583,
-4.29423438922274));
#28942=CARTESIAN_POINT('Ctrl Pts',(-38.7693229171003,2.62923534983068,-4.20765611530936));
#28943=CARTESIAN_POINT('Ctrl Pts',(-38.7428645837669,3.79389505549643,-2.0172497837413));
#28944=CARTESIAN_POINT('Ctrl Pts',(-38.7164062504336,4.95855476116219,0.173156547826753));
#28945=CARTESIAN_POINT('Ctrl Pts',(-38.6899479171003,3.64393708624685,2.27698460548143));
#28946=CARTESIAN_POINT('Ctrl Pts',(-38.6634895837669,2.32931941133151,4.38081266313611));
#28947=CARTESIAN_POINT('Ctrl Pts',(-38.6370312504336,-0.149957969249583,
4.29423438922274));
#28948=CARTESIAN_POINT('Ctrl Pts',(-38.6105729171003,-2.62923534983068,
4.20765611530936));
#28949=CARTESIAN_POINT('Ctrl Pts',(-38.5841145837669,-3.79389505549643,
2.01724978374131));
#28950=CARTESIAN_POINT('Ctrl Pts',(-38.5576562504336,-4.95855476116219,
-0.173156547826752));
#28951=CARTESIAN_POINT('Ctrl Pts',(-38.5311979171003,-3.64393708624685,
-2.27698460548143));
#28952=CARTESIAN_POINT('Ctrl Pts',(-38.5047395837669,-2.32931941133151,
-4.38081266313611));
#28953=CARTESIAN_POINT('Ctrl Pts',(-38.4782812504336,0.149957969249583,
-4.29423438922274));
#28954=CARTESIAN_POINT('Ctrl Pts',(-38.4518229171003,2.62923534983068,-4.20765611530936));
#28955=CARTESIAN_POINT('Ctrl Pts',(-38.4253645837669,3.79389505549643,-2.0172497837413));
#28956=CARTESIAN_POINT('Ctrl Pts',(-38.3989062504336,4.95855476116219,0.173156547826753));
#28957=CARTESIAN_POINT('Ctrl Pts',(-38.3724479171003,3.64393708624685,2.27698460548143));
#28958=CARTESIAN_POINT('Ctrl Pts',(-38.3459895837669,2.32931941133151,4.38081266313611));
#28959=CARTESIAN_POINT('Ctrl Pts',(-38.3195312504336,-0.149957969249583,
4.29423438922274));
#28960=CARTESIAN_POINT('Ctrl Pts',(-38.2930729171003,-2.62923534983068,
4.20765611530936));
#28961=CARTESIAN_POINT('Ctrl Pts',(-38.2666145837669,-3.79389505549643,
2.01724978374131));
#28962=CARTESIAN_POINT('Ctrl Pts',(-38.2401562504336,-4.95855476116219,
-0.173156547826752));
#28963=CARTESIAN_POINT('Ctrl Pts',(-38.2136979171003,-3.64393708624685,
-2.27698460548143));
#28964=CARTESIAN_POINT('Ctrl Pts',(-38.1872395837669,-2.32931941133151,
-4.38081266313611));
#28965=CARTESIAN_POINT('Ctrl Pts',(-38.1607812504336,0.149957969249583,
-4.29423438922274));
#28966=CARTESIAN_POINT('Ctrl Pts',(-38.1343229171003,2.62923534983068,-4.20765611530936));
#28967=CARTESIAN_POINT('Ctrl Pts',(-38.1078645837669,3.79389505549643,-2.0172497837413));
#28968=CARTESIAN_POINT('Ctrl Pts',(-38.0814062504336,4.95855476116219,0.173156547826753));
#28969=CARTESIAN_POINT('Ctrl Pts',(-38.0549479171003,3.64393708624685,2.27698460548143));
#28970=CARTESIAN_POINT('Ctrl Pts',(-38.0284895837669,2.32931941133151,4.38081266313611));
#28971=CARTESIAN_POINT('Ctrl Pts',(-38.0020312504336,-0.149957969249583,
4.29423438922274));
#28972=CARTESIAN_POINT('Ctrl Pts',(-37.9755729171003,-2.62923534983068,
4.20765611530936));
#28973=CARTESIAN_POINT('Ctrl Pts',(-37.9491145837669,-3.79389505549643,
2.01724978374131));
#28974=CARTESIAN_POINT('Ctrl Pts',(-37.9226562504336,-4.95855476116219,
-0.173156547826752));
#28975=CARTESIAN_POINT('Ctrl Pts',(-37.8961979171003,-3.64393708624685,
-2.27698460548143));
#28976=CARTESIAN_POINT('Ctrl Pts',(-37.8697395837669,-2.32931941133151,
-4.38081266313611));
#28977=CARTESIAN_POINT('Ctrl Pts',(-37.8432812504336,0.149957969249583,
-4.29423438922274));
#28978=CARTESIAN_POINT('Ctrl Pts',(-37.8168229171003,2.62923534983068,-4.20765611530936));
#28979=CARTESIAN_POINT('Ctrl Pts',(-37.7903645837669,3.79389505549643,-2.0172497837413));
#28980=CARTESIAN_POINT('Ctrl Pts',(-37.7639062504336,4.95855476116219,0.173156547826753));
#28981=CARTESIAN_POINT('Ctrl Pts',(-37.7374479171003,3.64393708624685,2.27698460548143));
#28982=CARTESIAN_POINT('Ctrl Pts',(-37.7109895837669,2.32931941133151,4.38081266313611));
#28983=CARTESIAN_POINT('Ctrl Pts',(-37.6845312504336,-0.149957969249583,
4.29423438922274));
#28984=CARTESIAN_POINT('Ctrl Pts',(-37.6580729171003,-2.62923534983068,
4.20765611530936));
#28985=CARTESIAN_POINT('Ctrl Pts',(-37.6316145837669,-3.79389505549643,
2.01724978374131));
#28986=CARTESIAN_POINT('Ctrl Pts',(-37.6051562504336,-4.95855476116219,
-0.173156547826752));
#28987=CARTESIAN_POINT('Ctrl Pts',(-37.5786979171003,-3.64393708624685,
-2.27698460548143));
#28988=CARTESIAN_POINT('Ctrl Pts',(-37.5522395837669,-2.32931941133151,
-4.38081266313611));
#28989=CARTESIAN_POINT('Ctrl Pts',(-37.5257812504336,0.149957969249583,
-4.29423438922274));
#28990=CARTESIAN_POINT('Ctrl Pts',(-37.4993229171003,2.62923534983068,-4.20765611530936));
#28991=CARTESIAN_POINT('Ctrl Pts',(-37.4728645837669,3.79389505549643,-2.0172497837413));
#28992=CARTESIAN_POINT('Ctrl Pts',(-37.4464062504336,4.95855476116219,0.173156547826753));
#28993=CARTESIAN_POINT('Ctrl Pts',(-37.4199479171003,3.64393708624685,2.27698460548143));
#28994=CARTESIAN_POINT('Ctrl Pts',(-37.3934895837669,2.32931941133151,4.38081266313611));
#28995=CARTESIAN_POINT('Ctrl Pts',(-37.3670312504336,-0.149957969249583,
4.29423438922274));
#28996=CARTESIAN_POINT('Ctrl Pts',(-37.3405729171003,-2.62923534983068,
4.20765611530936));
#28997=CARTESIAN_POINT('Ctrl Pts',(-37.3141145837669,-3.79389505549643,
2.01724978374131));
#28998=CARTESIAN_POINT('Ctrl Pts',(-37.2876562504336,-4.95855476116219,
-0.173156547826752));
#28999=CARTESIAN_POINT('Ctrl Pts',(-37.2611979171003,-3.64393708624685,
-2.27698460548143));
#29000=CARTESIAN_POINT('Ctrl Pts',(-37.2347395837669,-2.32931941133151,
-4.38081266313611));
#29001=CARTESIAN_POINT('Ctrl Pts',(-37.2082812504336,0.149957969249583,
-4.29423438922274));
#29002=CARTESIAN_POINT('Ctrl Pts',(-37.1818229171003,2.62923534983068,-4.20765611530936));
#29003=CARTESIAN_POINT('Ctrl Pts',(-37.1553645837669,3.79389505549643,-2.0172497837413));
#29004=CARTESIAN_POINT('Ctrl Pts',(-37.1289062504336,4.95855476116219,0.173156547826753));
#29005=CARTESIAN_POINT('Ctrl Pts',(-37.1024479171003,3.64393708624685,2.27698460548143));
#29006=CARTESIAN_POINT('Ctrl Pts',(-37.0759895837669,2.32931941133151,4.38081266313611));
#29007=CARTESIAN_POINT('Ctrl Pts',(-37.0495312504336,-0.149957969249583,
4.29423438922274));
#29008=CARTESIAN_POINT('Ctrl Pts',(-37.0230729171003,-2.62923534983068,
4.20765611530936));
#29009=CARTESIAN_POINT('Ctrl Pts',(-36.9966145837669,-3.79389505549643,
2.01724978374131));
#29010=CARTESIAN_POINT('Ctrl Pts',(-36.9701562504336,-4.95855476116219,
-0.173156547826752));
#29011=CARTESIAN_POINT('Ctrl Pts',(-36.9436979171003,-3.64393708624685,
-2.27698460548143));
#29012=CARTESIAN_POINT('Ctrl Pts',(-36.9172395837669,-2.32931941133151,
-4.38081266313611));
#29013=CARTESIAN_POINT('Ctrl Pts',(-36.8907812504336,0.149957969249583,
-4.29423438922274));
#29014=CARTESIAN_POINT('Ctrl Pts',(-36.8643229171003,2.62923534983068,-4.20765611530936));
#29015=CARTESIAN_POINT('Ctrl Pts',(-36.8378645837669,3.79389505549643,-2.0172497837413));
#29016=CARTESIAN_POINT('Ctrl Pts',(-36.8114062504336,4.95855476116219,0.173156547826753));
#29017=CARTESIAN_POINT('Ctrl Pts',(-36.7849479171003,3.64393708624685,2.27698460548143));
#29018=CARTESIAN_POINT('Ctrl Pts',(-36.7584895837669,2.32931941133151,4.38081266313611));
#29019=CARTESIAN_POINT('Ctrl Pts',(-36.7320312504336,-0.149957969249583,
4.29423438922274));
#29020=CARTESIAN_POINT('Ctrl Pts',(-36.7055729171003,-2.62923534983068,
4.20765611530936));
#29021=CARTESIAN_POINT('Ctrl Pts',(-36.6791145837669,-3.79389505549643,
2.01724978374131));
#29022=CARTESIAN_POINT('Ctrl Pts',(-36.6526562504336,-4.95855476116219,
-0.173156547826752));
#29023=CARTESIAN_POINT('Ctrl Pts',(-36.6261979171003,-3.64393708624685,
-2.27698460548143));
#29024=CARTESIAN_POINT('Ctrl Pts',(-36.5997395837669,-2.32931941133151,
-4.38081266313611));
#29025=CARTESIAN_POINT('Ctrl Pts',(-36.5732812504336,0.149957969249583,
-4.29423438922274));
#29026=CARTESIAN_POINT('Ctrl Pts',(-36.5468229171003,2.62923534983068,-4.20765611530936));
#29027=CARTESIAN_POINT('Ctrl Pts',(-36.5203645837669,3.79389505549643,-2.0172497837413));
#29028=CARTESIAN_POINT('Ctrl Pts',(-36.4939062504336,4.95855476116219,0.173156547826753));
#29029=CARTESIAN_POINT('Ctrl Pts',(-36.4674479171003,3.64393708624685,2.27698460548143));
#29030=CARTESIAN_POINT('Ctrl Pts',(-36.4409895837669,2.32931941133151,4.38081266313611));
#29031=CARTESIAN_POINT('Ctrl Pts',(-36.4145312504336,-0.149957969249583,
4.29423438922274));
#29032=CARTESIAN_POINT('Ctrl Pts',(-36.3880729171003,-2.62923534983068,
4.20765611530936));
#29033=CARTESIAN_POINT('Ctrl Pts',(-36.3616145837669,-3.79389505549643,
2.01724978374131));
#29034=CARTESIAN_POINT('Ctrl Pts',(-36.3351562504336,-4.95855476116219,
-0.173156547826752));
#29035=CARTESIAN_POINT('Ctrl Pts',(-36.3086979171003,-3.64393708624685,
-2.27698460548143));
#29036=CARTESIAN_POINT('Ctrl Pts',(-36.2822395837669,-2.32931941133151,
-4.38081266313611));
#29037=CARTESIAN_POINT('Ctrl Pts',(-36.2557812504336,0.149957969249583,
-4.29423438922274));
#29038=CARTESIAN_POINT('Ctrl Pts',(-36.2293229171003,2.62923534983068,-4.20765611530936));
#29039=CARTESIAN_POINT('Ctrl Pts',(-36.2028645837669,3.79389505549643,-2.0172497837413));
#29040=CARTESIAN_POINT('Ctrl Pts',(-36.1764062504336,4.95855476116219,0.173156547826753));
#29041=CARTESIAN_POINT('Ctrl Pts',(-36.1499479171003,3.64393708624685,2.27698460548143));
#29042=CARTESIAN_POINT('Ctrl Pts',(-36.1234895837669,2.32931941133151,4.38081266313611));
#29043=CARTESIAN_POINT('Ctrl Pts',(-36.0970312504336,-0.149957969249583,
4.29423438922274));
#29044=CARTESIAN_POINT('Ctrl Pts',(-36.0705729171003,-2.62923534983068,
4.20765611530936));
#29045=CARTESIAN_POINT('Ctrl Pts',(-36.0441145837669,-3.79389505549643,
2.01724978374131));
#29046=CARTESIAN_POINT('Ctrl Pts',(-36.0176562504336,-4.95855476116219,
-0.173156547826752));
#29047=CARTESIAN_POINT('Ctrl Pts',(-35.9911979171003,-3.64393708624685,
-2.27698460548143));
#29048=CARTESIAN_POINT('Ctrl Pts',(-35.9647395837669,-2.32931941133151,
-4.38081266313611));
#29049=CARTESIAN_POINT('Ctrl Pts',(-35.9382812504336,0.149957969249583,
-4.29423438922274));
#29050=CARTESIAN_POINT('Ctrl Pts',(-35.9118229171003,2.62923534983068,-4.20765611530936));
#29051=CARTESIAN_POINT('Ctrl Pts',(-35.8853645837669,3.79389505549643,-2.0172497837413));
#29052=CARTESIAN_POINT('Ctrl Pts',(-35.8589062504336,4.95855476116219,0.173156547826753));
#29053=CARTESIAN_POINT('Ctrl Pts',(-35.8324479171003,3.64393708624685,2.27698460548143));
#29054=CARTESIAN_POINT('Ctrl Pts',(-35.8059895837669,2.32931941133151,4.38081266313611));
#29055=CARTESIAN_POINT('Ctrl Pts',(-35.7795312504336,-0.149957969249583,
4.29423438922274));
#29056=CARTESIAN_POINT('Ctrl Pts',(-35.7530729171003,-2.62923534983068,
4.20765611530936));
#29057=CARTESIAN_POINT('Ctrl Pts',(-35.7266145837669,-3.79389505549643,
2.01724978374131));
#29058=CARTESIAN_POINT('Ctrl Pts',(-35.7001562504336,-4.95855476116219,
-0.173156547826752));
#29059=CARTESIAN_POINT('Ctrl Pts',(-35.6736979171003,-3.64393708624685,
-2.27698460548143));
#29060=CARTESIAN_POINT('Ctrl Pts',(-35.6472395837669,-2.32931941133151,
-4.38081266313611));
#29061=CARTESIAN_POINT('Ctrl Pts',(-35.6207812504336,0.149957969249583,
-4.29423438922274));
#29062=CARTESIAN_POINT('Ctrl Pts',(-35.5943229171003,2.62923534983068,-4.20765611530936));
#29063=CARTESIAN_POINT('Ctrl Pts',(-35.5678645837669,3.79389505549643,-2.0172497837413));
#29064=CARTESIAN_POINT('Ctrl Pts',(-35.5414062504336,4.95855476116219,0.173156547826753));
#29065=CARTESIAN_POINT('Ctrl Pts',(-35.5149479171003,3.64393708624685,2.27698460548143));
#29066=CARTESIAN_POINT('Ctrl Pts',(-35.4884895837669,2.32931941133151,4.38081266313611));
#29067=CARTESIAN_POINT('Ctrl Pts',(-35.4620312504336,-0.149957969249583,
4.29423438922274));
#29068=CARTESIAN_POINT('Ctrl Pts',(-35.4355729171003,-2.62923534983068,
4.20765611530936));
#29069=CARTESIAN_POINT('Ctrl Pts',(-35.4091145837669,-3.79389505549643,
2.01724978374131));
#29070=CARTESIAN_POINT('Ctrl Pts',(-35.3826562504336,-4.95855476116219,
-0.173156547826752));
#29071=CARTESIAN_POINT('Ctrl Pts',(-35.3561979171003,-3.64393708624685,
-2.27698460548143));
#29072=CARTESIAN_POINT('Ctrl Pts',(-35.3297395837669,-2.32931941133151,
-4.38081266313611));
#29073=CARTESIAN_POINT('Ctrl Pts',(-35.3032812504336,0.149957969249583,
-4.29423438922274));
#29074=CARTESIAN_POINT('Ctrl Pts',(-35.2768229171003,2.62923534983068,-4.20765611530936));
#29075=CARTESIAN_POINT('Ctrl Pts',(-35.2503645837669,3.79389505549643,-2.0172497837413));
#29076=CARTESIAN_POINT('Ctrl Pts',(-35.2239062504336,4.95855476116219,0.173156547826753));
#29077=CARTESIAN_POINT('Ctrl Pts',(-35.1974479171003,3.64393708624685,2.27698460548143));
#29078=CARTESIAN_POINT('Ctrl Pts',(-35.1709895837669,2.32931941133151,4.38081266313611));
#29079=CARTESIAN_POINT('Ctrl Pts',(-35.1445312504336,-0.149957969249583,
4.29423438922274));
#29080=CARTESIAN_POINT('Ctrl Pts',(-35.1180729171003,-2.62923534983068,
4.20765611530936));
#29081=CARTESIAN_POINT('Ctrl Pts',(-35.0916145837669,-3.79389505549643,
2.01724978374131));
#29082=CARTESIAN_POINT('Ctrl Pts',(-35.0651562504336,-4.95855476116219,
-0.173156547826752));
#29083=CARTESIAN_POINT('Ctrl Pts',(-35.0386979171003,-3.64393708624685,
-2.27698460548143));
#29084=CARTESIAN_POINT('Ctrl Pts',(-35.0122395837669,-2.32931941133151,
-4.38081266313611));
#29085=CARTESIAN_POINT('Ctrl Pts',(-34.9857812504336,0.149957969249583,
-4.29423438922274));
#29086=CARTESIAN_POINT('Ctrl Pts',(-34.9593229171003,2.62923534983068,-4.20765611530936));
#29087=CARTESIAN_POINT('Ctrl Pts',(-34.9328645837669,3.79389505549643,-2.0172497837413));
#29088=CARTESIAN_POINT('Ctrl Pts',(-34.9064062504336,4.95855476116219,0.173156547826753));
#29089=CARTESIAN_POINT('Ctrl Pts',(-34.8799479171003,3.64393708624685,2.27698460548143));
#29090=CARTESIAN_POINT('Ctrl Pts',(-34.8534895837669,2.32931941133151,4.38081266313611));
#29091=CARTESIAN_POINT('Ctrl Pts',(-34.8270312504336,-0.149957969249583,
4.29423438922274));
#29092=CARTESIAN_POINT('Ctrl Pts',(-34.8005729171003,-2.62923534983068,
4.20765611530936));
#29093=CARTESIAN_POINT('Ctrl Pts',(-34.7741145837669,-3.79389505549643,
2.01724978374131));
#29094=CARTESIAN_POINT('Ctrl Pts',(-34.7476562504336,-4.95855476116219,
-0.173156547826752));
#29095=CARTESIAN_POINT('Ctrl Pts',(-34.7211979171003,-3.64393708624685,
-2.27698460548143));
#29096=CARTESIAN_POINT('Ctrl Pts',(-34.6947395837669,-2.32931941133151,
-4.38081266313611));
#29097=CARTESIAN_POINT('Ctrl Pts',(-34.6682812504336,0.149957969249583,
-4.29423438922274));
#29098=CARTESIAN_POINT('Ctrl Pts',(-34.6418229171003,2.62923534983068,-4.20765611530936));
#29099=CARTESIAN_POINT('Ctrl Pts',(-34.6153645837669,3.79389505549643,-2.0172497837413));
#29100=CARTESIAN_POINT('Ctrl Pts',(-34.5889062504336,4.95855476116219,0.173156547826753));
#29101=CARTESIAN_POINT('Ctrl Pts',(-34.5624479171003,3.64393708624685,2.27698460548143));
#29102=CARTESIAN_POINT('Ctrl Pts',(-34.5359895837669,2.32931941133151,4.38081266313611));
#29103=CARTESIAN_POINT('Ctrl Pts',(-34.5095312504336,-0.149957969249583,
4.29423438922274));
#29104=CARTESIAN_POINT('Ctrl Pts',(-34.4830729171003,-2.62923534983068,
4.20765611530936));
#29105=CARTESIAN_POINT('Ctrl Pts',(-34.4566145837669,-3.79389505549643,
2.01724978374131));
#29106=CARTESIAN_POINT('Ctrl Pts',(-34.4301562504336,-4.95855476116219,
-0.173156547826752));
#29107=CARTESIAN_POINT('Ctrl Pts',(-34.4036979171003,-3.64393708624685,
-2.27698460548143));
#29108=CARTESIAN_POINT('Ctrl Pts',(-34.3772395837669,-2.32931941133151,
-4.38081266313611));
#29109=CARTESIAN_POINT('Ctrl Pts',(-34.3507812504336,0.149957969249583,
-4.29423438922274));
#29110=CARTESIAN_POINT('Ctrl Pts',(-34.3243229171003,2.62923534983068,-4.20765611530936));
#29111=CARTESIAN_POINT('Ctrl Pts',(-34.2978645837669,3.79389505549643,-2.0172497837413));
#29112=CARTESIAN_POINT('Ctrl Pts',(-34.2714062504336,4.95855476116219,0.173156547826753));
#29113=CARTESIAN_POINT('Ctrl Pts',(-34.2449479171003,3.64393708624685,2.27698460548143));
#29114=CARTESIAN_POINT('Ctrl Pts',(-34.2184895837669,2.32931941133151,4.38081266313611));
#29115=CARTESIAN_POINT('Ctrl Pts',(-34.1920312504336,-0.149957969249583,
4.29423438922274));
#29116=CARTESIAN_POINT('Ctrl Pts',(-34.1655729171003,-2.62923534983068,
4.20765611530936));
#29117=CARTESIAN_POINT('Ctrl Pts',(-34.1391145837669,-3.79389505549643,
2.01724978374131));
#29118=CARTESIAN_POINT('Ctrl Pts',(-34.1126562504336,-4.95855476116219,
-0.173156547826752));
#29119=CARTESIAN_POINT('Ctrl Pts',(-34.0861979171003,-3.64393708624685,
-2.27698460548143));
#29120=CARTESIAN_POINT('Ctrl Pts',(-34.0597395837669,-2.32931941133151,
-4.38081266313611));
#29121=CARTESIAN_POINT('Ctrl Pts',(-34.0332812504336,0.149957969249583,
-4.29423438922274));
#29122=CARTESIAN_POINT('Ctrl Pts',(-34.0068229171003,2.62923534983068,-4.20765611530936));
#29123=CARTESIAN_POINT('Ctrl Pts',(-33.9803645837669,3.79389505549643,-2.0172497837413));
#29124=CARTESIAN_POINT('Ctrl Pts',(-33.9539062504336,4.95855476116219,0.173156547826753));
#29125=CARTESIAN_POINT('Ctrl Pts',(-33.9274479171003,3.64393708624685,2.27698460548143));
#29126=CARTESIAN_POINT('Ctrl Pts',(-33.9017400219133,2.36660593421046,4.32114175310506));
#29127=CARTESIAN_POINT('Ctrl Pts',(-33.8756728679143,-0.043695390769236,
4.29662973677627));
#29128=CARTESIAN_POINT('Ctrl Pts',(-43.8360937504336,0.149957969249583,
-4.29423438922274));
#29129=CARTESIAN_POINT('Ctrl Pts',(-43.8096354171003,2.62923534983068,-4.20765611530936));
#29130=CARTESIAN_POINT('Ctrl Pts',(-43.7831770837669,3.79389505549644,-2.0172497837413));
#29131=CARTESIAN_POINT('Ctrl Pts',(-43.7567187504336,4.95855476116219,0.173156547826753));
#29132=CARTESIAN_POINT('Ctrl Pts',(-43.7302604171003,3.64393708624685,2.27698460548143));
#29133=CARTESIAN_POINT('Ctrl Pts',(-43.7038020837669,2.32931941133151,4.38081266313611));
#29134=CARTESIAN_POINT('Ctrl Pts',(-43.6773437504336,-0.149957969249583,
4.29423438922274));
#29135=CARTESIAN_POINT('Ctrl Pts',(-43.6508854171003,-2.62923534983068,
4.20765611530936));
#29136=CARTESIAN_POINT('Ctrl Pts',(-43.6244270837669,-3.79389505549643,
2.01724978374131));
#29137=CARTESIAN_POINT('Ctrl Pts',(-43.5979687504336,-4.95855476116219,
-0.173156547826752));
#29138=CARTESIAN_POINT('Ctrl Pts',(-43.5715104171003,-3.64393708624685,
-2.27698460548143));
#29139=CARTESIAN_POINT('Ctrl Pts',(-43.5450520837669,-2.32931941133151,
-4.38081266313611));
#29140=CARTESIAN_POINT('Ctrl Pts',(-43.5185937504336,0.149957969249583,
-4.29423438922274));
#29141=CARTESIAN_POINT('Ctrl Pts',(-43.4921354171003,2.62923534983068,-4.20765611530936));
#29142=CARTESIAN_POINT('Ctrl Pts',(-43.4656770837669,3.79389505549644,-2.0172497837413));
#29143=CARTESIAN_POINT('Ctrl Pts',(-43.4392187504336,4.95855476116219,0.173156547826753));
#29144=CARTESIAN_POINT('Ctrl Pts',(-43.4127604171003,3.64393708624685,2.27698460548143));
#29145=CARTESIAN_POINT('Ctrl Pts',(-43.3863020837669,2.32931941133151,4.38081266313611));
#29146=CARTESIAN_POINT('Ctrl Pts',(-43.3598437504336,-0.149957969249583,
4.29423438922274));
#29147=CARTESIAN_POINT('Ctrl Pts',(-43.3333854171003,-2.62923534983068,
4.20765611530936));
#29148=CARTESIAN_POINT('Ctrl Pts',(-43.3069270837669,-3.79389505549643,
2.01724978374131));
#29149=CARTESIAN_POINT('Ctrl Pts',(-43.2804687504336,-4.95855476116219,
-0.173156547826752));
#29150=CARTESIAN_POINT('Ctrl Pts',(-43.2540104171003,-3.64393708624685,
-2.27698460548143));
#29151=CARTESIAN_POINT('Ctrl Pts',(-43.2275520837669,-2.32931941133151,
-4.38081266313611));
#29152=CARTESIAN_POINT('Ctrl Pts',(-43.2010937504336,0.149957969249583,
-4.29423438922274));
#29153=CARTESIAN_POINT('Ctrl Pts',(-43.1746354171003,2.62923534983068,-4.20765611530936));
#29154=CARTESIAN_POINT('Ctrl Pts',(-43.1481770837669,3.79389505549644,-2.0172497837413));
#29155=CARTESIAN_POINT('Ctrl Pts',(-43.1217187504336,4.95855476116219,0.173156547826753));
#29156=CARTESIAN_POINT('Ctrl Pts',(-43.0952604171003,3.64393708624685,2.27698460548143));
#29157=CARTESIAN_POINT('Ctrl Pts',(-43.0688020837669,2.32931941133151,4.38081266313611));
#29158=CARTESIAN_POINT('Ctrl Pts',(-43.0423437504336,-0.149957969249583,
4.29423438922274));
#29159=CARTESIAN_POINT('Ctrl Pts',(-43.0158854171003,-2.62923534983068,
4.20765611530936));
#29160=CARTESIAN_POINT('Ctrl Pts',(-42.9894270837669,-3.79389505549643,
2.01724978374131));
#29161=CARTESIAN_POINT('Ctrl Pts',(-42.9629687504336,-4.95855476116219,
-0.173156547826752));
#29162=CARTESIAN_POINT('Ctrl Pts',(-42.9365104171003,-3.64393708624685,
-2.27698460548143));
#29163=CARTESIAN_POINT('Ctrl Pts',(-42.9100520837669,-2.32931941133151,
-4.38081266313611));
#29164=CARTESIAN_POINT('Ctrl Pts',(-42.8835937504336,0.149957969249583,
-4.29423438922274));
#29165=CARTESIAN_POINT('Ctrl Pts',(-42.8571354171003,2.62923534983068,-4.20765611530936));
#29166=CARTESIAN_POINT('Ctrl Pts',(-42.8306770837669,3.79389505549644,-2.0172497837413));
#29167=CARTESIAN_POINT('Ctrl Pts',(-42.8042187504336,4.95855476116219,0.173156547826753));
#29168=CARTESIAN_POINT('Ctrl Pts',(-42.7777604171003,3.64393708624685,2.27698460548143));
#29169=CARTESIAN_POINT('Ctrl Pts',(-42.7513020837669,2.32931941133151,4.38081266313611));
#29170=CARTESIAN_POINT('Ctrl Pts',(-42.7248437504336,-0.149957969249583,
4.29423438922274));
#29171=CARTESIAN_POINT('Ctrl Pts',(-42.6983854171003,-2.62923534983068,
4.20765611530936));
#29172=CARTESIAN_POINT('Ctrl Pts',(-42.6719270837669,-3.79389505549643,
2.01724978374131));
#29173=CARTESIAN_POINT('Ctrl Pts',(-42.6454687504336,-4.95855476116219,
-0.173156547826752));
#29174=CARTESIAN_POINT('Ctrl Pts',(-42.6190104171003,-3.64393708624685,
-2.27698460548143));
#29175=CARTESIAN_POINT('Ctrl Pts',(-42.5925520837669,-2.32931941133151,
-4.38081266313611));
#29176=CARTESIAN_POINT('Ctrl Pts',(-42.5660937504336,0.149957969249583,
-4.29423438922274));
#29177=CARTESIAN_POINT('Ctrl Pts',(-42.5396354171003,2.62923534983068,-4.20765611530936));
#29178=CARTESIAN_POINT('Ctrl Pts',(-42.5131770837669,3.79389505549644,-2.0172497837413));
#29179=CARTESIAN_POINT('Ctrl Pts',(-42.4867187504336,4.95855476116219,0.173156547826753));
#29180=CARTESIAN_POINT('Ctrl Pts',(-42.4602604171003,3.64393708624685,2.27698460548143));
#29181=CARTESIAN_POINT('Ctrl Pts',(-42.4338020837669,2.32931941133151,4.38081266313611));
#29182=CARTESIAN_POINT('Ctrl Pts',(-42.4073437504336,-0.149957969249583,
4.29423438922274));
#29183=CARTESIAN_POINT('Ctrl Pts',(-42.3808854171003,-2.62923534983068,
4.20765611530936));
#29184=CARTESIAN_POINT('Ctrl Pts',(-42.3544270837669,-3.79389505549643,
2.01724978374131));
#29185=CARTESIAN_POINT('Ctrl Pts',(-42.3279687504336,-4.95855476116219,
-0.173156547826752));
#29186=CARTESIAN_POINT('Ctrl Pts',(-42.3015104171003,-3.64393708624685,
-2.27698460548143));
#29187=CARTESIAN_POINT('Ctrl Pts',(-42.2750520837669,-2.32931941133151,
-4.38081266313611));
#29188=CARTESIAN_POINT('Ctrl Pts',(-42.2485937504336,0.149957969249583,
-4.29423438922274));
#29189=CARTESIAN_POINT('Ctrl Pts',(-42.2221354171003,2.62923534983068,-4.20765611530936));
#29190=CARTESIAN_POINT('Ctrl Pts',(-42.1956770837669,3.79389505549644,-2.0172497837413));
#29191=CARTESIAN_POINT('Ctrl Pts',(-42.1692187504336,4.95855476116219,0.173156547826753));
#29192=CARTESIAN_POINT('Ctrl Pts',(-42.1427604171003,3.64393708624685,2.27698460548143));
#29193=CARTESIAN_POINT('Ctrl Pts',(-42.1163020837669,2.32931941133151,4.38081266313611));
#29194=CARTESIAN_POINT('Ctrl Pts',(-42.0898437504336,-0.149957969249583,
4.29423438922274));
#29195=CARTESIAN_POINT('Ctrl Pts',(-42.0633854171003,-2.62923534983068,
4.20765611530936));
#29196=CARTESIAN_POINT('Ctrl Pts',(-42.0369270837669,-3.79389505549643,
2.01724978374131));
#29197=CARTESIAN_POINT('Ctrl Pts',(-42.0104687504336,-4.95855476116219,
-0.173156547826752));
#29198=CARTESIAN_POINT('Ctrl Pts',(-41.9840104171003,-3.64393708624685,
-2.27698460548143));
#29199=CARTESIAN_POINT('Ctrl Pts',(-41.9575520837669,-2.32931941133151,
-4.38081266313611));
#29200=CARTESIAN_POINT('Ctrl Pts',(-41.9310937504336,0.149957969249583,
-4.29423438922274));
#29201=CARTESIAN_POINT('Ctrl Pts',(-41.9046354171003,2.62923534983068,-4.20765611530936));
#29202=CARTESIAN_POINT('Ctrl Pts',(-41.8781770837669,3.79389505549644,-2.0172497837413));
#29203=CARTESIAN_POINT('Ctrl Pts',(-41.8517187504336,4.95855476116219,0.173156547826753));
#29204=CARTESIAN_POINT('Ctrl Pts',(-41.8252604171003,3.64393708624685,2.27698460548143));
#29205=CARTESIAN_POINT('Ctrl Pts',(-41.7988020837669,2.32931941133151,4.38081266313611));
#29206=CARTESIAN_POINT('Ctrl Pts',(-41.7723437504336,-0.149957969249583,
4.29423438922274));
#29207=CARTESIAN_POINT('Ctrl Pts',(-41.7458854171003,-2.62923534983068,
4.20765611530936));
#29208=CARTESIAN_POINT('Ctrl Pts',(-41.7194270837669,-3.79389505549643,
2.01724978374131));
#29209=CARTESIAN_POINT('Ctrl Pts',(-41.6929687504336,-4.95855476116219,
-0.173156547826752));
#29210=CARTESIAN_POINT('Ctrl Pts',(-41.6665104171003,-3.64393708624685,
-2.27698460548143));
#29211=CARTESIAN_POINT('Ctrl Pts',(-41.6400520837669,-2.32931941133151,
-4.38081266313611));
#29212=CARTESIAN_POINT('Ctrl Pts',(-41.6135937504336,0.149957969249583,
-4.29423438922274));
#29213=CARTESIAN_POINT('Ctrl Pts',(-41.5871354171003,2.62923534983068,-4.20765611530936));
#29214=CARTESIAN_POINT('Ctrl Pts',(-41.5606770837669,3.79389505549644,-2.0172497837413));
#29215=CARTESIAN_POINT('Ctrl Pts',(-41.5342187504336,4.95855476116219,0.173156547826753));
#29216=CARTESIAN_POINT('Ctrl Pts',(-41.5077604171003,3.64393708624685,2.27698460548143));
#29217=CARTESIAN_POINT('Ctrl Pts',(-41.4813020837669,2.32931941133151,4.38081266313611));
#29218=CARTESIAN_POINT('Ctrl Pts',(-41.4548437504336,-0.149957969249583,
4.29423438922274));
#29219=CARTESIAN_POINT('Ctrl Pts',(-41.4283854171003,-2.62923534983068,
4.20765611530936));
#29220=CARTESIAN_POINT('Ctrl Pts',(-41.4019270837669,-3.79389505549643,
2.01724978374131));
#29221=CARTESIAN_POINT('Ctrl Pts',(-41.3754687504336,-4.95855476116219,
-0.173156547826752));
#29222=CARTESIAN_POINT('Ctrl Pts',(-41.3490104171003,-3.64393708624685,
-2.27698460548143));
#29223=CARTESIAN_POINT('Ctrl Pts',(-41.3225520837669,-2.32931941133151,
-4.38081266313611));
#29224=CARTESIAN_POINT('Ctrl Pts',(-41.2960937504336,0.149957969249583,
-4.29423438922274));
#29225=CARTESIAN_POINT('Ctrl Pts',(-41.2696354171003,2.62923534983068,-4.20765611530936));
#29226=CARTESIAN_POINT('Ctrl Pts',(-41.2431770837669,3.79389505549644,-2.0172497837413));
#29227=CARTESIAN_POINT('Ctrl Pts',(-41.2167187504336,4.95855476116219,0.173156547826753));
#29228=CARTESIAN_POINT('Ctrl Pts',(-41.1902604171003,3.64393708624685,2.27698460548143));
#29229=CARTESIAN_POINT('Ctrl Pts',(-41.1638020837669,2.32931941133151,4.38081266313611));
#29230=CARTESIAN_POINT('Ctrl Pts',(-41.1373437504336,-0.149957969249583,
4.29423438922274));
#29231=CARTESIAN_POINT('Ctrl Pts',(-41.1108854171003,-2.62923534983068,
4.20765611530936));
#29232=CARTESIAN_POINT('Ctrl Pts',(-41.0844270837669,-3.79389505549643,
2.01724978374131));
#29233=CARTESIAN_POINT('Ctrl Pts',(-41.0579687504336,-4.95855476116219,
-0.173156547826752));
#29234=CARTESIAN_POINT('Ctrl Pts',(-41.0315104171003,-3.64393708624685,
-2.27698460548143));
#29235=CARTESIAN_POINT('Ctrl Pts',(-41.0050520837669,-2.32931941133151,
-4.38081266313611));
#29236=CARTESIAN_POINT('Ctrl Pts',(-40.9785937504336,0.149957969249583,
-4.29423438922274));
#29237=CARTESIAN_POINT('Ctrl Pts',(-40.9521354171003,2.62923534983068,-4.20765611530936));
#29238=CARTESIAN_POINT('Ctrl Pts',(-40.9256770837669,3.79389505549644,-2.0172497837413));
#29239=CARTESIAN_POINT('Ctrl Pts',(-40.8992187504336,4.95855476116219,0.173156547826753));
#29240=CARTESIAN_POINT('Ctrl Pts',(-40.8727604171003,3.64393708624685,2.27698460548143));
#29241=CARTESIAN_POINT('Ctrl Pts',(-40.8463020837669,2.32931941133151,4.38081266313611));
#29242=CARTESIAN_POINT('Ctrl Pts',(-40.8198437504336,-0.149957969249583,
4.29423438922274));
#29243=CARTESIAN_POINT('Ctrl Pts',(-40.7933854171003,-2.62923534983068,
4.20765611530936));
#29244=CARTESIAN_POINT('Ctrl Pts',(-40.7669270837669,-3.79389505549643,
2.01724978374131));
#29245=CARTESIAN_POINT('Ctrl Pts',(-40.7404687504336,-4.95855476116219,
-0.173156547826752));
#29246=CARTESIAN_POINT('Ctrl Pts',(-40.7140104171003,-3.64393708624685,
-2.27698460548143));
#29247=CARTESIAN_POINT('Ctrl Pts',(-40.6875520837669,-2.32931941133151,
-4.38081266313611));
#29248=CARTESIAN_POINT('Ctrl Pts',(-40.6610937504336,0.149957969249583,
-4.29423438922274));
#29249=CARTESIAN_POINT('Ctrl Pts',(-40.6346354171003,2.62923534983068,-4.20765611530936));
#29250=CARTESIAN_POINT('Ctrl Pts',(-40.6081770837669,3.79389505549644,-2.0172497837413));
#29251=CARTESIAN_POINT('Ctrl Pts',(-40.5817187504336,4.95855476116219,0.173156547826753));
#29252=CARTESIAN_POINT('Ctrl Pts',(-40.5552604171002,3.64393708624685,2.27698460548143));
#29253=CARTESIAN_POINT('Ctrl Pts',(-40.5288020837669,2.32931941133151,4.38081266313611));
#29254=CARTESIAN_POINT('Ctrl Pts',(-40.5023437504336,-0.149957969249583,
4.29423438922274));
#29255=CARTESIAN_POINT('Ctrl Pts',(-40.4758854171003,-2.62923534983068,
4.20765611530936));
#29256=CARTESIAN_POINT('Ctrl Pts',(-40.4494270837669,-3.79389505549643,
2.01724978374131));
#29257=CARTESIAN_POINT('Ctrl Pts',(-40.4229687504336,-4.95855476116219,
-0.173156547826752));
#29258=CARTESIAN_POINT('Ctrl Pts',(-40.3965104171003,-3.64393708624685,
-2.27698460548143));
#29259=CARTESIAN_POINT('Ctrl Pts',(-40.3700520837669,-2.32931941133151,
-4.38081266313611));
#29260=CARTESIAN_POINT('Ctrl Pts',(-40.3435937504336,0.149957969249583,
-4.29423438922274));
#29261=CARTESIAN_POINT('Ctrl Pts',(-40.3171354171003,2.62923534983068,-4.20765611530936));
#29262=CARTESIAN_POINT('Ctrl Pts',(-40.2906770837669,3.79389505549644,-2.0172497837413));
#29263=CARTESIAN_POINT('Ctrl Pts',(-40.2642187504336,4.95855476116219,0.173156547826753));
#29264=CARTESIAN_POINT('Ctrl Pts',(-40.2377604171003,3.64393708624685,2.27698460548143));
#29265=CARTESIAN_POINT('Ctrl Pts',(-40.2113020837669,2.32931941133151,4.38081266313611));
#29266=CARTESIAN_POINT('Ctrl Pts',(-40.1848437504336,-0.149957969249583,
4.29423438922274));
#29267=CARTESIAN_POINT('Ctrl Pts',(-40.1583854171003,-2.62923534983068,
4.20765611530936));
#29268=CARTESIAN_POINT('Ctrl Pts',(-40.1319270837669,-3.79389505549643,
2.01724978374131));
#29269=CARTESIAN_POINT('Ctrl Pts',(-40.1054687504336,-4.95855476116219,
-0.173156547826752));
#29270=CARTESIAN_POINT('Ctrl Pts',(-40.0790104171003,-3.64393708624685,
-2.27698460548143));
#29271=CARTESIAN_POINT('Ctrl Pts',(-40.0525520837669,-2.32931941133151,
-4.38081266313611));
#29272=CARTESIAN_POINT('Ctrl Pts',(-40.0260937504336,0.149957969249583,
-4.29423438922274));
#29273=CARTESIAN_POINT('Ctrl Pts',(-39.9996354171003,2.62923534983068,-4.20765611530936));
#29274=CARTESIAN_POINT('Ctrl Pts',(-39.9731770837669,3.79389505549644,-2.0172497837413));
#29275=CARTESIAN_POINT('Ctrl Pts',(-39.9467187504336,4.95855476116219,0.173156547826753));
#29276=CARTESIAN_POINT('Ctrl Pts',(-39.9202604171003,3.64393708624685,2.27698460548143));
#29277=CARTESIAN_POINT('Ctrl Pts',(-39.8938020837669,2.32931941133151,4.38081266313611));
#29278=CARTESIAN_POINT('Ctrl Pts',(-39.8673437504336,-0.149957969249583,
4.29423438922274));
#29279=CARTESIAN_POINT('Ctrl Pts',(-39.8408854171003,-2.62923534983068,
4.20765611530936));
#29280=CARTESIAN_POINT('Ctrl Pts',(-39.8144270837669,-3.79389505549643,
2.01724978374131));
#29281=CARTESIAN_POINT('Ctrl Pts',(-39.7879687504336,-4.95855476116219,
-0.173156547826752));
#29282=CARTESIAN_POINT('Ctrl Pts',(-39.7615104171003,-3.64393708624685,
-2.27698460548143));
#29283=CARTESIAN_POINT('Ctrl Pts',(-39.7350520837669,-2.32931941133151,
-4.38081266313611));
#29284=CARTESIAN_POINT('Ctrl Pts',(-39.7085937504336,0.149957969249583,
-4.29423438922274));
#29285=CARTESIAN_POINT('Ctrl Pts',(-39.6821354171003,2.62923534983068,-4.20765611530936));
#29286=CARTESIAN_POINT('Ctrl Pts',(-39.6556770837669,3.79389505549644,-2.0172497837413));
#29287=CARTESIAN_POINT('Ctrl Pts',(-39.6292187504336,4.95855476116219,0.173156547826753));
#29288=CARTESIAN_POINT('Ctrl Pts',(-39.6027604171003,3.64393708624685,2.27698460548143));
#29289=CARTESIAN_POINT('Ctrl Pts',(-39.5763020837669,2.32931941133151,4.38081266313611));
#29290=CARTESIAN_POINT('Ctrl Pts',(-39.5498437504336,-0.149957969249583,
4.29423438922274));
#29291=CARTESIAN_POINT('Ctrl Pts',(-39.5233854171003,-2.62923534983068,
4.20765611530936));
#29292=CARTESIAN_POINT('Ctrl Pts',(-39.4969270837669,-3.79389505549643,
2.01724978374131));
#29293=CARTESIAN_POINT('Ctrl Pts',(-39.4704687504336,-4.95855476116219,
-0.173156547826752));
#29294=CARTESIAN_POINT('Ctrl Pts',(-39.4440104171003,-3.64393708624685,
-2.27698460548143));
#29295=CARTESIAN_POINT('Ctrl Pts',(-39.4175520837669,-2.32931941133151,
-4.38081266313611));
#29296=CARTESIAN_POINT('Ctrl Pts',(-39.3910937504336,0.149957969249583,
-4.29423438922274));
#29297=CARTESIAN_POINT('Ctrl Pts',(-39.3646354171003,2.62923534983068,-4.20765611530936));
#29298=CARTESIAN_POINT('Ctrl Pts',(-39.3381770837669,3.79389505549644,-2.0172497837413));
#29299=CARTESIAN_POINT('Ctrl Pts',(-39.3117187504336,4.95855476116219,0.173156547826753));
#29300=CARTESIAN_POINT('Ctrl Pts',(-39.2852604171003,3.64393708624685,2.27698460548143));
#29301=CARTESIAN_POINT('Ctrl Pts',(-39.2588020837669,2.32931941133151,4.38081266313611));
#29302=CARTESIAN_POINT('Ctrl Pts',(-39.2323437504336,-0.149957969249583,
4.29423438922274));
#29303=CARTESIAN_POINT('Ctrl Pts',(-39.2058854171003,-2.62923534983068,
4.20765611530936));
#29304=CARTESIAN_POINT('Ctrl Pts',(-39.1794270837669,-3.79389505549643,
2.01724978374131));
#29305=CARTESIAN_POINT('Ctrl Pts',(-39.1529687504336,-4.95855476116219,
-0.173156547826752));
#29306=CARTESIAN_POINT('Ctrl Pts',(-39.1265104171003,-3.64393708624685,
-2.27698460548143));
#29307=CARTESIAN_POINT('Ctrl Pts',(-39.1000520837669,-2.32931941133151,
-4.38081266313611));
#29308=CARTESIAN_POINT('Ctrl Pts',(-39.0735937504336,0.149957969249583,
-4.29423438922274));
#29309=CARTESIAN_POINT('Ctrl Pts',(-39.0471354171003,2.62923534983068,-4.20765611530936));
#29310=CARTESIAN_POINT('Ctrl Pts',(-39.0206770837669,3.79389505549644,-2.0172497837413));
#29311=CARTESIAN_POINT('Ctrl Pts',(-38.9942187504336,4.95855476116219,0.173156547826753));
#29312=CARTESIAN_POINT('Ctrl Pts',(-38.9677604171003,3.64393708624685,2.27698460548143));
#29313=CARTESIAN_POINT('Ctrl Pts',(-38.9413020837669,2.32931941133151,4.38081266313611));
#29314=CARTESIAN_POINT('Ctrl Pts',(-38.9148437504336,-0.149957969249583,
4.29423438922274));
#29315=CARTESIAN_POINT('Ctrl Pts',(-38.8883854171003,-2.62923534983068,
4.20765611530936));
#29316=CARTESIAN_POINT('Ctrl Pts',(-38.8619270837669,-3.79389505549643,
2.01724978374131));
#29317=CARTESIAN_POINT('Ctrl Pts',(-38.8354687504336,-4.95855476116219,
-0.173156547826752));
#29318=CARTESIAN_POINT('Ctrl Pts',(-38.8090104171003,-3.64393708624685,
-2.27698460548143));
#29319=CARTESIAN_POINT('Ctrl Pts',(-38.7825520837669,-2.32931941133151,
-4.38081266313611));
#29320=CARTESIAN_POINT('Ctrl Pts',(-38.7560937504336,0.149957969249583,
-4.29423438922274));
#29321=CARTESIAN_POINT('Ctrl Pts',(-38.7296354171002,2.62923534983068,-4.20765611530936));
#29322=CARTESIAN_POINT('Ctrl Pts',(-38.7031770837669,3.79389505549644,-2.0172497837413));
#29323=CARTESIAN_POINT('Ctrl Pts',(-38.6767187504336,4.95855476116219,0.173156547826753));
#29324=CARTESIAN_POINT('Ctrl Pts',(-38.6502604171003,3.64393708624685,2.27698460548143));
#29325=CARTESIAN_POINT('Ctrl Pts',(-38.6238020837669,2.32931941133151,4.38081266313611));
#29326=CARTESIAN_POINT('Ctrl Pts',(-38.5973437504336,-0.149957969249583,
4.29423438922274));
#29327=CARTESIAN_POINT('Ctrl Pts',(-38.5708854171003,-2.62923534983068,
4.20765611530936));
#29328=CARTESIAN_POINT('Ctrl Pts',(-38.5444270837669,-3.79389505549643,
2.01724978374131));
#29329=CARTESIAN_POINT('Ctrl Pts',(-38.5179687504336,-4.95855476116219,
-0.173156547826752));
#29330=CARTESIAN_POINT('Ctrl Pts',(-38.4915104171003,-3.64393708624685,
-2.27698460548143));
#29331=CARTESIAN_POINT('Ctrl Pts',(-38.4650520837669,-2.32931941133151,
-4.38081266313611));
#29332=CARTESIAN_POINT('Ctrl Pts',(-38.4385937504336,0.149957969249583,
-4.29423438922274));
#29333=CARTESIAN_POINT('Ctrl Pts',(-38.4121354171003,2.62923534983068,-4.20765611530936));
#29334=CARTESIAN_POINT('Ctrl Pts',(-38.3856770837669,3.79389505549644,-2.0172497837413));
#29335=CARTESIAN_POINT('Ctrl Pts',(-38.3592187504336,4.95855476116219,0.173156547826753));
#29336=CARTESIAN_POINT('Ctrl Pts',(-38.3327604171003,3.64393708624685,2.27698460548143));
#29337=CARTESIAN_POINT('Ctrl Pts',(-38.3063020837669,2.32931941133151,4.38081266313611));
#29338=CARTESIAN_POINT('Ctrl Pts',(-38.2798437504336,-0.149957969249583,
4.29423438922274));
#29339=CARTESIAN_POINT('Ctrl Pts',(-38.2533854171003,-2.62923534983068,
4.20765611530936));
#29340=CARTESIAN_POINT('Ctrl Pts',(-38.2269270837669,-3.79389505549643,
2.01724978374131));
#29341=CARTESIAN_POINT('Ctrl Pts',(-38.2004687504336,-4.95855476116219,
-0.173156547826752));
#29342=CARTESIAN_POINT('Ctrl Pts',(-38.1740104171002,-3.64393708624685,
-2.27698460548143));
#29343=CARTESIAN_POINT('Ctrl Pts',(-38.1475520837669,-2.32931941133151,
-4.38081266313611));
#29344=CARTESIAN_POINT('Ctrl Pts',(-38.1210937504336,0.149957969249583,
-4.29423438922274));
#29345=CARTESIAN_POINT('Ctrl Pts',(-38.0946354171003,2.62923534983068,-4.20765611530936));
#29346=CARTESIAN_POINT('Ctrl Pts',(-38.0681770837669,3.79389505549644,-2.0172497837413));
#29347=CARTESIAN_POINT('Ctrl Pts',(-38.0417187504336,4.95855476116219,0.173156547826753));
#29348=CARTESIAN_POINT('Ctrl Pts',(-38.0152604171003,3.64393708624685,2.27698460548143));
#29349=CARTESIAN_POINT('Ctrl Pts',(-37.9888020837669,2.32931941133151,4.38081266313611));
#29350=CARTESIAN_POINT('Ctrl Pts',(-37.9623437504336,-0.149957969249583,
4.29423438922274));
#29351=CARTESIAN_POINT('Ctrl Pts',(-37.9358854171003,-2.62923534983068,
4.20765611530936));
#29352=CARTESIAN_POINT('Ctrl Pts',(-37.9094270837669,-3.79389505549643,
2.01724978374131));
#29353=CARTESIAN_POINT('Ctrl Pts',(-37.8829687504336,-4.95855476116219,
-0.173156547826752));
#29354=CARTESIAN_POINT('Ctrl Pts',(-37.8565104171003,-3.64393708624685,
-2.27698460548143));
#29355=CARTESIAN_POINT('Ctrl Pts',(-37.8300520837669,-2.32931941133151,
-4.38081266313611));
#29356=CARTESIAN_POINT('Ctrl Pts',(-37.8035937504336,0.149957969249583,
-4.29423438922274));
#29357=CARTESIAN_POINT('Ctrl Pts',(-37.7771354171003,2.62923534983068,-4.20765611530936));
#29358=CARTESIAN_POINT('Ctrl Pts',(-37.7506770837669,3.79389505549644,-2.0172497837413));
#29359=CARTESIAN_POINT('Ctrl Pts',(-37.7242187504336,4.95855476116219,0.173156547826753));
#29360=CARTESIAN_POINT('Ctrl Pts',(-37.6977604171003,3.64393708624685,2.27698460548143));
#29361=CARTESIAN_POINT('Ctrl Pts',(-37.6713020837669,2.32931941133151,4.38081266313611));
#29362=CARTESIAN_POINT('Ctrl Pts',(-37.6448437504336,-0.149957969249583,
4.29423438922274));
#29363=CARTESIAN_POINT('Ctrl Pts',(-37.6183854171003,-2.62923534983068,
4.20765611530936));
#29364=CARTESIAN_POINT('Ctrl Pts',(-37.5919270837669,-3.79389505549643,
2.01724978374131));
#29365=CARTESIAN_POINT('Ctrl Pts',(-37.5654687504336,-4.95855476116219,
-0.173156547826752));
#29366=CARTESIAN_POINT('Ctrl Pts',(-37.5390104171003,-3.64393708624685,
-2.27698460548143));
#29367=CARTESIAN_POINT('Ctrl Pts',(-37.5125520837669,-2.32931941133151,
-4.38081266313611));
#29368=CARTESIAN_POINT('Ctrl Pts',(-37.4860937504336,0.149957969249583,
-4.29423438922274));
#29369=CARTESIAN_POINT('Ctrl Pts',(-37.4596354171003,2.62923534983068,-4.20765611530936));
#29370=CARTESIAN_POINT('Ctrl Pts',(-37.4331770837669,3.79389505549644,-2.0172497837413));
#29371=CARTESIAN_POINT('Ctrl Pts',(-37.4067187504336,4.95855476116219,0.173156547826753));
#29372=CARTESIAN_POINT('Ctrl Pts',(-37.3802604171003,3.64393708624685,2.27698460548143));
#29373=CARTESIAN_POINT('Ctrl Pts',(-37.3538020837669,2.32931941133151,4.38081266313611));
#29374=CARTESIAN_POINT('Ctrl Pts',(-37.3273437504336,-0.149957969249583,
4.29423438922274));
#29375=CARTESIAN_POINT('Ctrl Pts',(-37.3008854171003,-2.62923534983068,
4.20765611530936));
#29376=CARTESIAN_POINT('Ctrl Pts',(-37.2744270837669,-3.79389505549643,
2.01724978374131));
#29377=CARTESIAN_POINT('Ctrl Pts',(-37.2479687504336,-4.95855476116219,
-0.173156547826752));
#29378=CARTESIAN_POINT('Ctrl Pts',(-37.2215104171003,-3.64393708624685,
-2.27698460548143));
#29379=CARTESIAN_POINT('Ctrl Pts',(-37.1950520837669,-2.32931941133151,
-4.38081266313611));
#29380=CARTESIAN_POINT('Ctrl Pts',(-37.1685937504336,0.149957969249583,
-4.29423438922274));
#29381=CARTESIAN_POINT('Ctrl Pts',(-37.1421354171003,2.62923534983068,-4.20765611530936));
#29382=CARTESIAN_POINT('Ctrl Pts',(-37.1156770837669,3.79389505549644,-2.0172497837413));
#29383=CARTESIAN_POINT('Ctrl Pts',(-37.0892187504336,4.95855476116219,0.173156547826753));
#29384=CARTESIAN_POINT('Ctrl Pts',(-37.0627604171003,3.64393708624685,2.27698460548143));
#29385=CARTESIAN_POINT('Ctrl Pts',(-37.0363020837669,2.32931941133151,4.38081266313611));
#29386=CARTESIAN_POINT('Ctrl Pts',(-37.0098437504336,-0.149957969249583,
4.29423438922274));
#29387=CARTESIAN_POINT('Ctrl Pts',(-36.9833854171003,-2.62923534983068,
4.20765611530936));
#29388=CARTESIAN_POINT('Ctrl Pts',(-36.9569270837669,-3.79389505549643,
2.01724978374131));
#29389=CARTESIAN_POINT('Ctrl Pts',(-36.9304687504336,-4.95855476116219,
-0.173156547826752));
#29390=CARTESIAN_POINT('Ctrl Pts',(-36.9040104171003,-3.64393708624685,
-2.27698460548143));
#29391=CARTESIAN_POINT('Ctrl Pts',(-36.8775520837669,-2.32931941133151,
-4.38081266313611));
#29392=CARTESIAN_POINT('Ctrl Pts',(-36.8510937504336,0.149957969249583,
-4.29423438922274));
#29393=CARTESIAN_POINT('Ctrl Pts',(-36.8246354171003,2.62923534983068,-4.20765611530936));
#29394=CARTESIAN_POINT('Ctrl Pts',(-36.7981770837669,3.79389505549644,-2.0172497837413));
#29395=CARTESIAN_POINT('Ctrl Pts',(-36.7717187504336,4.95855476116219,0.173156547826753));
#29396=CARTESIAN_POINT('Ctrl Pts',(-36.7452604171003,3.64393708624685,2.27698460548143));
#29397=CARTESIAN_POINT('Ctrl Pts',(-36.7188020837669,2.32931941133151,4.38081266313611));
#29398=CARTESIAN_POINT('Ctrl Pts',(-36.6923437504336,-0.149957969249583,
4.29423438922274));
#29399=CARTESIAN_POINT('Ctrl Pts',(-36.6658854171003,-2.62923534983068,
4.20765611530936));
#29400=CARTESIAN_POINT('Ctrl Pts',(-36.6394270837669,-3.79389505549643,
2.01724978374131));
#29401=CARTESIAN_POINT('Ctrl Pts',(-36.6129687504336,-4.95855476116219,
-0.173156547826752));
#29402=CARTESIAN_POINT('Ctrl Pts',(-36.5865104171002,-3.64393708624685,
-2.27698460548143));
#29403=CARTESIAN_POINT('Ctrl Pts',(-36.5600520837669,-2.32931941133151,
-4.38081266313611));
#29404=CARTESIAN_POINT('Ctrl Pts',(-36.5335937504336,0.149957969249583,
-4.29423438922274));
#29405=CARTESIAN_POINT('Ctrl Pts',(-36.5071354171003,2.62923534983068,-4.20765611530936));
#29406=CARTESIAN_POINT('Ctrl Pts',(-36.4806770837669,3.79389505549644,-2.0172497837413));
#29407=CARTESIAN_POINT('Ctrl Pts',(-36.4542187504336,4.95855476116219,0.173156547826753));
#29408=CARTESIAN_POINT('Ctrl Pts',(-36.4277604171003,3.64393708624685,2.27698460548143));
#29409=CARTESIAN_POINT('Ctrl Pts',(-36.4013020837669,2.32931941133151,4.38081266313611));
#29410=CARTESIAN_POINT('Ctrl Pts',(-36.3748437504336,-0.149957969249583,
4.29423438922274));
#29411=CARTESIAN_POINT('Ctrl Pts',(-36.3483854171003,-2.62923534983068,
4.20765611530936));
#29412=CARTESIAN_POINT('Ctrl Pts',(-36.3219270837669,-3.79389505549643,
2.01724978374131));
#29413=CARTESIAN_POINT('Ctrl Pts',(-36.2954687504336,-4.95855476116219,
-0.173156547826752));
#29414=CARTESIAN_POINT('Ctrl Pts',(-36.2690104171003,-3.64393708624685,
-2.27698460548143));
#29415=CARTESIAN_POINT('Ctrl Pts',(-36.2425520837669,-2.32931941133151,
-4.38081266313611));
#29416=CARTESIAN_POINT('Ctrl Pts',(-36.2160937504336,0.149957969249583,
-4.29423438922274));
#29417=CARTESIAN_POINT('Ctrl Pts',(-36.1896354171003,2.62923534983068,-4.20765611530936));
#29418=CARTESIAN_POINT('Ctrl Pts',(-36.1631770837669,3.79389505549644,-2.0172497837413));
#29419=CARTESIAN_POINT('Ctrl Pts',(-36.1367187504336,4.95855476116219,0.173156547826753));
#29420=CARTESIAN_POINT('Ctrl Pts',(-36.1102604171003,3.64393708624685,2.27698460548143));
#29421=CARTESIAN_POINT('Ctrl Pts',(-36.0838020837669,2.32931941133151,4.38081266313611));
#29422=CARTESIAN_POINT('Ctrl Pts',(-36.0573437504336,-0.149957969249583,
4.29423438922274));
#29423=CARTESIAN_POINT('Ctrl Pts',(-36.0308854171003,-2.62923534983068,
4.20765611530936));
#29424=CARTESIAN_POINT('Ctrl Pts',(-36.0044270837669,-3.79389505549643,
2.01724978374131));
#29425=CARTESIAN_POINT('Ctrl Pts',(-35.9779687504336,-4.95855476116219,
-0.173156547826752));
#29426=CARTESIAN_POINT('Ctrl Pts',(-35.9515104171003,-3.64393708624685,
-2.27698460548143));
#29427=CARTESIAN_POINT('Ctrl Pts',(-35.9250520837669,-2.32931941133151,
-4.38081266313611));
#29428=CARTESIAN_POINT('Ctrl Pts',(-35.8985937504336,0.149957969249583,
-4.29423438922274));
#29429=CARTESIAN_POINT('Ctrl Pts',(-35.8721354171003,2.62923534983068,-4.20765611530936));
#29430=CARTESIAN_POINT('Ctrl Pts',(-35.8456770837669,3.79389505549644,-2.0172497837413));
#29431=CARTESIAN_POINT('Ctrl Pts',(-35.8192187504336,4.95855476116219,0.173156547826753));
#29432=CARTESIAN_POINT('Ctrl Pts',(-35.7927604171002,3.64393708624685,2.27698460548143));
#29433=CARTESIAN_POINT('Ctrl Pts',(-35.7663020837669,2.32931941133151,4.38081266313611));
#29434=CARTESIAN_POINT('Ctrl Pts',(-35.7398437504336,-0.149957969249583,
4.29423438922274));
#29435=CARTESIAN_POINT('Ctrl Pts',(-35.7133854171003,-2.62923534983068,
4.20765611530936));
#29436=CARTESIAN_POINT('Ctrl Pts',(-35.6869270837669,-3.79389505549643,
2.01724978374131));
#29437=CARTESIAN_POINT('Ctrl Pts',(-35.6604687504336,-4.95855476116219,
-0.173156547826752));
#29438=CARTESIAN_POINT('Ctrl Pts',(-35.6340104171002,-3.64393708624685,
-2.27698460548143));
#29439=CARTESIAN_POINT('Ctrl Pts',(-35.6075520837669,-2.32931941133151,
-4.38081266313611));
#29440=CARTESIAN_POINT('Ctrl Pts',(-35.5810937504336,0.149957969249583,
-4.29423438922274));
#29441=CARTESIAN_POINT('Ctrl Pts',(-35.5546354171003,2.62923534983068,-4.20765611530936));
#29442=CARTESIAN_POINT('Ctrl Pts',(-35.5281770837669,3.79389505549644,-2.0172497837413));
#29443=CARTESIAN_POINT('Ctrl Pts',(-35.5017187504336,4.95855476116219,0.173156547826753));
#29444=CARTESIAN_POINT('Ctrl Pts',(-35.4752604171003,3.64393708624685,2.27698460548143));
#29445=CARTESIAN_POINT('Ctrl Pts',(-35.4488020837669,2.32931941133151,4.38081266313611));
#29446=CARTESIAN_POINT('Ctrl Pts',(-35.4223437504336,-0.149957969249583,
4.29423438922274));
#29447=CARTESIAN_POINT('Ctrl Pts',(-35.3958854171003,-2.62923534983068,
4.20765611530936));
#29448=CARTESIAN_POINT('Ctrl Pts',(-35.3694270837669,-3.79389505549643,
2.01724978374131));
#29449=CARTESIAN_POINT('Ctrl Pts',(-35.3429687504336,-4.95855476116219,
-0.173156547826752));
#29450=CARTESIAN_POINT('Ctrl Pts',(-35.3165104171003,-3.64393708624685,
-2.27698460548143));
#29451=CARTESIAN_POINT('Ctrl Pts',(-35.2900520837669,-2.32931941133151,
-4.38081266313611));
#29452=CARTESIAN_POINT('Ctrl Pts',(-35.2635937504336,0.149957969249583,
-4.29423438922274));
#29453=CARTESIAN_POINT('Ctrl Pts',(-35.2371354171003,2.62923534983068,-4.20765611530936));
#29454=CARTESIAN_POINT('Ctrl Pts',(-35.2106770837669,3.79389505549644,-2.0172497837413));
#29455=CARTESIAN_POINT('Ctrl Pts',(-35.1842187504336,4.95855476116219,0.173156547826753));
#29456=CARTESIAN_POINT('Ctrl Pts',(-35.1577604171003,3.64393708624685,2.27698460548143));
#29457=CARTESIAN_POINT('Ctrl Pts',(-35.1313020837669,2.32931941133151,4.38081266313611));
#29458=CARTESIAN_POINT('Ctrl Pts',(-35.1048437504336,-0.149957969249583,
4.29423438922274));
#29459=CARTESIAN_POINT('Ctrl Pts',(-35.0783854171003,-2.62923534983068,
4.20765611530936));
#29460=CARTESIAN_POINT('Ctrl Pts',(-35.0519270837669,-3.79389505549643,
2.01724978374131));
#29461=CARTESIAN_POINT('Ctrl Pts',(-35.0254687504336,-4.95855476116219,
-0.173156547826752));
#29462=CARTESIAN_POINT('Ctrl Pts',(-34.9990104171003,-3.64393708624685,
-2.27698460548143));
#29463=CARTESIAN_POINT('Ctrl Pts',(-34.9725520837669,-2.32931941133151,
-4.38081266313611));
#29464=CARTESIAN_POINT('Ctrl Pts',(-34.9460937504336,0.149957969249583,
-4.29423438922274));
#29465=CARTESIAN_POINT('Ctrl Pts',(-34.9196354171003,2.62923534983068,-4.20765611530936));
#29466=CARTESIAN_POINT('Ctrl Pts',(-34.8931770837669,3.79389505549644,-2.0172497837413));
#29467=CARTESIAN_POINT('Ctrl Pts',(-34.8667187504336,4.95855476116219,0.173156547826753));
#29468=CARTESIAN_POINT('Ctrl Pts',(-34.8402604171003,3.64393708624685,2.27698460548143));
#29469=CARTESIAN_POINT('Ctrl Pts',(-34.8138020837669,2.32931941133151,4.38081266313611));
#29470=CARTESIAN_POINT('Ctrl Pts',(-34.7873437504336,-0.149957969249583,
4.29423438922274));
#29471=CARTESIAN_POINT('Ctrl Pts',(-34.7608854171003,-2.62923534983068,
4.20765611530936));
#29472=CARTESIAN_POINT('Ctrl Pts',(-34.7344270837669,-3.79389505549643,
2.01724978374131));
#29473=CARTESIAN_POINT('Ctrl Pts',(-34.7079687504336,-4.95855476116219,
-0.173156547826752));
#29474=CARTESIAN_POINT('Ctrl Pts',(-34.6815104171003,-3.64393708624685,
-2.27698460548143));
#29475=CARTESIAN_POINT('Ctrl Pts',(-34.6550520837669,-2.32931941133151,
-4.38081266313611));
#29476=CARTESIAN_POINT('Ctrl Pts',(-34.6285937504336,0.149957969249583,
-4.29423438922274));
#29477=CARTESIAN_POINT('Ctrl Pts',(-34.6021354171003,2.62923534983068,-4.20765611530936));
#29478=CARTESIAN_POINT('Ctrl Pts',(-34.5756770837669,3.79389505549644,-2.0172497837413));
#29479=CARTESIAN_POINT('Ctrl Pts',(-34.5492187504336,4.95855476116219,0.173156547826753));
#29480=CARTESIAN_POINT('Ctrl Pts',(-34.5227604171003,3.64393708624685,2.27698460548143));
#29481=CARTESIAN_POINT('Ctrl Pts',(-34.4963020837669,2.32931941133151,4.38081266313611));
#29482=CARTESIAN_POINT('Ctrl Pts',(-34.4698437504336,-0.149957969249583,
4.29423438922274));
#29483=CARTESIAN_POINT('Ctrl Pts',(-34.4433854171002,-2.62923534983068,
4.20765611530936));
#29484=CARTESIAN_POINT('Ctrl Pts',(-34.4169270837669,-3.79389505549643,
2.01724978374131));
#29485=CARTESIAN_POINT('Ctrl Pts',(-34.3904687504336,-4.95855476116219,
-0.173156547826752));
#29486=CARTESIAN_POINT('Ctrl Pts',(-34.3640104171003,-3.64393708624685,
-2.27698460548143));
#29487=CARTESIAN_POINT('Ctrl Pts',(-34.3375520837669,-2.32931941133151,
-4.38081266313611));
#29488=CARTESIAN_POINT('Ctrl Pts',(-34.3110937504336,0.149957969249583,
-4.29423438922274));
#29489=CARTESIAN_POINT('Ctrl Pts',(-34.2846354171002,2.62923534983068,-4.20765611530936));
#29490=CARTESIAN_POINT('Ctrl Pts',(-34.2581770837669,3.79389505549644,-2.0172497837413));
#29491=CARTESIAN_POINT('Ctrl Pts',(-34.2317187504336,4.95855476116219,0.173156547826753));
#29492=CARTESIAN_POINT('Ctrl Pts',(-34.2052604171002,3.64393708624685,2.27698460548143));
#29493=CARTESIAN_POINT('Ctrl Pts',(-34.1788020837669,2.32931941133151,4.38081266313611));
#29494=CARTESIAN_POINT('Ctrl Pts',(-34.1523437504336,-0.149957969249583,
4.29423438922274));
#29495=CARTESIAN_POINT('Ctrl Pts',(-34.1258854171002,-2.62923534983068,
4.20765611530936));
#29496=CARTESIAN_POINT('Ctrl Pts',(-34.0994270837669,-3.79389505549643,
2.01724978374131));
#29497=CARTESIAN_POINT('Ctrl Pts',(-34.0729687504336,-4.95855476116219,
-0.173156547826752));
#29498=CARTESIAN_POINT('Ctrl Pts',(-34.0465104171003,-3.64393708624685,
-2.27698460548143));
#29499=CARTESIAN_POINT('Ctrl Pts',(-34.0200520837669,-2.32931941133151,
-4.38081266313611));
#29500=CARTESIAN_POINT('Ctrl Pts',(-33.9935937504336,0.149957969249583,
-4.29423438922274));
#29501=CARTESIAN_POINT('Ctrl Pts',(-33.9671354171003,2.62923534983068,-4.20765611530936));
#29502=CARTESIAN_POINT('Ctrl Pts',(-33.9406770837669,3.79389505549644,-2.0172497837413));
#29503=CARTESIAN_POINT('Ctrl Pts',(-33.9142187504336,4.95855476116219,0.173156547826753));
#29504=CARTESIAN_POINT('Ctrl Pts',(-33.8877604171003,3.64393708624685,2.27698460548143));
#29505=CARTESIAN_POINT('Ctrl Pts',(-33.8620525212145,2.36660589948903,4.32114180867095));
#29506=CARTESIAN_POINT('Ctrl Pts',(-33.8359853668364,-0.0436954904407579,
4.29662973576265));
#29507=CARTESIAN_POINT('Ctrl Pts',(-43.7368750008672,0.143960423897816,
-4.12248716145376));
#29508=CARTESIAN_POINT('Ctrl Pts',(-43.7104166675338,2.52407949629392,-4.03937157196371));
#29509=CARTESIAN_POINT('Ctrl Pts',(-43.6839583342005,3.64215882054307,-1.9365701964918));
#29510=CARTESIAN_POINT('Ctrl Pts',(-43.6575000008672,4.76023814479221,0.166231178980113));
#29511=CARTESIAN_POINT('Ctrl Pts',(-43.6310416675338,3.49819839664525,2.18591696496197));
#29512=CARTESIAN_POINT('Ctrl Pts',(-43.6045833342005,2.23615864849829,4.20560275094382));
#29513=CARTESIAN_POINT('Ctrl Pts',(-43.5781250008672,-0.143960423897816,
4.12248716145376));
#29514=CARTESIAN_POINT('Ctrl Pts',(-43.5516666675338,-2.52407949629392,
4.03937157196371));
#29515=CARTESIAN_POINT('Ctrl Pts',(-43.5252083342005,-3.64215882054307,
1.9365701964918));
#29516=CARTESIAN_POINT('Ctrl Pts',(-43.4987500008672,-4.76023814479221,
-0.166231178980113));
#29517=CARTESIAN_POINT('Ctrl Pts',(-43.4722916675338,-3.49819839664525,
-2.18591696496196));
#29518=CARTESIAN_POINT('Ctrl Pts',(-43.4458333342005,-2.23615864849829,
-4.20560275094382));
#29519=CARTESIAN_POINT('Ctrl Pts',(-43.4193750008672,0.143960423897816,
-4.12248716145376));
#29520=CARTESIAN_POINT('Ctrl Pts',(-43.3929166675338,2.52407949629392,-4.03937157196371));
#29521=CARTESIAN_POINT('Ctrl Pts',(-43.3664583342005,3.64215882054307,-1.9365701964918));
#29522=CARTESIAN_POINT('Ctrl Pts',(-43.3400000008672,4.76023814479221,0.166231178980113));
#29523=CARTESIAN_POINT('Ctrl Pts',(-43.3135416675338,3.49819839664525,2.18591696496197));
#29524=CARTESIAN_POINT('Ctrl Pts',(-43.2870833342005,2.23615864849829,4.20560275094382));
#29525=CARTESIAN_POINT('Ctrl Pts',(-43.2606250008672,-0.143960423897816,
4.12248716145376));
#29526=CARTESIAN_POINT('Ctrl Pts',(-43.2341666675338,-2.52407949629392,
4.03937157196371));
#29527=CARTESIAN_POINT('Ctrl Pts',(-43.2077083342005,-3.64215882054307,
1.9365701964918));
#29528=CARTESIAN_POINT('Ctrl Pts',(-43.1812500008672,-4.76023814479221,
-0.166231178980113));
#29529=CARTESIAN_POINT('Ctrl Pts',(-43.1547916675338,-3.49819839664525,
-2.18591696496196));
#29530=CARTESIAN_POINT('Ctrl Pts',(-43.1283333342005,-2.23615864849829,
-4.20560275094382));
#29531=CARTESIAN_POINT('Ctrl Pts',(-43.1018750008672,0.143960423897816,
-4.12248716145376));
#29532=CARTESIAN_POINT('Ctrl Pts',(-43.0754166675338,2.52407949629392,-4.03937157196371));
#29533=CARTESIAN_POINT('Ctrl Pts',(-43.0489583342005,3.64215882054307,-1.9365701964918));
#29534=CARTESIAN_POINT('Ctrl Pts',(-43.0225000008672,4.76023814479221,0.166231178980113));
#29535=CARTESIAN_POINT('Ctrl Pts',(-42.9960416675338,3.49819839664525,2.18591696496197));
#29536=CARTESIAN_POINT('Ctrl Pts',(-42.9695833342005,2.23615864849829,4.20560275094382));
#29537=CARTESIAN_POINT('Ctrl Pts',(-42.9431250008672,-0.143960423897816,
4.12248716145376));
#29538=CARTESIAN_POINT('Ctrl Pts',(-42.9166666675338,-2.52407949629392,
4.03937157196371));
#29539=CARTESIAN_POINT('Ctrl Pts',(-42.8902083342005,-3.64215882054307,
1.9365701964918));
#29540=CARTESIAN_POINT('Ctrl Pts',(-42.8637500008672,-4.76023814479221,
-0.166231178980113));
#29541=CARTESIAN_POINT('Ctrl Pts',(-42.8372916675338,-3.49819839664525,
-2.18591696496196));
#29542=CARTESIAN_POINT('Ctrl Pts',(-42.8108333342005,-2.23615864849829,
-4.20560275094382));
#29543=CARTESIAN_POINT('Ctrl Pts',(-42.7843750008672,0.143960423897816,
-4.12248716145376));
#29544=CARTESIAN_POINT('Ctrl Pts',(-42.7579166675338,2.52407949629392,-4.03937157196371));
#29545=CARTESIAN_POINT('Ctrl Pts',(-42.7314583342005,3.64215882054307,-1.9365701964918));
#29546=CARTESIAN_POINT('Ctrl Pts',(-42.7050000008672,4.76023814479221,0.166231178980113));
#29547=CARTESIAN_POINT('Ctrl Pts',(-42.6785416675338,3.49819839664525,2.18591696496197));
#29548=CARTESIAN_POINT('Ctrl Pts',(-42.6520833342005,2.23615864849829,4.20560275094382));
#29549=CARTESIAN_POINT('Ctrl Pts',(-42.6256250008672,-0.143960423897816,
4.12248716145376));
#29550=CARTESIAN_POINT('Ctrl Pts',(-42.5991666675338,-2.52407949629392,
4.03937157196371));
#29551=CARTESIAN_POINT('Ctrl Pts',(-42.5727083342005,-3.64215882054307,
1.9365701964918));
#29552=CARTESIAN_POINT('Ctrl Pts',(-42.5462500008672,-4.76023814479221,
-0.166231178980113));
#29553=CARTESIAN_POINT('Ctrl Pts',(-42.5197916675338,-3.49819839664525,
-2.18591696496196));
#29554=CARTESIAN_POINT('Ctrl Pts',(-42.4933333342005,-2.23615864849829,
-4.20560275094382));
#29555=CARTESIAN_POINT('Ctrl Pts',(-42.4668750008672,0.143960423897816,
-4.12248716145376));
#29556=CARTESIAN_POINT('Ctrl Pts',(-42.4404166675338,2.52407949629392,-4.03937157196371));
#29557=CARTESIAN_POINT('Ctrl Pts',(-42.4139583342005,3.64215882054307,-1.9365701964918));
#29558=CARTESIAN_POINT('Ctrl Pts',(-42.3875000008672,4.76023814479221,0.166231178980113));
#29559=CARTESIAN_POINT('Ctrl Pts',(-42.3610416675338,3.49819839664525,2.18591696496197));
#29560=CARTESIAN_POINT('Ctrl Pts',(-42.3345833342005,2.23615864849829,4.20560275094382));
#29561=CARTESIAN_POINT('Ctrl Pts',(-42.3081250008672,-0.143960423897816,
4.12248716145376));
#29562=CARTESIAN_POINT('Ctrl Pts',(-42.2816666675338,-2.52407949629392,
4.03937157196371));
#29563=CARTESIAN_POINT('Ctrl Pts',(-42.2552083342005,-3.64215882054307,
1.9365701964918));
#29564=CARTESIAN_POINT('Ctrl Pts',(-42.2287500008672,-4.76023814479221,
-0.166231178980113));
#29565=CARTESIAN_POINT('Ctrl Pts',(-42.2022916675338,-3.49819839664525,
-2.18591696496196));
#29566=CARTESIAN_POINT('Ctrl Pts',(-42.1758333342005,-2.23615864849829,
-4.20560275094382));
#29567=CARTESIAN_POINT('Ctrl Pts',(-42.1493750008672,0.143960423897816,
-4.12248716145376));
#29568=CARTESIAN_POINT('Ctrl Pts',(-42.1229166675338,2.52407949629392,-4.03937157196371));
#29569=CARTESIAN_POINT('Ctrl Pts',(-42.0964583342005,3.64215882054307,-1.9365701964918));
#29570=CARTESIAN_POINT('Ctrl Pts',(-42.0700000008672,4.76023814479221,0.166231178980113));
#29571=CARTESIAN_POINT('Ctrl Pts',(-42.0435416675338,3.49819839664525,2.18591696496197));
#29572=CARTESIAN_POINT('Ctrl Pts',(-42.0170833342005,2.23615864849829,4.20560275094382));
#29573=CARTESIAN_POINT('Ctrl Pts',(-41.9906250008672,-0.143960423897816,
4.12248716145376));
#29574=CARTESIAN_POINT('Ctrl Pts',(-41.9641666675338,-2.52407949629392,
4.03937157196371));
#29575=CARTESIAN_POINT('Ctrl Pts',(-41.9377083342005,-3.64215882054307,
1.9365701964918));
#29576=CARTESIAN_POINT('Ctrl Pts',(-41.9112500008672,-4.76023814479221,
-0.166231178980113));
#29577=CARTESIAN_POINT('Ctrl Pts',(-41.8847916675338,-3.49819839664525,
-2.18591696496196));
#29578=CARTESIAN_POINT('Ctrl Pts',(-41.8583333342005,-2.23615864849829,
-4.20560275094382));
#29579=CARTESIAN_POINT('Ctrl Pts',(-41.8318750008672,0.143960423897816,
-4.12248716145376));
#29580=CARTESIAN_POINT('Ctrl Pts',(-41.8054166675338,2.52407949629392,-4.03937157196371));
#29581=CARTESIAN_POINT('Ctrl Pts',(-41.7789583342005,3.64215882054307,-1.9365701964918));
#29582=CARTESIAN_POINT('Ctrl Pts',(-41.7525000008672,4.76023814479221,0.166231178980113));
#29583=CARTESIAN_POINT('Ctrl Pts',(-41.7260416675338,3.49819839664525,2.18591696496197));
#29584=CARTESIAN_POINT('Ctrl Pts',(-41.6995833342005,2.23615864849829,4.20560275094382));
#29585=CARTESIAN_POINT('Ctrl Pts',(-41.6731250008672,-0.143960423897816,
4.12248716145376));
#29586=CARTESIAN_POINT('Ctrl Pts',(-41.6466666675338,-2.52407949629392,
4.03937157196371));
#29587=CARTESIAN_POINT('Ctrl Pts',(-41.6202083342005,-3.64215882054307,
1.9365701964918));
#29588=CARTESIAN_POINT('Ctrl Pts',(-41.5937500008672,-4.76023814479221,
-0.166231178980113));
#29589=CARTESIAN_POINT('Ctrl Pts',(-41.5672916675338,-3.49819839664525,
-2.18591696496196));
#29590=CARTESIAN_POINT('Ctrl Pts',(-41.5408333342005,-2.23615864849829,
-4.20560275094382));
#29591=CARTESIAN_POINT('Ctrl Pts',(-41.5143750008672,0.143960423897816,
-4.12248716145376));
#29592=CARTESIAN_POINT('Ctrl Pts',(-41.4879166675338,2.52407949629392,-4.03937157196371));
#29593=CARTESIAN_POINT('Ctrl Pts',(-41.4614583342005,3.64215882054307,-1.9365701964918));
#29594=CARTESIAN_POINT('Ctrl Pts',(-41.4350000008672,4.76023814479221,0.166231178980113));
#29595=CARTESIAN_POINT('Ctrl Pts',(-41.4085416675338,3.49819839664525,2.18591696496197));
#29596=CARTESIAN_POINT('Ctrl Pts',(-41.3820833342005,2.23615864849829,4.20560275094382));
#29597=CARTESIAN_POINT('Ctrl Pts',(-41.3556250008672,-0.143960423897816,
4.12248716145376));
#29598=CARTESIAN_POINT('Ctrl Pts',(-41.3291666675338,-2.52407949629392,
4.03937157196371));
#29599=CARTESIAN_POINT('Ctrl Pts',(-41.3027083342005,-3.64215882054307,
1.9365701964918));
#29600=CARTESIAN_POINT('Ctrl Pts',(-41.2762500008672,-4.76023814479221,
-0.166231178980113));
#29601=CARTESIAN_POINT('Ctrl Pts',(-41.2497916675338,-3.49819839664525,
-2.18591696496196));
#29602=CARTESIAN_POINT('Ctrl Pts',(-41.2233333342005,-2.23615864849829,
-4.20560275094382));
#29603=CARTESIAN_POINT('Ctrl Pts',(-41.1968750008672,0.143960423897816,
-4.12248716145376));
#29604=CARTESIAN_POINT('Ctrl Pts',(-41.1704166675338,2.52407949629392,-4.03937157196371));
#29605=CARTESIAN_POINT('Ctrl Pts',(-41.1439583342005,3.64215882054307,-1.9365701964918));
#29606=CARTESIAN_POINT('Ctrl Pts',(-41.1175000008672,4.76023814479221,0.166231178980113));
#29607=CARTESIAN_POINT('Ctrl Pts',(-41.0910416675338,3.49819839664525,2.18591696496197));
#29608=CARTESIAN_POINT('Ctrl Pts',(-41.0645833342005,2.23615864849829,4.20560275094382));
#29609=CARTESIAN_POINT('Ctrl Pts',(-41.0381250008672,-0.143960423897816,
4.12248716145376));
#29610=CARTESIAN_POINT('Ctrl Pts',(-41.0116666675338,-2.52407949629392,
4.03937157196371));
#29611=CARTESIAN_POINT('Ctrl Pts',(-40.9852083342005,-3.64215882054307,
1.9365701964918));
#29612=CARTESIAN_POINT('Ctrl Pts',(-40.9587500008672,-4.76023814479221,
-0.166231178980113));
#29613=CARTESIAN_POINT('Ctrl Pts',(-40.9322916675338,-3.49819839664525,
-2.18591696496196));
#29614=CARTESIAN_POINT('Ctrl Pts',(-40.9058333342005,-2.23615864849829,
-4.20560275094382));
#29615=CARTESIAN_POINT('Ctrl Pts',(-40.8793750008672,0.143960423897816,
-4.12248716145376));
#29616=CARTESIAN_POINT('Ctrl Pts',(-40.8529166675338,2.52407949629392,-4.03937157196371));
#29617=CARTESIAN_POINT('Ctrl Pts',(-40.8264583342005,3.64215882054307,-1.9365701964918));
#29618=CARTESIAN_POINT('Ctrl Pts',(-40.8000000008672,4.76023814479221,0.166231178980113));
#29619=CARTESIAN_POINT('Ctrl Pts',(-40.7735416675338,3.49819839664525,2.18591696496197));
#29620=CARTESIAN_POINT('Ctrl Pts',(-40.7470833342005,2.23615864849829,4.20560275094382));
#29621=CARTESIAN_POINT('Ctrl Pts',(-40.7206250008672,-0.143960423897816,
4.12248716145376));
#29622=CARTESIAN_POINT('Ctrl Pts',(-40.6941666675338,-2.52407949629392,
4.03937157196371));
#29623=CARTESIAN_POINT('Ctrl Pts',(-40.6677083342005,-3.64215882054307,
1.9365701964918));
#29624=CARTESIAN_POINT('Ctrl Pts',(-40.6412500008672,-4.76023814479221,
-0.166231178980113));
#29625=CARTESIAN_POINT('Ctrl Pts',(-40.6147916675338,-3.49819839664525,
-2.18591696496196));
#29626=CARTESIAN_POINT('Ctrl Pts',(-40.5883333342005,-2.23615864849829,
-4.20560275094382));
#29627=CARTESIAN_POINT('Ctrl Pts',(-40.5618750008672,0.143960423897816,
-4.12248716145376));
#29628=CARTESIAN_POINT('Ctrl Pts',(-40.5354166675338,2.52407949629392,-4.03937157196371));
#29629=CARTESIAN_POINT('Ctrl Pts',(-40.5089583342005,3.64215882054307,-1.9365701964918));
#29630=CARTESIAN_POINT('Ctrl Pts',(-40.4825000008672,4.76023814479221,0.166231178980113));
#29631=CARTESIAN_POINT('Ctrl Pts',(-40.4560416675338,3.49819839664525,2.18591696496197));
#29632=CARTESIAN_POINT('Ctrl Pts',(-40.4295833342005,2.23615864849829,4.20560275094382));
#29633=CARTESIAN_POINT('Ctrl Pts',(-40.4031250008672,-0.143960423897816,
4.12248716145376));
#29634=CARTESIAN_POINT('Ctrl Pts',(-40.3766666675338,-2.52407949629392,
4.03937157196371));
#29635=CARTESIAN_POINT('Ctrl Pts',(-40.3502083342005,-3.64215882054307,
1.9365701964918));
#29636=CARTESIAN_POINT('Ctrl Pts',(-40.3237500008672,-4.76023814479221,
-0.166231178980113));
#29637=CARTESIAN_POINT('Ctrl Pts',(-40.2972916675338,-3.49819839664525,
-2.18591696496196));
#29638=CARTESIAN_POINT('Ctrl Pts',(-40.2708333342005,-2.23615864849829,
-4.20560275094382));
#29639=CARTESIAN_POINT('Ctrl Pts',(-40.2443750008672,0.143960423897816,
-4.12248716145376));
#29640=CARTESIAN_POINT('Ctrl Pts',(-40.2179166675338,2.52407949629392,-4.03937157196371));
#29641=CARTESIAN_POINT('Ctrl Pts',(-40.1914583342005,3.64215882054307,-1.9365701964918));
#29642=CARTESIAN_POINT('Ctrl Pts',(-40.1650000008672,4.76023814479221,0.166231178980113));
#29643=CARTESIAN_POINT('Ctrl Pts',(-40.1385416675338,3.49819839664525,2.18591696496197));
#29644=CARTESIAN_POINT('Ctrl Pts',(-40.1120833342005,2.23615864849829,4.20560275094382));
#29645=CARTESIAN_POINT('Ctrl Pts',(-40.0856250008672,-0.143960423897816,
4.12248716145376));
#29646=CARTESIAN_POINT('Ctrl Pts',(-40.0591666675338,-2.52407949629392,
4.03937157196371));
#29647=CARTESIAN_POINT('Ctrl Pts',(-40.0327083342005,-3.64215882054307,
1.9365701964918));
#29648=CARTESIAN_POINT('Ctrl Pts',(-40.0062500008672,-4.76023814479221,
-0.166231178980113));
#29649=CARTESIAN_POINT('Ctrl Pts',(-39.9797916675338,-3.49819839664525,
-2.18591696496196));
#29650=CARTESIAN_POINT('Ctrl Pts',(-39.9533333342005,-2.23615864849829,
-4.20560275094382));
#29651=CARTESIAN_POINT('Ctrl Pts',(-39.9268750008672,0.143960423897816,
-4.12248716145376));
#29652=CARTESIAN_POINT('Ctrl Pts',(-39.9004166675338,2.52407949629392,-4.03937157196371));
#29653=CARTESIAN_POINT('Ctrl Pts',(-39.8739583342005,3.64215882054307,-1.9365701964918));
#29654=CARTESIAN_POINT('Ctrl Pts',(-39.8475000008672,4.76023814479221,0.166231178980113));
#29655=CARTESIAN_POINT('Ctrl Pts',(-39.8210416675338,3.49819839664525,2.18591696496197));
#29656=CARTESIAN_POINT('Ctrl Pts',(-39.7945833342005,2.23615864849829,4.20560275094382));
#29657=CARTESIAN_POINT('Ctrl Pts',(-39.7681250008672,-0.143960423897816,
4.12248716145376));
#29658=CARTESIAN_POINT('Ctrl Pts',(-39.7416666675338,-2.52407949629392,
4.03937157196371));
#29659=CARTESIAN_POINT('Ctrl Pts',(-39.7152083342005,-3.64215882054307,
1.9365701964918));
#29660=CARTESIAN_POINT('Ctrl Pts',(-39.6887500008672,-4.76023814479221,
-0.166231178980113));
#29661=CARTESIAN_POINT('Ctrl Pts',(-39.6622916675338,-3.49819839664525,
-2.18591696496196));
#29662=CARTESIAN_POINT('Ctrl Pts',(-39.6358333342005,-2.23615864849829,
-4.20560275094382));
#29663=CARTESIAN_POINT('Ctrl Pts',(-39.6093750008672,0.143960423897816,
-4.12248716145376));
#29664=CARTESIAN_POINT('Ctrl Pts',(-39.5829166675338,2.52407949629392,-4.03937157196371));
#29665=CARTESIAN_POINT('Ctrl Pts',(-39.5564583342005,3.64215882054307,-1.9365701964918));
#29666=CARTESIAN_POINT('Ctrl Pts',(-39.5300000008672,4.76023814479221,0.166231178980113));
#29667=CARTESIAN_POINT('Ctrl Pts',(-39.5035416675338,3.49819839664525,2.18591696496197));
#29668=CARTESIAN_POINT('Ctrl Pts',(-39.4770833342005,2.23615864849829,4.20560275094382));
#29669=CARTESIAN_POINT('Ctrl Pts',(-39.4506250008672,-0.143960423897816,
4.12248716145376));
#29670=CARTESIAN_POINT('Ctrl Pts',(-39.4241666675338,-2.52407949629392,
4.03937157196371));
#29671=CARTESIAN_POINT('Ctrl Pts',(-39.3977083342005,-3.64215882054307,
1.9365701964918));
#29672=CARTESIAN_POINT('Ctrl Pts',(-39.3712500008672,-4.76023814479221,
-0.166231178980113));
#29673=CARTESIAN_POINT('Ctrl Pts',(-39.3447916675338,-3.49819839664525,
-2.18591696496196));
#29674=CARTESIAN_POINT('Ctrl Pts',(-39.3183333342005,-2.23615864849829,
-4.20560275094382));
#29675=CARTESIAN_POINT('Ctrl Pts',(-39.2918750008672,0.143960423897816,
-4.12248716145376));
#29676=CARTESIAN_POINT('Ctrl Pts',(-39.2654166675338,2.52407949629392,-4.03937157196371));
#29677=CARTESIAN_POINT('Ctrl Pts',(-39.2389583342005,3.64215882054307,-1.9365701964918));
#29678=CARTESIAN_POINT('Ctrl Pts',(-39.2125000008672,4.76023814479221,0.166231178980113));
#29679=CARTESIAN_POINT('Ctrl Pts',(-39.1860416675338,3.49819839664525,2.18591696496197));
#29680=CARTESIAN_POINT('Ctrl Pts',(-39.1595833342005,2.23615864849829,4.20560275094382));
#29681=CARTESIAN_POINT('Ctrl Pts',(-39.1331250008672,-0.143960423897816,
4.12248716145376));
#29682=CARTESIAN_POINT('Ctrl Pts',(-39.1066666675338,-2.52407949629392,
4.03937157196371));
#29683=CARTESIAN_POINT('Ctrl Pts',(-39.0802083342005,-3.64215882054307,
1.9365701964918));
#29684=CARTESIAN_POINT('Ctrl Pts',(-39.0537500008672,-4.76023814479221,
-0.166231178980113));
#29685=CARTESIAN_POINT('Ctrl Pts',(-39.0272916675338,-3.49819839664525,
-2.18591696496196));
#29686=CARTESIAN_POINT('Ctrl Pts',(-39.0008333342005,-2.23615864849829,
-4.20560275094382));
#29687=CARTESIAN_POINT('Ctrl Pts',(-38.9743750008672,0.143960423897816,
-4.12248716145376));
#29688=CARTESIAN_POINT('Ctrl Pts',(-38.9479166675338,2.52407949629392,-4.03937157196371));
#29689=CARTESIAN_POINT('Ctrl Pts',(-38.9214583342005,3.64215882054307,-1.9365701964918));
#29690=CARTESIAN_POINT('Ctrl Pts',(-38.8950000008672,4.76023814479221,0.166231178980113));
#29691=CARTESIAN_POINT('Ctrl Pts',(-38.8685416675338,3.49819839664525,2.18591696496197));
#29692=CARTESIAN_POINT('Ctrl Pts',(-38.8420833342005,2.23615864849829,4.20560275094382));
#29693=CARTESIAN_POINT('Ctrl Pts',(-38.8156250008672,-0.143960423897816,
4.12248716145376));
#29694=CARTESIAN_POINT('Ctrl Pts',(-38.7891666675338,-2.52407949629392,
4.03937157196371));
#29695=CARTESIAN_POINT('Ctrl Pts',(-38.7627083342005,-3.64215882054307,
1.9365701964918));
#29696=CARTESIAN_POINT('Ctrl Pts',(-38.7362500008672,-4.76023814479221,
-0.166231178980113));
#29697=CARTESIAN_POINT('Ctrl Pts',(-38.7097916675338,-3.49819839664525,
-2.18591696496196));
#29698=CARTESIAN_POINT('Ctrl Pts',(-38.6833333342005,-2.23615864849829,
-4.20560275094382));
#29699=CARTESIAN_POINT('Ctrl Pts',(-38.6568750008672,0.143960423897816,
-4.12248716145376));
#29700=CARTESIAN_POINT('Ctrl Pts',(-38.6304166675338,2.52407949629392,-4.03937157196371));
#29701=CARTESIAN_POINT('Ctrl Pts',(-38.6039583342005,3.64215882054307,-1.9365701964918));
#29702=CARTESIAN_POINT('Ctrl Pts',(-38.5775000008672,4.76023814479221,0.166231178980113));
#29703=CARTESIAN_POINT('Ctrl Pts',(-38.5510416675338,3.49819839664525,2.18591696496197));
#29704=CARTESIAN_POINT('Ctrl Pts',(-38.5245833342005,2.23615864849829,4.20560275094382));
#29705=CARTESIAN_POINT('Ctrl Pts',(-38.4981250008672,-0.143960423897816,
4.12248716145376));
#29706=CARTESIAN_POINT('Ctrl Pts',(-38.4716666675338,-2.52407949629392,
4.03937157196371));
#29707=CARTESIAN_POINT('Ctrl Pts',(-38.4452083342005,-3.64215882054307,
1.9365701964918));
#29708=CARTESIAN_POINT('Ctrl Pts',(-38.4187500008672,-4.76023814479221,
-0.166231178980113));
#29709=CARTESIAN_POINT('Ctrl Pts',(-38.3922916675338,-3.49819839664525,
-2.18591696496196));
#29710=CARTESIAN_POINT('Ctrl Pts',(-38.3658333342005,-2.23615864849829,
-4.20560275094382));
#29711=CARTESIAN_POINT('Ctrl Pts',(-38.3393750008672,0.143960423897816,
-4.12248716145376));
#29712=CARTESIAN_POINT('Ctrl Pts',(-38.3129166675338,2.52407949629392,-4.03937157196371));
#29713=CARTESIAN_POINT('Ctrl Pts',(-38.2864583342005,3.64215882054307,-1.9365701964918));
#29714=CARTESIAN_POINT('Ctrl Pts',(-38.2600000008672,4.76023814479221,0.166231178980113));
#29715=CARTESIAN_POINT('Ctrl Pts',(-38.2335416675338,3.49819839664525,2.18591696496197));
#29716=CARTESIAN_POINT('Ctrl Pts',(-38.2070833342005,2.23615864849829,4.20560275094382));
#29717=CARTESIAN_POINT('Ctrl Pts',(-38.1806250008672,-0.143960423897816,
4.12248716145376));
#29718=CARTESIAN_POINT('Ctrl Pts',(-38.1541666675338,-2.52407949629392,
4.03937157196371));
#29719=CARTESIAN_POINT('Ctrl Pts',(-38.1277083342005,-3.64215882054307,
1.9365701964918));
#29720=CARTESIAN_POINT('Ctrl Pts',(-38.1012500008672,-4.76023814479221,
-0.166231178980113));
#29721=CARTESIAN_POINT('Ctrl Pts',(-38.0747916675338,-3.49819839664525,
-2.18591696496196));
#29722=CARTESIAN_POINT('Ctrl Pts',(-38.0483333342005,-2.23615864849829,
-4.20560275094382));
#29723=CARTESIAN_POINT('Ctrl Pts',(-38.0218750008672,0.143960423897816,
-4.12248716145376));
#29724=CARTESIAN_POINT('Ctrl Pts',(-37.9954166675338,2.52407949629392,-4.03937157196371));
#29725=CARTESIAN_POINT('Ctrl Pts',(-37.9689583342005,3.64215882054307,-1.9365701964918));
#29726=CARTESIAN_POINT('Ctrl Pts',(-37.9425000008672,4.76023814479221,0.166231178980113));
#29727=CARTESIAN_POINT('Ctrl Pts',(-37.9160416675338,3.49819839664525,2.18591696496197));
#29728=CARTESIAN_POINT('Ctrl Pts',(-37.8895833342005,2.23615864849829,4.20560275094382));
#29729=CARTESIAN_POINT('Ctrl Pts',(-37.8631250008672,-0.143960423897816,
4.12248716145376));
#29730=CARTESIAN_POINT('Ctrl Pts',(-37.8366666675338,-2.52407949629392,
4.03937157196371));
#29731=CARTESIAN_POINT('Ctrl Pts',(-37.8102083342005,-3.64215882054307,
1.9365701964918));
#29732=CARTESIAN_POINT('Ctrl Pts',(-37.7837500008672,-4.76023814479221,
-0.166231178980113));
#29733=CARTESIAN_POINT('Ctrl Pts',(-37.7572916675338,-3.49819839664525,
-2.18591696496196));
#29734=CARTESIAN_POINT('Ctrl Pts',(-37.7308333342005,-2.23615864849829,
-4.20560275094382));
#29735=CARTESIAN_POINT('Ctrl Pts',(-37.7043750008672,0.143960423897816,
-4.12248716145376));
#29736=CARTESIAN_POINT('Ctrl Pts',(-37.6779166675338,2.52407949629392,-4.03937157196371));
#29737=CARTESIAN_POINT('Ctrl Pts',(-37.6514583342005,3.64215882054307,-1.9365701964918));
#29738=CARTESIAN_POINT('Ctrl Pts',(-37.6250000008672,4.76023814479221,0.166231178980113));
#29739=CARTESIAN_POINT('Ctrl Pts',(-37.5985416675338,3.49819839664525,2.18591696496197));
#29740=CARTESIAN_POINT('Ctrl Pts',(-37.5720833342005,2.23615864849829,4.20560275094382));
#29741=CARTESIAN_POINT('Ctrl Pts',(-37.5456250008672,-0.143960423897816,
4.12248716145376));
#29742=CARTESIAN_POINT('Ctrl Pts',(-37.5191666675338,-2.52407949629392,
4.03937157196371));
#29743=CARTESIAN_POINT('Ctrl Pts',(-37.4927083342005,-3.64215882054307,
1.9365701964918));
#29744=CARTESIAN_POINT('Ctrl Pts',(-37.4662500008672,-4.76023814479221,
-0.166231178980113));
#29745=CARTESIAN_POINT('Ctrl Pts',(-37.4397916675338,-3.49819839664525,
-2.18591696496196));
#29746=CARTESIAN_POINT('Ctrl Pts',(-37.4133333342005,-2.23615864849829,
-4.20560275094382));
#29747=CARTESIAN_POINT('Ctrl Pts',(-37.3868750008672,0.143960423897816,
-4.12248716145376));
#29748=CARTESIAN_POINT('Ctrl Pts',(-37.3604166675338,2.52407949629392,-4.03937157196371));
#29749=CARTESIAN_POINT('Ctrl Pts',(-37.3339583342005,3.64215882054307,-1.9365701964918));
#29750=CARTESIAN_POINT('Ctrl Pts',(-37.3075000008672,4.76023814479221,0.166231178980113));
#29751=CARTESIAN_POINT('Ctrl Pts',(-37.2810416675338,3.49819839664525,2.18591696496197));
#29752=CARTESIAN_POINT('Ctrl Pts',(-37.2545833342005,2.23615864849829,4.20560275094382));
#29753=CARTESIAN_POINT('Ctrl Pts',(-37.2281250008672,-0.143960423897816,
4.12248716145376));
#29754=CARTESIAN_POINT('Ctrl Pts',(-37.2016666675338,-2.52407949629392,
4.03937157196371));
#29755=CARTESIAN_POINT('Ctrl Pts',(-37.1752083342005,-3.64215882054307,
1.9365701964918));
#29756=CARTESIAN_POINT('Ctrl Pts',(-37.1487500008672,-4.76023814479221,
-0.166231178980113));
#29757=CARTESIAN_POINT('Ctrl Pts',(-37.1222916675338,-3.49819839664525,
-2.18591696496196));
#29758=CARTESIAN_POINT('Ctrl Pts',(-37.0958333342005,-2.23615864849829,
-4.20560275094382));
#29759=CARTESIAN_POINT('Ctrl Pts',(-37.0693750008672,0.143960423897816,
-4.12248716145376));
#29760=CARTESIAN_POINT('Ctrl Pts',(-37.0429166675338,2.52407949629392,-4.03937157196371));
#29761=CARTESIAN_POINT('Ctrl Pts',(-37.0164583342005,3.64215882054307,-1.9365701964918));
#29762=CARTESIAN_POINT('Ctrl Pts',(-36.9900000008672,4.76023814479221,0.166231178980113));
#29763=CARTESIAN_POINT('Ctrl Pts',(-36.9635416675338,3.49819839664525,2.18591696496197));
#29764=CARTESIAN_POINT('Ctrl Pts',(-36.9370833342005,2.23615864849829,4.20560275094382));
#29765=CARTESIAN_POINT('Ctrl Pts',(-36.9106250008672,-0.143960423897816,
4.12248716145376));
#29766=CARTESIAN_POINT('Ctrl Pts',(-36.8841666675338,-2.52407949629392,
4.03937157196371));
#29767=CARTESIAN_POINT('Ctrl Pts',(-36.8577083342005,-3.64215882054307,
1.9365701964918));
#29768=CARTESIAN_POINT('Ctrl Pts',(-36.8312500008672,-4.76023814479221,
-0.166231178980113));
#29769=CARTESIAN_POINT('Ctrl Pts',(-36.8047916675338,-3.49819839664525,
-2.18591696496196));
#29770=CARTESIAN_POINT('Ctrl Pts',(-36.7783333342005,-2.23615864849829,
-4.20560275094382));
#29771=CARTESIAN_POINT('Ctrl Pts',(-36.7518750008672,0.143960423897816,
-4.12248716145376));
#29772=CARTESIAN_POINT('Ctrl Pts',(-36.7254166675338,2.52407949629392,-4.03937157196371));
#29773=CARTESIAN_POINT('Ctrl Pts',(-36.6989583342005,3.64215882054307,-1.9365701964918));
#29774=CARTESIAN_POINT('Ctrl Pts',(-36.6725000008672,4.76023814479221,0.166231178980113));
#29775=CARTESIAN_POINT('Ctrl Pts',(-36.6460416675338,3.49819839664525,2.18591696496197));
#29776=CARTESIAN_POINT('Ctrl Pts',(-36.6195833342005,2.23615864849829,4.20560275094382));
#29777=CARTESIAN_POINT('Ctrl Pts',(-36.5931250008672,-0.143960423897816,
4.12248716145376));
#29778=CARTESIAN_POINT('Ctrl Pts',(-36.5666666675338,-2.52407949629392,
4.03937157196371));
#29779=CARTESIAN_POINT('Ctrl Pts',(-36.5402083342005,-3.64215882054307,
1.9365701964918));
#29780=CARTESIAN_POINT('Ctrl Pts',(-36.5137500008672,-4.76023814479221,
-0.166231178980113));
#29781=CARTESIAN_POINT('Ctrl Pts',(-36.4872916675338,-3.49819839664525,
-2.18591696496196));
#29782=CARTESIAN_POINT('Ctrl Pts',(-36.4608333342005,-2.23615864849829,
-4.20560275094382));
#29783=CARTESIAN_POINT('Ctrl Pts',(-36.4343750008672,0.143960423897816,
-4.12248716145376));
#29784=CARTESIAN_POINT('Ctrl Pts',(-36.4079166675338,2.52407949629392,-4.03937157196371));
#29785=CARTESIAN_POINT('Ctrl Pts',(-36.3814583342005,3.64215882054307,-1.9365701964918));
#29786=CARTESIAN_POINT('Ctrl Pts',(-36.3550000008672,4.76023814479221,0.166231178980113));
#29787=CARTESIAN_POINT('Ctrl Pts',(-36.3285416675338,3.49819839664525,2.18591696496197));
#29788=CARTESIAN_POINT('Ctrl Pts',(-36.3020833342005,2.23615864849829,4.20560275094382));
#29789=CARTESIAN_POINT('Ctrl Pts',(-36.2756250008672,-0.143960423897816,
4.12248716145376));
#29790=CARTESIAN_POINT('Ctrl Pts',(-36.2491666675338,-2.52407949629392,
4.03937157196371));
#29791=CARTESIAN_POINT('Ctrl Pts',(-36.2227083342005,-3.64215882054307,
1.9365701964918));
#29792=CARTESIAN_POINT('Ctrl Pts',(-36.1962500008672,-4.76023814479221,
-0.166231178980113));
#29793=CARTESIAN_POINT('Ctrl Pts',(-36.1697916675338,-3.49819839664525,
-2.18591696496196));
#29794=CARTESIAN_POINT('Ctrl Pts',(-36.1433333342005,-2.23615864849829,
-4.20560275094382));
#29795=CARTESIAN_POINT('Ctrl Pts',(-36.1168750008672,0.143960423897816,
-4.12248716145376));
#29796=CARTESIAN_POINT('Ctrl Pts',(-36.0904166675338,2.52407949629392,-4.03937157196371));
#29797=CARTESIAN_POINT('Ctrl Pts',(-36.0639583342005,3.64215882054307,-1.9365701964918));
#29798=CARTESIAN_POINT('Ctrl Pts',(-36.0375000008672,4.76023814479221,0.166231178980113));
#29799=CARTESIAN_POINT('Ctrl Pts',(-36.0110416675338,3.49819839664525,2.18591696496197));
#29800=CARTESIAN_POINT('Ctrl Pts',(-35.9845833342005,2.23615864849829,4.20560275094382));
#29801=CARTESIAN_POINT('Ctrl Pts',(-35.9581250008672,-0.143960423897816,
4.12248716145376));
#29802=CARTESIAN_POINT('Ctrl Pts',(-35.9316666675338,-2.52407949629392,
4.03937157196371));
#29803=CARTESIAN_POINT('Ctrl Pts',(-35.9052083342005,-3.64215882054307,
1.9365701964918));
#29804=CARTESIAN_POINT('Ctrl Pts',(-35.8787500008672,-4.76023814479221,
-0.166231178980113));
#29805=CARTESIAN_POINT('Ctrl Pts',(-35.8522916675338,-3.49819839664525,
-2.18591696496196));
#29806=CARTESIAN_POINT('Ctrl Pts',(-35.8258333342005,-2.23615864849829,
-4.20560275094382));
#29807=CARTESIAN_POINT('Ctrl Pts',(-35.7993750008672,0.143960423897816,
-4.12248716145376));
#29808=CARTESIAN_POINT('Ctrl Pts',(-35.7729166675338,2.52407949629392,-4.03937157196371));
#29809=CARTESIAN_POINT('Ctrl Pts',(-35.7464583342005,3.64215882054307,-1.9365701964918));
#29810=CARTESIAN_POINT('Ctrl Pts',(-35.7200000008672,4.76023814479221,0.166231178980113));
#29811=CARTESIAN_POINT('Ctrl Pts',(-35.6935416675338,3.49819839664525,2.18591696496197));
#29812=CARTESIAN_POINT('Ctrl Pts',(-35.6670833342005,2.23615864849829,4.20560275094382));
#29813=CARTESIAN_POINT('Ctrl Pts',(-35.6406250008672,-0.143960423897816,
4.12248716145376));
#29814=CARTESIAN_POINT('Ctrl Pts',(-35.6141666675338,-2.52407949629392,
4.03937157196371));
#29815=CARTESIAN_POINT('Ctrl Pts',(-35.5877083342005,-3.64215882054307,
1.9365701964918));
#29816=CARTESIAN_POINT('Ctrl Pts',(-35.5612500008672,-4.76023814479221,
-0.166231178980113));
#29817=CARTESIAN_POINT('Ctrl Pts',(-35.5347916675338,-3.49819839664525,
-2.18591696496196));
#29818=CARTESIAN_POINT('Ctrl Pts',(-35.5083333342005,-2.23615864849829,
-4.20560275094382));
#29819=CARTESIAN_POINT('Ctrl Pts',(-35.4818750008672,0.143960423897816,
-4.12248716145376));
#29820=CARTESIAN_POINT('Ctrl Pts',(-35.4554166675338,2.52407949629392,-4.03937157196371));
#29821=CARTESIAN_POINT('Ctrl Pts',(-35.4289583342005,3.64215882054307,-1.9365701964918));
#29822=CARTESIAN_POINT('Ctrl Pts',(-35.4025000008672,4.76023814479221,0.166231178980113));
#29823=CARTESIAN_POINT('Ctrl Pts',(-35.3760416675338,3.49819839664525,2.18591696496197));
#29824=CARTESIAN_POINT('Ctrl Pts',(-35.3495833342005,2.23615864849829,4.20560275094382));
#29825=CARTESIAN_POINT('Ctrl Pts',(-35.3231250008672,-0.143960423897816,
4.12248716145376));
#29826=CARTESIAN_POINT('Ctrl Pts',(-35.2966666675338,-2.52407949629392,
4.03937157196371));
#29827=CARTESIAN_POINT('Ctrl Pts',(-35.2702083342005,-3.64215882054307,
1.9365701964918));
#29828=CARTESIAN_POINT('Ctrl Pts',(-35.2437500008672,-4.76023814479221,
-0.166231178980113));
#29829=CARTESIAN_POINT('Ctrl Pts',(-35.2172916675338,-3.49819839664525,
-2.18591696496196));
#29830=CARTESIAN_POINT('Ctrl Pts',(-35.1908333342005,-2.23615864849829,
-4.20560275094382));
#29831=CARTESIAN_POINT('Ctrl Pts',(-35.1643750008672,0.143960423897816,
-4.12248716145376));
#29832=CARTESIAN_POINT('Ctrl Pts',(-35.1379166675338,2.52407949629392,-4.03937157196371));
#29833=CARTESIAN_POINT('Ctrl Pts',(-35.1114583342005,3.64215882054307,-1.9365701964918));
#29834=CARTESIAN_POINT('Ctrl Pts',(-35.0850000008672,4.76023814479221,0.166231178980113));
#29835=CARTESIAN_POINT('Ctrl Pts',(-35.0585416675338,3.49819839664525,2.18591696496197));
#29836=CARTESIAN_POINT('Ctrl Pts',(-35.0320833342005,2.23615864849829,4.20560275094382));
#29837=CARTESIAN_POINT('Ctrl Pts',(-35.0056250008672,-0.143960423897816,
4.12248716145376));
#29838=CARTESIAN_POINT('Ctrl Pts',(-34.9791666675338,-2.52407949629392,
4.03937157196371));
#29839=CARTESIAN_POINT('Ctrl Pts',(-34.9527083342005,-3.64215882054307,
1.9365701964918));
#29840=CARTESIAN_POINT('Ctrl Pts',(-34.9262500008672,-4.76023814479221,
-0.166231178980113));
#29841=CARTESIAN_POINT('Ctrl Pts',(-34.8997916675338,-3.49819839664525,
-2.18591696496196));
#29842=CARTESIAN_POINT('Ctrl Pts',(-34.8733333342005,-2.23615864849829,
-4.20560275094382));
#29843=CARTESIAN_POINT('Ctrl Pts',(-34.8468750008672,0.143960423897816,
-4.12248716145376));
#29844=CARTESIAN_POINT('Ctrl Pts',(-34.8204166675338,2.52407949629392,-4.03937157196371));
#29845=CARTESIAN_POINT('Ctrl Pts',(-34.7939583342005,3.64215882054307,-1.9365701964918));
#29846=CARTESIAN_POINT('Ctrl Pts',(-34.7675000008672,4.76023814479221,0.166231178980113));
#29847=CARTESIAN_POINT('Ctrl Pts',(-34.7410416675338,3.49819839664525,2.18591696496197));
#29848=CARTESIAN_POINT('Ctrl Pts',(-34.7145833342005,2.23615864849829,4.20560275094382));
#29849=CARTESIAN_POINT('Ctrl Pts',(-34.6881250008672,-0.143960423897816,
4.12248716145376));
#29850=CARTESIAN_POINT('Ctrl Pts',(-34.6616666675338,-2.52407949629392,
4.03937157196371));
#29851=CARTESIAN_POINT('Ctrl Pts',(-34.6352083342005,-3.64215882054307,
1.9365701964918));
#29852=CARTESIAN_POINT('Ctrl Pts',(-34.6087500008672,-4.76023814479221,
-0.166231178980113));
#29853=CARTESIAN_POINT('Ctrl Pts',(-34.5822916675338,-3.49819839664525,
-2.18591696496196));
#29854=CARTESIAN_POINT('Ctrl Pts',(-34.5558333342005,-2.23615864849829,
-4.20560275094382));
#29855=CARTESIAN_POINT('Ctrl Pts',(-34.5293750008672,0.143960423897816,
-4.12248716145376));
#29856=CARTESIAN_POINT('Ctrl Pts',(-34.5029166675338,2.52407949629392,-4.03937157196371));
#29857=CARTESIAN_POINT('Ctrl Pts',(-34.4764583342005,3.64215882054307,-1.9365701964918));
#29858=CARTESIAN_POINT('Ctrl Pts',(-34.4500000008672,4.76023814479221,0.166231178980113));
#29859=CARTESIAN_POINT('Ctrl Pts',(-34.4235416675338,3.49819839664525,2.18591696496197));
#29860=CARTESIAN_POINT('Ctrl Pts',(-34.3970833342005,2.23615864849829,4.20560275094382));
#29861=CARTESIAN_POINT('Ctrl Pts',(-34.3706250008672,-0.143960423897816,
4.12248716145376));
#29862=CARTESIAN_POINT('Ctrl Pts',(-34.3441666675338,-2.52407949629392,
4.03937157196371));
#29863=CARTESIAN_POINT('Ctrl Pts',(-34.3177083342005,-3.64215882054307,
1.9365701964918));
#29864=CARTESIAN_POINT('Ctrl Pts',(-34.2912500008672,-4.76023814479221,
-0.166231178980113));
#29865=CARTESIAN_POINT('Ctrl Pts',(-34.2647916675338,-3.49819839664525,
-2.18591696496196));
#29866=CARTESIAN_POINT('Ctrl Pts',(-34.2383333342005,-2.23615864849829,
-4.20560275094382));
#29867=CARTESIAN_POINT('Ctrl Pts',(-34.2118750008672,0.143960423897816,
-4.12248716145376));
#29868=CARTESIAN_POINT('Ctrl Pts',(-34.1854166675338,2.52407949629392,-4.03937157196371));
#29869=CARTESIAN_POINT('Ctrl Pts',(-34.1589583342005,3.64215882054307,-1.9365701964918));
#29870=CARTESIAN_POINT('Ctrl Pts',(-34.1325000008672,4.76023814479221,0.166231178980113));
#29871=CARTESIAN_POINT('Ctrl Pts',(-34.1060416675338,3.49819839664525,2.18591696496197));
#29872=CARTESIAN_POINT('Ctrl Pts',(-34.0795833342005,2.23615864849829,4.20560275094382));
#29873=CARTESIAN_POINT('Ctrl Pts',(-34.0531250008672,-0.143960423897816,
4.12248716145376));
#29874=CARTESIAN_POINT('Ctrl Pts',(-34.0266666675338,-2.52407949629392,
4.03937157196371));
#29875=CARTESIAN_POINT('Ctrl Pts',(-34.0002083342005,-3.64215882054307,
1.9365701964918));
#29876=CARTESIAN_POINT('Ctrl Pts',(-33.9737500008672,-4.76023814479221,
-0.166231178980113));
#29877=CARTESIAN_POINT('Ctrl Pts',(-33.9472916675338,-3.49819839664525,
-2.18591696496196));
#29878=CARTESIAN_POINT('Ctrl Pts',(-33.9208333342005,-2.23615864849829,
-4.20560275094382));
#29879=CARTESIAN_POINT('Ctrl Pts',(-33.8943750008672,0.143960423897816,
-4.12248716145376));
#29880=CARTESIAN_POINT('Ctrl Pts',(-33.8679166675338,2.52407949629392,-4.03937157196371));
#29881=CARTESIAN_POINT('Ctrl Pts',(-33.8414583342005,3.64215882054307,-1.9365701964918));
#29882=CARTESIAN_POINT('Ctrl Pts',(-33.8150000008672,4.76023814479221,0.166231178980113));
#29883=CARTESIAN_POINT('Ctrl Pts',(-33.7885416675338,3.49819839664525,2.18591696496197));
#29884=CARTESIAN_POINT('Ctrl Pts',(-33.7628337716481,2.27195386943706,4.14831842290086));
#29885=CARTESIAN_POINT('Ctrl Pts',(-33.73676661727,-0.0419478961855304,
4.12478670648623));
#38607=UNCERTAINTY_MEASURE_WITH_UNIT(LENGTH_MEASURE(0.01),#38636,
'DISTANCE_ACCURACY_VALUE',
'Maximum model space distance between geometric entities at asserted c
onnectivities');
#38619=UNCERTAINTY_MEASURE_WITH_UNIT(LENGTH_MEASURE(0.01),#38636,
'DISTANCE_ACCURACY_VALUE',
'Maximum model space distance between geometric entities at asserted c
onnectivities');
#38623=(
GEOMETRIC_REPRESENTATION_CONTEXT(3)
GLOBAL_UNCERTAINTY_ASSIGNED_CONTEXT((#38607))
GLOBAL_UNIT_ASSIGNED_CONTEXT((#38636,#38638,#38639))
REPRESENTATION_CONTEXT('','3D')
);
#38635=(
GEOMETRIC_REPRESENTATION_CONTEXT(3)
GLOBAL_UNCERTAINTY_ASSIGNED_CONTEXT((#38619))
GLOBAL_UNIT_ASSIGNED_CONTEXT((#38636,#38638,#38639))
REPRESENTATION_CONTEXT('','3D')
);
#38636=(
LENGTH_UNIT()
NAMED_UNIT(*)
SI_UNIT(.MILLI.,.METRE.)
);
#38638=(
NAMED_UNIT(*)
PLANE_ANGLE_UNIT()
SI_UNIT($,.RADIAN.)
);
#38639=(
NAMED_UNIT(*)
SI_UNIT($,.STERADIAN.)
SOLID_ANGLE_UNIT()
);
#38643=SHAPE_DEFINITION_REPRESENTATION(#38658,#38687);
#38658=PRODUCT_DEFINITION_SHAPE('',$,#38703);
#38687=SHAPE_REPRESENTATION('',(#17909),#38623);
#38699=PRODUCT_DEFINITION_CONTEXT('part definition',#38746,'design');
#38703=PRODUCT_DEFINITION('Base Cap','Base Cap',#38718,#38699);
#38718=PRODUCT_DEFINITION_FORMATION('',$,#38751);
#38746=APPLICATION_CONTEXT(
'Core Data for Automotive Mechanical Design Process');
#38747=PRODUCT_CONTEXT('part definition',#38746,'mechanical');
#38751=PRODUCT('Base Cap','Base Cap',$,(#38747));
#38766=PRESENTATION_STYLE_ASSIGNMENT((#38773));
#38773=SURFACE_STYLE_USAGE(.BOTH.,#38780);
#38780=SURFACE_SIDE_STYLE('',(#38787));
#38787=SURFACE_STYLE_FILL_AREA(#38794);
#38794=FILL_AREA_STYLE('Opaque(61,176,222)',(#38801));
#38801=FILL_AREA_STYLE_COLOUR('Opaque(61,176,222)',#38808);
#38808=COLOUR_RGB('Opaque(61,176,222)',0.23921568627451,0.690196078431373,
0.870588235294118);
ENDSEC;
END-ISO-10303-21;
